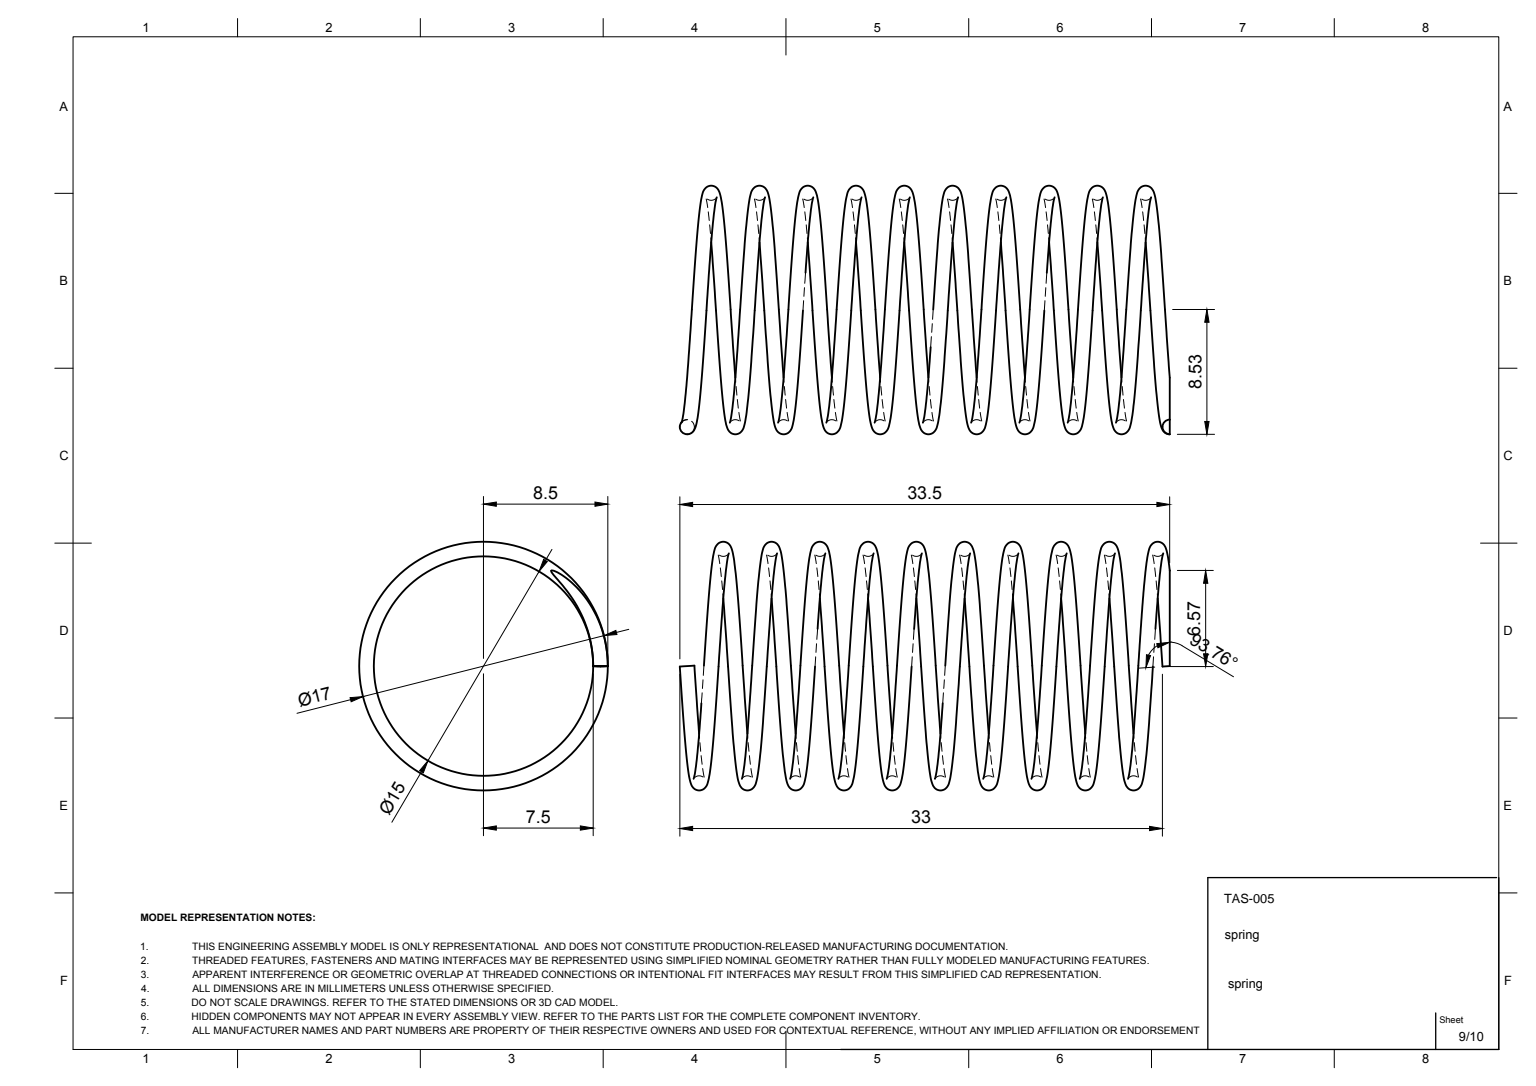
ISO-10303-21;
HEADER;
/* Generated by software containing ST-Developer
 * from STEP Tools, Inc. (www.steptools.com) 
 */

FILE_DESCRIPTION(
/* description */ ('STEP AP214'),
/* implementation_level */ '2;1');

FILE_NAME(
/* name */ 'spring.step',
/* time_stamp */ '2026-11-04T19:54:22-08:00',
/* author */ (''),
/* organization */ (''),
/* preprocessor_version */ 'ST-DEVELOPER v20.2',
/* originating_system */ 'Autodesk Translation Framework v15.17.0.0',
/* authorisation */ '');

FILE_SCHEMA (('AUTOMOTIVE_DESIGN { 1 0 10303 214 3 1 1 }'));
ENDSEC;

DATA;
#10=MECHANICAL_DESIGN_GEOMETRIC_PRESENTATION_REPRESENTATION('',(#245),#14084);
#63=(
BOUNDED_SURFACE()
B_SPLINE_SURFACE(3,2,((#9369,#9370,#9371,#9372,#9373,#9374,#9375,#9376,
#9377,#9378,#9379,#9380,#9381,#9382,#9383,#9384,#9385,#9386,#9387,#9388,
#9389,#9390,#9391,#9392,#9393,#9394,#9395,#9396,#9397,#9398,#9399,#9400,
#9401,#9402,#9403,#9404,#9405,#9406,#9407,#9408,#9409,#9410,#9411,#9412,
#9413,#9414,#9415,#9416,#9417,#9418,#9419,#9420,#9421,#9422,#9423,#9424,
#9425,#9426,#9427,#9428,#9429,#9430,#9431,#9432,#9433,#9434,#9435,#9436,
#9437,#9438,#9439,#9440,#9441,#9442,#9443,#9444,#9445,#9446,#9447,#9448,
#9449,#9450,#9451,#9452,#9453,#9454,#9455,#9456,#9457,#9458,#9459,#9460,
#9461,#9462,#9463,#9464,#9465,#9466,#9467,#9468,#9469,#9470,#9471,#9472,
#9473,#9474,#9475,#9476,#9477,#9478,#9479,#9480,#9481,#9482,#9483,#9484,
#9485,#9486,#9487,#9488,#9489,#9490,#9491,#9492,#9493,#9494,#9495,#9496,
#9497,#9498,#9499,#9500,#9501,#9502,#9503,#9504,#9505,#9506,#9507,#9508,
#9509,#9510,#9511,#9512,#9513,#9514,#9515,#9516,#9517,#9518,#9519,#9520,
#9521,#9522,#9523,#9524,#9525,#9526,#9527,#9528,#9529,#9530,#9531,#9532,
#9533,#9534,#9535,#9536,#9537,#9538,#9539,#9540,#9541,#9542,#9543,#9544,
#9545,#9546,#9547,#9548,#9549,#9550,#9551,#9552,#9553,#9554,#9555,#9556,
#9557,#9558,#9559,#9560,#9561,#9562,#9563,#9564,#9565,#9566,#9567,#9568,
#9569,#9570,#9571,#9572,#9573,#9574,#9575,#9576,#9577,#9578,#9579,#9580,
#9581,#9582,#9583,#9584,#9585,#9586,#9587,#9588,#9589,#9590,#9591,#9592,
#9593,#9594,#9595,#9596,#9597,#9598,#9599,#9600,#9601,#9602,#9603,#9604,
#9605,#9606,#9607,#9608,#9609),(#9610,#9611,#9612,#9613,#9614,#9615,#9616,
#9617,#9618,#9619,#9620,#9621,#9622,#9623,#9624,#9625,#9626,#9627,#9628,
#9629,#9630,#9631,#9632,#9633,#9634,#9635,#9636,#9637,#9638,#9639,#9640,
#9641,#9642,#9643,#9644,#9645,#9646,#9647,#9648,#9649,#9650,#9651,#9652,
#9653,#9654,#9655,#9656,#9657,#9658,#9659,#9660,#9661,#9662,#9663,#9664,
#9665,#9666,#9667,#9668,#9669,#9670,#9671,#9672,#9673,#9674,#9675,#9676,
#9677,#9678,#9679,#9680,#9681,#9682,#9683,#9684,#9685,#9686,#9687,#9688,
#9689,#9690,#9691,#9692,#9693,#9694,#9695,#9696,#9697,#9698,#9699,#9700,
#9701,#9702,#9703,#9704,#9705,#9706,#9707,#9708,#9709,#9710,#9711,#9712,
#9713,#9714,#9715,#9716,#9717,#9718,#9719,#9720,#9721,#9722,#9723,#9724,
#9725,#9726,#9727,#9728,#9729,#9730,#9731,#9732,#9733,#9734,#9735,#9736,
#9737,#9738,#9739,#9740,#9741,#9742,#9743,#9744,#9745,#9746,#9747,#9748,
#9749,#9750,#9751,#9752,#9753,#9754,#9755,#9756,#9757,#9758,#9759,#9760,
#9761,#9762,#9763,#9764,#9765,#9766,#9767,#9768,#9769,#9770,#9771,#9772,
#9773,#9774,#9775,#9776,#9777,#9778,#9779,#9780,#9781,#9782,#9783,#9784,
#9785,#9786,#9787,#9788,#9789,#9790,#9791,#9792,#9793,#9794,#9795,#9796,
#9797,#9798,#9799,#9800,#9801,#9802,#9803,#9804,#9805,#9806,#9807,#9808,
#9809,#9810,#9811,#9812,#9813,#9814,#9815,#9816,#9817,#9818,#9819,#9820,
#9821,#9822,#9823,#9824,#9825,#9826,#9827,#9828,#9829,#9830,#9831,#9832,
#9833,#9834,#9835,#9836,#9837,#9838,#9839,#9840,#9841,#9842,#9843,#9844,
#9845,#9846,#9847,#9848,#9849,#9850),(#9851,#9852,#9853,#9854,#9855,#9856,
#9857,#9858,#9859,#9860,#9861,#9862,#9863,#9864,#9865,#9866,#9867,#9868,
#9869,#9870,#9871,#9872,#9873,#9874,#9875,#9876,#9877,#9878,#9879,#9880,
#9881,#9882,#9883,#9884,#9885,#9886,#9887,#9888,#9889,#9890,#9891,#9892,
#9893,#9894,#9895,#9896,#9897,#9898,#9899,#9900,#9901,#9902,#9903,#9904,
#9905,#9906,#9907,#9908,#9909,#9910,#9911,#9912,#9913,#9914,#9915,#9916,
#9917,#9918,#9919,#9920,#9921,#9922,#9923,#9924,#9925,#9926,#9927,#9928,
#9929,#9930,#9931,#9932,#9933,#9934,#9935,#9936,#9937,#9938,#9939,#9940,
#9941,#9942,#9943,#9944,#9945,#9946,#9947,#9948,#9949,#9950,#9951,#9952,
#9953,#9954,#9955,#9956,#9957,#9958,#9959,#9960,#9961,#9962,#9963,#9964,
#9965,#9966,#9967,#9968,#9969,#9970,#9971,#9972,#9973,#9974,#9975,#9976,
#9977,#9978,#9979,#9980,#9981,#9982,#9983,#9984,#9985,#9986,#9987,#9988,
#9989,#9990,#9991,#9992,#9993,#9994,#9995,#9996,#9997,#9998,#9999,#10000,
#10001,#10002,#10003,#10004,#10005,#10006,#10007,#10008,#10009,#10010,#10011,
#10012,#10013,#10014,#10015,#10016,#10017,#10018,#10019,#10020,#10021,#10022,
#10023,#10024,#10025,#10026,#10027,#10028,#10029,#10030,#10031,#10032,#10033,
#10034,#10035,#10036,#10037,#10038,#10039,#10040,#10041,#10042,#10043,#10044,
#10045,#10046,#10047,#10048,#10049,#10050,#10051,#10052,#10053,#10054,#10055,
#10056,#10057,#10058,#10059,#10060,#10061,#10062,#10063,#10064,#10065,#10066,
#10067,#10068,#10069,#10070,#10071,#10072,#10073,#10074,#10075,#10076,#10077,
#10078,#10079,#10080,#10081,#10082,#10083,#10084,#10085,#10086,#10087,#10088,
#10089,#10090,#10091),(#10092,#10093,#10094,#10095,#10096,#10097,#10098,
#10099,#10100,#10101,#10102,#10103,#10104,#10105,#10106,#10107,#10108,#10109,
#10110,#10111,#10112,#10113,#10114,#10115,#10116,#10117,#10118,#10119,#10120,
#10121,#10122,#10123,#10124,#10125,#10126,#10127,#10128,#10129,#10130,#10131,
#10132,#10133,#10134,#10135,#10136,#10137,#10138,#10139,#10140,#10141,#10142,
#10143,#10144,#10145,#10146,#10147,#10148,#10149,#10150,#10151,#10152,#10153,
#10154,#10155,#10156,#10157,#10158,#10159,#10160,#10161,#10162,#10163,#10164,
#10165,#10166,#10167,#10168,#10169,#10170,#10171,#10172,#10173,#10174,#10175,
#10176,#10177,#10178,#10179,#10180,#10181,#10182,#10183,#10184,#10185,#10186,
#10187,#10188,#10189,#10190,#10191,#10192,#10193,#10194,#10195,#10196,#10197,
#10198,#10199,#10200,#10201,#10202,#10203,#10204,#10205,#10206,#10207,#10208,
#10209,#10210,#10211,#10212,#10213,#10214,#10215,#10216,#10217,#10218,#10219,
#10220,#10221,#10222,#10223,#10224,#10225,#10226,#10227,#10228,#10229,#10230,
#10231,#10232,#10233,#10234,#10235,#10236,#10237,#10238,#10239,#10240,#10241,
#10242,#10243,#10244,#10245,#10246,#10247,#10248,#10249,#10250,#10251,#10252,
#10253,#10254,#10255,#10256,#10257,#10258,#10259,#10260,#10261,#10262,#10263,
#10264,#10265,#10266,#10267,#10268,#10269,#10270,#10271,#10272,#10273,#10274,
#10275,#10276,#10277,#10278,#10279,#10280,#10281,#10282,#10283,#10284,#10285,
#10286,#10287,#10288,#10289,#10290,#10291,#10292,#10293,#10294,#10295,#10296,
#10297,#10298,#10299,#10300,#10301,#10302,#10303,#10304,#10305,#10306,#10307,
#10308,#10309,#10310,#10311,#10312,#10313,#10314,#10315,#10316,#10317,#10318,
#10319,#10320,#10321,#10322,#10323,#10324,#10325,#10326,#10327,#10328,#10329,
#10330,#10331,#10332),(#10333,#10334,#10335,#10336,#10337,#10338,#10339,
#10340,#10341,#10342,#10343,#10344,#10345,#10346,#10347,#10348,#10349,#10350,
#10351,#10352,#10353,#10354,#10355,#10356,#10357,#10358,#10359,#10360,#10361,
#10362,#10363,#10364,#10365,#10366,#10367,#10368,#10369,#10370,#10371,#10372,
#10373,#10374,#10375,#10376,#10377,#10378,#10379,#10380,#10381,#10382,#10383,
#10384,#10385,#10386,#10387,#10388,#10389,#10390,#10391,#10392,#10393,#10394,
#10395,#10396,#10397,#10398,#10399,#10400,#10401,#10402,#10403,#10404,#10405,
#10406,#10407,#10408,#10409,#10410,#10411,#10412,#10413,#10414,#10415,#10416,
#10417,#10418,#10419,#10420,#10421,#10422,#10423,#10424,#10425,#10426,#10427,
#10428,#10429,#10430,#10431,#10432,#10433,#10434,#10435,#10436,#10437,#10438,
#10439,#10440,#10441,#10442,#10443,#10444,#10445,#10446,#10447,#10448,#10449,
#10450,#10451,#10452,#10453,#10454,#10455,#10456,#10457,#10458,#10459,#10460,
#10461,#10462,#10463,#10464,#10465,#10466,#10467,#10468,#10469,#10470,#10471,
#10472,#10473,#10474,#10475,#10476,#10477,#10478,#10479,#10480,#10481,#10482,
#10483,#10484,#10485,#10486,#10487,#10488,#10489,#10490,#10491,#10492,#10493,
#10494,#10495,#10496,#10497,#10498,#10499,#10500,#10501,#10502,#10503,#10504,
#10505,#10506,#10507,#10508,#10509,#10510,#10511,#10512,#10513,#10514,#10515,
#10516,#10517,#10518,#10519,#10520,#10521,#10522,#10523,#10524,#10525,#10526,
#10527,#10528,#10529,#10530,#10531,#10532,#10533,#10534,#10535,#10536,#10537,
#10538,#10539,#10540,#10541,#10542,#10543,#10544,#10545,#10546,#10547,#10548,
#10549,#10550,#10551,#10552,#10553,#10554,#10555,#10556,#10557,#10558,#10559,
#10560,#10561,#10562,#10563,#10564,#10565,#10566,#10567,#10568,#10569,#10570,
#10571,#10572,#10573),(#10574,#10575,#10576,#10577,#10578,#10579,#10580,
#10581,#10582,#10583,#10584,#10585,#10586,#10587,#10588,#10589,#10590,#10591,
#10592,#10593,#10594,#10595,#10596,#10597,#10598,#10599,#10600,#10601,#10602,
#10603,#10604,#10605,#10606,#10607,#10608,#10609,#10610,#10611,#10612,#10613,
#10614,#10615,#10616,#10617,#10618,#10619,#10620,#10621,#10622,#10623,#10624,
#10625,#10626,#10627,#10628,#10629,#10630,#10631,#10632,#10633,#10634,#10635,
#10636,#10637,#10638,#10639,#10640,#10641,#10642,#10643,#10644,#10645,#10646,
#10647,#10648,#10649,#10650,#10651,#10652,#10653,#10654,#10655,#10656,#10657,
#10658,#10659,#10660,#10661,#10662,#10663,#10664,#10665,#10666,#10667,#10668,
#10669,#10670,#10671,#10672,#10673,#10674,#10675,#10676,#10677,#10678,#10679,
#10680,#10681,#10682,#10683,#10684,#10685,#10686,#10687,#10688,#10689,#10690,
#10691,#10692,#10693,#10694,#10695,#10696,#10697,#10698,#10699,#10700,#10701,
#10702,#10703,#10704,#10705,#10706,#10707,#10708,#10709,#10710,#10711,#10712,
#10713,#10714,#10715,#10716,#10717,#10718,#10719,#10720,#10721,#10722,#10723,
#10724,#10725,#10726,#10727,#10728,#10729,#10730,#10731,#10732,#10733,#10734,
#10735,#10736,#10737,#10738,#10739,#10740,#10741,#10742,#10743,#10744,#10745,
#10746,#10747,#10748,#10749,#10750,#10751,#10752,#10753,#10754,#10755,#10756,
#10757,#10758,#10759,#10760,#10761,#10762,#10763,#10764,#10765,#10766,#10767,
#10768,#10769,#10770,#10771,#10772,#10773,#10774,#10775,#10776,#10777,#10778,
#10779,#10780,#10781,#10782,#10783,#10784,#10785,#10786,#10787,#10788,#10789,
#10790,#10791,#10792,#10793,#10794,#10795,#10796,#10797,#10798,#10799,#10800,
#10801,#10802,#10803,#10804,#10805,#10806,#10807,#10808,#10809,#10810,#10811,
#10812,#10813,#10814),(#10815,#10816,#10817,#10818,#10819,#10820,#10821,
#10822,#10823,#10824,#10825,#10826,#10827,#10828,#10829,#10830,#10831,#10832,
#10833,#10834,#10835,#10836,#10837,#10838,#10839,#10840,#10841,#10842,#10843,
#10844,#10845,#10846,#10847,#10848,#10849,#10850,#10851,#10852,#10853,#10854,
#10855,#10856,#10857,#10858,#10859,#10860,#10861,#10862,#10863,#10864,#10865,
#10866,#10867,#10868,#10869,#10870,#10871,#10872,#10873,#10874,#10875,#10876,
#10877,#10878,#10879,#10880,#10881,#10882,#10883,#10884,#10885,#10886,#10887,
#10888,#10889,#10890,#10891,#10892,#10893,#10894,#10895,#10896,#10897,#10898,
#10899,#10900,#10901,#10902,#10903,#10904,#10905,#10906,#10907,#10908,#10909,
#10910,#10911,#10912,#10913,#10914,#10915,#10916,#10917,#10918,#10919,#10920,
#10921,#10922,#10923,#10924,#10925,#10926,#10927,#10928,#10929,#10930,#10931,
#10932,#10933,#10934,#10935,#10936,#10937,#10938,#10939,#10940,#10941,#10942,
#10943,#10944,#10945,#10946,#10947,#10948,#10949,#10950,#10951,#10952,#10953,
#10954,#10955,#10956,#10957,#10958,#10959,#10960,#10961,#10962,#10963,#10964,
#10965,#10966,#10967,#10968,#10969,#10970,#10971,#10972,#10973,#10974,#10975,
#10976,#10977,#10978,#10979,#10980,#10981,#10982,#10983,#10984,#10985,#10986,
#10987,#10988,#10989,#10990,#10991,#10992,#10993,#10994,#10995,#10996,#10997,
#10998,#10999,#11000,#11001,#11002,#11003,#11004,#11005,#11006,#11007,#11008,
#11009,#11010,#11011,#11012,#11013,#11014,#11015,#11016,#11017,#11018,#11019,
#11020,#11021,#11022,#11023,#11024,#11025,#11026,#11027,#11028,#11029,#11030,
#11031,#11032,#11033,#11034,#11035,#11036,#11037,#11038,#11039,#11040,#11041,
#11042,#11043,#11044,#11045,#11046,#11047,#11048,#11049,#11050,#11051,#11052,
#11053,#11054,#11055)),.UNSPECIFIED.,.T.,.F.,.F.)
B_SPLINE_SURFACE_WITH_KNOTS((4,3,4),(3,2,2,2,2,2,2,2,2,2,2,2,2,2,2,2,2,
2,2,2,2,2,2,2,2,2,2,2,2,2,2,2,2,2,2,2,2,2,2,2,2,2,2,2,2,2,2,2,2,2,2,2,2,
2,2,2,2,2,2,2,2,2,2,2,2,2,2,2,2,2,2,2,2,2,2,2,2,2,2,2,2,2,2,2,2,2,2,2,2,
2,2,2,2,2,2,2,2,2,2,2,2,2,2,2,2,2,2,2,2,2,2,2,2,2,2,2,2,2,2,2,3),(0.,0.5,
1.),(0.,0.00833333333333333,0.0166666666666667,0.025,0.0333333333333333,
0.0416666666666667,0.05,0.0583333333333333,0.0666666666666667,0.075,0.0833333333333333,
0.0916666666666667,0.1,0.108333333333333,0.116666666666667,0.125,0.133333333333333,
0.141666666666667,0.15,0.158333333333333,0.166666666666667,0.175,0.183333333333333,
0.191666666666667,0.2,0.208333333333333,0.216666666666667,0.225,0.233333333333333,
0.241666666666667,0.25,0.258333333333333,0.266666666666667,0.275,0.283333333333333,
0.291666666666667,0.3,0.308333333333333,0.316666666666667,0.325,0.333333333333333,
0.341666666666667,0.35,0.358333333333333,0.366666666666667,0.375,0.383333333333333,
0.391666666666667,0.4,0.408333333333333,0.416666666666667,0.425,0.433333333333333,
0.441666666666667,0.45,0.458333333333333,0.466666666666667,0.475,0.483333333333333,
0.491666666666667,0.5,0.508333333333333,0.516666666666667,0.525,0.533333333333333,
0.541666666666667,0.55,0.558333333333333,0.566666666666667,0.575,0.583333333333333,
0.591666666666667,0.6,0.608333333333333,0.616666666666667,0.625,0.633333333333333,
0.641666666666667,0.65,0.658333333333333,0.666666666666667,0.675,0.683333333333333,
0.691666666666667,0.7,0.708333333333333,0.716666666666667,0.725,0.733333333333333,
0.741666666666667,0.75,0.758333333333333,0.766666666666667,0.775,0.783333333333333,
0.791666666666667,0.8,0.808333333333333,0.816666666666667,0.825,0.833333333333333,
0.841666666666667,0.85,0.858333333333333,0.866666666666667,0.875,0.883333333333333,
0.891666666666667,0.9,0.908333333333333,0.916666666666667,0.925,0.933333333333333,
0.941666666666667,0.95,0.958333333333333,0.966666666666667,0.975,0.983333333333333,
0.991666666666667,1.),.UNSPECIFIED.)
GEOMETRIC_REPRESENTATION_ITEM()
RATIONAL_B_SPLINE_SURFACE(((1.,0.965925826289068,1.,0.965925826289068,1.,
0.965925826289068,1.,0.965925826289068,1.,0.965925826289068,1.,0.965925826289068,
1.,0.965925826289068,1.,0.965925826289068,1.,0.965925826289068,1.,0.965925826289068,
1.,0.965925826289068,1.,0.965925826289068,1.,0.965925826289068,1.,0.965925826289068,
1.,0.965925826289068,1.,0.965925826289068,1.,0.965925826289068,1.,0.965925826289068,
1.,0.965925826289068,1.,0.965925826289068,1.,0.965925826289068,1.,0.965925826289068,
1.,0.965925826289068,1.,0.965925826289068,1.,0.965925826289068,1.,0.965925826289068,
1.,0.965925826289068,1.,0.965925826289068,1.,0.965925826289068,1.,0.965925826289068,
1.,0.965925826289068,1.,0.965925826289068,1.,0.965925826289068,1.,0.965925826289068,
1.,0.965925826289068,1.,0.965925826289068,1.,0.965925826289068,1.,0.965925826289068,
1.,0.965925826289068,1.,0.965925826289068,1.,0.965925826289068,1.,0.965925826289068,
1.,0.965925826289068,1.,0.965925826289068,1.,0.965925826289068,1.,0.965925826289068,
1.,0.965925826289068,1.,0.965925826289068,1.,0.965925826289068,1.,0.965925826289068,
1.,0.965925826289068,1.,0.965925826289068,1.,0.965925826289068,1.,0.965925826289068,
1.,0.965925826289068,1.,0.965925826289068,1.,0.965925826289068,1.,0.965925826289068,
1.,0.965925826289068,1.,0.965925826289068,1.,0.965925826289068,1.,0.965925826289068,
1.,0.965925826289068,1.,0.965925826289068,1.,0.965925826289068,1.,0.965925826289068,
1.,0.965925826289068,1.,0.965925826289068,1.,0.965925826289068,1.,0.965925826289068,
1.,0.965925826289068,1.,0.965925826289068,1.,0.965925826289068,1.,0.965925826289068,
1.,0.965925826289068,1.,0.965925826289068,1.,0.965925826289068,1.,0.965925826289068,
1.,0.965925826289068,1.,0.965925826289068,1.,0.965925826289068,1.,0.965925826289068,
1.,0.965925826289068,1.,0.965925826289068,1.,0.965925826289068,1.,0.965925826289068,
1.,0.965925826289068,1.,0.965925826289068,1.,0.965925826289068,1.,0.965925826289068,
1.,0.965925826289068,1.,0.965925826289068,1.,0.965925826289068,1.,0.965925826289068,
1.,0.965925826289068,1.,0.965925826289068,1.,0.965925826289068,1.,0.965925826289068,
1.,0.965925826289068,1.,0.965925826289068,1.,0.965925826289068,1.,0.965925826289068,
1.,0.965925826289068,1.,0.965925826289068,1.,0.965925826289068,1.,0.965925826289068,
1.,0.965925826289068,1.,0.965925826289068,1.,0.965925826289068,1.,0.965925826289068,
1.,0.965925826289068,1.,0.965925826289068,1.,0.965925826289068,1.,0.965925826289068,
1.,0.965925826289068,1.,0.965925826289068,1.,0.965925826289068,1.,0.965925826289068,
1.,0.965925826289068,1.,0.965925826289068,1.),(0.333333333333333,0.321975275429689,
0.333333333333333,0.321975275429689,0.333333333333333,0.321975275429689,
0.333333333333333,0.321975275429689,0.333333333333333,0.321975275429689,
0.333333333333333,0.321975275429689,0.333333333333333,0.321975275429689,
0.333333333333333,0.321975275429689,0.333333333333333,0.321975275429689,
0.333333333333333,0.321975275429689,0.333333333333333,0.321975275429689,
0.333333333333333,0.321975275429689,0.333333333333333,0.321975275429689,
0.333333333333333,0.321975275429689,0.333333333333333,0.321975275429689,
0.333333333333333,0.321975275429689,0.333333333333333,0.321975275429689,
0.333333333333333,0.321975275429689,0.333333333333333,0.321975275429689,
0.333333333333333,0.321975275429689,0.333333333333333,0.321975275429689,
0.333333333333333,0.321975275429689,0.333333333333333,0.321975275429689,
0.333333333333333,0.321975275429689,0.333333333333333,0.321975275429689,
0.333333333333333,0.321975275429689,0.333333333333333,0.321975275429689,
0.333333333333333,0.321975275429689,0.333333333333333,0.321975275429689,
0.333333333333333,0.321975275429689,0.333333333333333,0.321975275429689,
0.333333333333333,0.321975275429689,0.333333333333333,0.321975275429689,
0.333333333333333,0.321975275429689,0.333333333333333,0.321975275429689,
0.333333333333333,0.321975275429689,0.333333333333333,0.321975275429689,
0.333333333333333,0.321975275429689,0.333333333333333,0.321975275429689,
0.333333333333333,0.321975275429689,0.333333333333333,0.321975275429689,
0.333333333333333,0.321975275429689,0.333333333333333,0.321975275429689,
0.333333333333333,0.321975275429689,0.333333333333333,0.321975275429689,
0.333333333333333,0.321975275429689,0.333333333333333,0.321975275429689,
0.333333333333333,0.321975275429689,0.333333333333333,0.321975275429689,
0.333333333333333,0.321975275429689,0.333333333333333,0.321975275429689,
0.333333333333333,0.321975275429689,0.333333333333333,0.321975275429689,
0.333333333333333,0.321975275429689,0.333333333333333,0.321975275429689,
0.333333333333333,0.321975275429689,0.333333333333333,0.321975275429689,
0.333333333333333,0.321975275429689,0.333333333333333,0.321975275429689,
0.333333333333333,0.321975275429689,0.333333333333333,0.321975275429689,
0.333333333333333,0.321975275429689,0.333333333333333,0.321975275429689,
0.333333333333333,0.321975275429689,0.333333333333333,0.321975275429689,
0.333333333333333,0.321975275429689,0.333333333333333,0.321975275429689,
0.333333333333333,0.321975275429689,0.333333333333333,0.321975275429689,
0.333333333333333,0.321975275429689,0.333333333333333,0.321975275429689,
0.333333333333333,0.321975275429689,0.333333333333333,0.321975275429689,
0.333333333333333,0.321975275429689,0.333333333333333,0.321975275429689,
0.333333333333333,0.321975275429689,0.333333333333333,0.321975275429689,
0.333333333333333,0.321975275429689,0.333333333333333,0.321975275429689,
0.333333333333333,0.321975275429689,0.333333333333333,0.321975275429689,
0.333333333333333,0.321975275429689,0.333333333333333,0.321975275429689,
0.333333333333333,0.321975275429689,0.333333333333333,0.321975275429689,
0.333333333333333,0.321975275429689,0.333333333333333,0.321975275429689,
0.333333333333333,0.321975275429689,0.333333333333333,0.321975275429689,
0.333333333333333,0.321975275429689,0.333333333333333,0.321975275429689,
0.333333333333333,0.321975275429689,0.333333333333333,0.321975275429689,
0.333333333333333,0.321975275429689,0.333333333333333,0.321975275429689,
0.333333333333333,0.321975275429689,0.333333333333333,0.321975275429689,
0.333333333333333,0.321975275429689,0.333333333333333,0.321975275429689,
0.333333333333333,0.321975275429689,0.333333333333333,0.321975275429689,
0.333333333333333,0.321975275429689,0.333333333333333,0.321975275429689,
0.333333333333333,0.321975275429689,0.333333333333333,0.321975275429689,
0.333333333333333,0.321975275429689,0.333333333333333,0.321975275429689,
0.333333333333333,0.321975275429689,0.333333333333333,0.321975275429689,
0.333333333333333,0.321975275429689,0.333333333333333,0.321975275429689,
0.333333333333333,0.321975275429689,0.333333333333333,0.321975275429689,
0.333333333333333,0.321975275429689,0.333333333333333,0.321975275429689,
0.333333333333333,0.321975275429689,0.333333333333333,0.321975275429689,
0.333333333333333,0.321975275429689,0.333333333333333,0.321975275429689,
0.333333333333333,0.321975275429689,0.333333333333333),(0.333333333333333,
0.321975275429689,0.333333333333333,0.321975275429689,0.333333333333333,
0.321975275429689,0.333333333333333,0.321975275429689,0.333333333333333,
0.321975275429689,0.333333333333333,0.321975275429689,0.333333333333333,
0.321975275429689,0.333333333333333,0.321975275429689,0.333333333333333,
0.321975275429689,0.333333333333333,0.321975275429689,0.333333333333333,
0.321975275429689,0.333333333333333,0.321975275429689,0.333333333333333,
0.321975275429689,0.333333333333333,0.321975275429689,0.333333333333333,
0.321975275429689,0.333333333333333,0.321975275429689,0.333333333333333,
0.321975275429689,0.333333333333333,0.321975275429689,0.333333333333333,
0.321975275429689,0.333333333333333,0.321975275429689,0.333333333333333,
0.321975275429689,0.333333333333333,0.321975275429689,0.333333333333333,
0.321975275429689,0.333333333333333,0.321975275429689,0.333333333333333,
0.321975275429689,0.333333333333333,0.321975275429689,0.333333333333333,
0.321975275429689,0.333333333333333,0.321975275429689,0.333333333333333,
0.321975275429689,0.333333333333333,0.321975275429689,0.333333333333333,
0.321975275429689,0.333333333333333,0.321975275429689,0.333333333333333,
0.321975275429689,0.333333333333333,0.321975275429689,0.333333333333333,
0.321975275429689,0.333333333333333,0.321975275429689,0.333333333333333,
0.321975275429689,0.333333333333333,0.321975275429689,0.333333333333333,
0.321975275429689,0.333333333333333,0.321975275429689,0.333333333333333,
0.321975275429689,0.333333333333333,0.321975275429689,0.333333333333333,
0.321975275429689,0.333333333333333,0.321975275429689,0.333333333333333,
0.321975275429689,0.333333333333333,0.321975275429689,0.333333333333333,
0.321975275429689,0.333333333333333,0.321975275429689,0.333333333333333,
0.321975275429689,0.333333333333333,0.321975275429689,0.333333333333333,
0.321975275429689,0.333333333333333,0.321975275429689,0.333333333333333,
0.321975275429689,0.333333333333333,0.321975275429689,0.333333333333333,
0.321975275429689,0.333333333333333,0.321975275429689,0.333333333333333,
0.321975275429689,0.333333333333333,0.321975275429689,0.333333333333333,
0.321975275429689,0.333333333333333,0.321975275429689,0.333333333333333,
0.321975275429689,0.333333333333333,0.321975275429689,0.333333333333333,
0.321975275429689,0.333333333333333,0.321975275429689,0.333333333333333,
0.321975275429689,0.333333333333333,0.321975275429689,0.333333333333333,
0.321975275429689,0.333333333333333,0.321975275429689,0.333333333333333,
0.321975275429689,0.333333333333333,0.321975275429689,0.333333333333333,
0.321975275429689,0.333333333333333,0.321975275429689,0.333333333333333,
0.321975275429689,0.333333333333333,0.321975275429689,0.333333333333333,
0.321975275429689,0.333333333333333,0.321975275429689,0.333333333333333,
0.321975275429689,0.333333333333333,0.321975275429689,0.333333333333333,
0.321975275429689,0.333333333333333,0.321975275429689,0.333333333333333,
0.321975275429689,0.333333333333333,0.321975275429689,0.333333333333333,
0.321975275429689,0.333333333333333,0.321975275429689,0.333333333333333,
0.321975275429689,0.333333333333333,0.321975275429689,0.333333333333333,
0.321975275429689,0.333333333333333,0.321975275429689,0.333333333333333,
0.321975275429689,0.333333333333333,0.321975275429689,0.333333333333333,
0.321975275429689,0.333333333333333,0.321975275429689,0.333333333333333,
0.321975275429689,0.333333333333333,0.321975275429689,0.333333333333333,
0.321975275429689,0.333333333333333,0.321975275429689,0.333333333333333,
0.321975275429689,0.333333333333333,0.321975275429689,0.333333333333333,
0.321975275429689,0.333333333333333,0.321975275429689,0.333333333333333,
0.321975275429689,0.333333333333333,0.321975275429689,0.333333333333333,
0.321975275429689,0.333333333333333,0.321975275429689,0.333333333333333,
0.321975275429689,0.333333333333333,0.321975275429689,0.333333333333333,
0.321975275429689,0.333333333333333,0.321975275429689,0.333333333333333,
0.321975275429689,0.333333333333333,0.321975275429689,0.333333333333333,
0.321975275429689,0.333333333333333,0.321975275429689,0.333333333333333,
0.321975275429689,0.333333333333333,0.321975275429689,0.333333333333333,
0.321975275429689,0.333333333333333,0.321975275429689,0.333333333333333,
0.321975275429689,0.333333333333333,0.321975275429689,0.333333333333333,
0.321975275429689,0.333333333333333,0.321975275429689,0.333333333333333),
(1.,0.965925826289068,1.,0.965925826289068,1.,0.965925826289068,1.,0.965925826289068,
1.,0.965925826289068,1.,0.965925826289068,1.,0.965925826289068,1.,0.965925826289068,
1.,0.965925826289068,1.,0.965925826289068,1.,0.965925826289068,1.,0.965925826289068,
1.,0.965925826289068,1.,0.965925826289068,1.,0.965925826289068,1.,0.965925826289068,
1.,0.965925826289068,1.,0.965925826289068,1.,0.965925826289068,1.,0.965925826289068,
1.,0.965925826289068,1.,0.965925826289068,1.,0.965925826289068,1.,0.965925826289068,
1.,0.965925826289068,1.,0.965925826289068,1.,0.965925826289068,1.,0.965925826289068,
1.,0.965925826289068,1.,0.965925826289068,1.,0.965925826289068,1.,0.965925826289068,
1.,0.965925826289068,1.,0.965925826289068,1.,0.965925826289068,1.,0.965925826289068,
1.,0.965925826289068,1.,0.965925826289068,1.,0.965925826289068,1.,0.965925826289068,
1.,0.965925826289068,1.,0.965925826289068,1.,0.965925826289068,1.,0.965925826289068,
1.,0.965925826289068,1.,0.965925826289068,1.,0.965925826289068,1.,0.965925826289068,
1.,0.965925826289068,1.,0.965925826289068,1.,0.965925826289068,1.,0.965925826289068,
1.,0.965925826289068,1.,0.965925826289068,1.,0.965925826289068,1.,0.965925826289068,
1.,0.965925826289068,1.,0.965925826289068,1.,0.965925826289068,1.,0.965925826289068,
1.,0.965925826289068,1.,0.965925826289068,1.,0.965925826289068,1.,0.965925826289068,
1.,0.965925826289068,1.,0.965925826289068,1.,0.965925826289068,1.,0.965925826289068,
1.,0.965925826289068,1.,0.965925826289068,1.,0.965925826289068,1.,0.965925826289068,
1.,0.965925826289068,1.,0.965925826289068,1.,0.965925826289068,1.,0.965925826289068,
1.,0.965925826289068,1.,0.965925826289068,1.,0.965925826289068,1.,0.965925826289068,
1.,0.965925826289068,1.,0.965925826289068,1.,0.965925826289068,1.,0.965925826289068,
1.,0.965925826289068,1.,0.965925826289068,1.,0.965925826289068,1.,0.965925826289068,
1.,0.965925826289068,1.,0.965925826289068,1.,0.965925826289068,1.,0.965925826289068,
1.,0.965925826289068,1.,0.965925826289068,1.,0.965925826289068,1.,0.965925826289068,
1.,0.965925826289068,1.,0.965925826289068,1.,0.965925826289068,1.,0.965925826289068,
1.,0.965925826289068,1.,0.965925826289068,1.,0.965925826289068,1.,0.965925826289068,
1.,0.965925826289068,1.,0.965925826289068,1.,0.965925826289068,1.,0.965925826289068,
1.,0.965925826289068,1.,0.965925826289068,1.,0.965925826289068,1.,0.965925826289068,
1.,0.965925826289068,1.,0.965925826289068,1.,0.965925826289068,1.,0.965925826289068,
1.,0.965925826289068,1.,0.965925826289068,1.,0.965925826289068,1.,0.965925826289068,
1.),(0.333333333333333,0.321975275429689,0.333333333333333,0.321975275429689,
0.333333333333333,0.321975275429689,0.333333333333333,0.321975275429689,
0.333333333333333,0.321975275429689,0.333333333333333,0.321975275429689,
0.333333333333333,0.321975275429689,0.333333333333333,0.321975275429689,
0.333333333333333,0.321975275429689,0.333333333333333,0.321975275429689,
0.333333333333333,0.321975275429689,0.333333333333333,0.321975275429689,
0.333333333333333,0.321975275429689,0.333333333333333,0.321975275429689,
0.333333333333333,0.321975275429689,0.333333333333333,0.321975275429689,
0.333333333333333,0.321975275429689,0.333333333333333,0.321975275429689,
0.333333333333333,0.321975275429689,0.333333333333333,0.321975275429689,
0.333333333333333,0.321975275429689,0.333333333333333,0.321975275429689,
0.333333333333333,0.321975275429689,0.333333333333333,0.321975275429689,
0.333333333333333,0.321975275429689,0.333333333333333,0.321975275429689,
0.333333333333333,0.321975275429689,0.333333333333333,0.321975275429689,
0.333333333333333,0.321975275429689,0.333333333333333,0.321975275429689,
0.333333333333333,0.321975275429689,0.333333333333333,0.321975275429689,
0.333333333333333,0.321975275429689,0.333333333333333,0.321975275429689,
0.333333333333333,0.321975275429689,0.333333333333333,0.321975275429689,
0.333333333333333,0.321975275429689,0.333333333333333,0.321975275429689,
0.333333333333333,0.321975275429689,0.333333333333333,0.321975275429689,
0.333333333333333,0.321975275429689,0.333333333333333,0.321975275429689,
0.333333333333333,0.321975275429689,0.333333333333333,0.321975275429689,
0.333333333333333,0.321975275429689,0.333333333333333,0.321975275429689,
0.333333333333333,0.321975275429689,0.333333333333333,0.321975275429689,
0.333333333333333,0.321975275429689,0.333333333333333,0.321975275429689,
0.333333333333333,0.321975275429689,0.333333333333333,0.321975275429689,
0.333333333333333,0.321975275429689,0.333333333333333,0.321975275429689,
0.333333333333333,0.321975275429689,0.333333333333333,0.321975275429689,
0.333333333333333,0.321975275429689,0.333333333333333,0.321975275429689,
0.333333333333333,0.321975275429689,0.333333333333333,0.321975275429689,
0.333333333333333,0.321975275429689,0.333333333333333,0.321975275429689,
0.333333333333333,0.321975275429689,0.333333333333333,0.321975275429689,
0.333333333333333,0.321975275429689,0.333333333333333,0.321975275429689,
0.333333333333333,0.321975275429689,0.333333333333333,0.321975275429689,
0.333333333333333,0.321975275429689,0.333333333333333,0.321975275429689,
0.333333333333333,0.321975275429689,0.333333333333333,0.321975275429689,
0.333333333333333,0.321975275429689,0.333333333333333,0.321975275429689,
0.333333333333333,0.321975275429689,0.333333333333333,0.321975275429689,
0.333333333333333,0.321975275429689,0.333333333333333,0.321975275429689,
0.333333333333333,0.321975275429689,0.333333333333333,0.321975275429689,
0.333333333333333,0.321975275429689,0.333333333333333,0.321975275429689,
0.333333333333333,0.321975275429689,0.333333333333333,0.321975275429689,
0.333333333333333,0.321975275429689,0.333333333333333,0.321975275429689,
0.333333333333333,0.321975275429689,0.333333333333333,0.321975275429689,
0.333333333333333,0.321975275429689,0.333333333333333,0.321975275429689,
0.333333333333333,0.321975275429689,0.333333333333333,0.321975275429689,
0.333333333333333,0.321975275429689,0.333333333333333,0.321975275429689,
0.333333333333333,0.321975275429689,0.333333333333333,0.321975275429689,
0.333333333333333,0.321975275429689,0.333333333333333,0.321975275429689,
0.333333333333333,0.321975275429689,0.333333333333333,0.321975275429689,
0.333333333333333,0.321975275429689,0.333333333333333,0.321975275429689,
0.333333333333333,0.321975275429689,0.333333333333333,0.321975275429689,
0.333333333333333,0.321975275429689,0.333333333333333,0.321975275429689,
0.333333333333333,0.321975275429689,0.333333333333333,0.321975275429689,
0.333333333333333,0.321975275429689,0.333333333333333,0.321975275429689,
0.333333333333333,0.321975275429689,0.333333333333333,0.321975275429689,
0.333333333333333,0.321975275429689,0.333333333333333,0.321975275429689,
0.333333333333333,0.321975275429689,0.333333333333333,0.321975275429689,
0.333333333333333,0.321975275429689,0.333333333333333,0.321975275429689,
0.333333333333333,0.321975275429689,0.333333333333333,0.321975275429689,
0.333333333333333),(0.333333333333333,0.321975275429689,0.333333333333333,
0.321975275429689,0.333333333333333,0.321975275429689,0.333333333333333,
0.321975275429689,0.333333333333333,0.321975275429689,0.333333333333333,
0.321975275429689,0.333333333333333,0.321975275429689,0.333333333333333,
0.321975275429689,0.333333333333333,0.321975275429689,0.333333333333333,
0.321975275429689,0.333333333333333,0.321975275429689,0.333333333333333,
0.321975275429689,0.333333333333333,0.321975275429689,0.333333333333333,
0.321975275429689,0.333333333333333,0.321975275429689,0.333333333333333,
0.321975275429689,0.333333333333333,0.321975275429689,0.333333333333333,
0.321975275429689,0.333333333333333,0.321975275429689,0.333333333333333,
0.321975275429689,0.333333333333333,0.321975275429689,0.333333333333333,
0.321975275429689,0.333333333333333,0.321975275429689,0.333333333333333,
0.321975275429689,0.333333333333333,0.321975275429689,0.333333333333333,
0.321975275429689,0.333333333333333,0.321975275429689,0.333333333333333,
0.321975275429689,0.333333333333333,0.321975275429689,0.333333333333333,
0.321975275429689,0.333333333333333,0.321975275429689,0.333333333333333,
0.321975275429689,0.333333333333333,0.321975275429689,0.333333333333333,
0.321975275429689,0.333333333333333,0.321975275429689,0.333333333333333,
0.321975275429689,0.333333333333333,0.321975275429689,0.333333333333333,
0.321975275429689,0.333333333333333,0.321975275429689,0.333333333333333,
0.321975275429689,0.333333333333333,0.321975275429689,0.333333333333333,
0.321975275429689,0.333333333333333,0.321975275429689,0.333333333333333,
0.321975275429689,0.333333333333333,0.321975275429689,0.333333333333333,
0.321975275429689,0.333333333333333,0.321975275429689,0.333333333333333,
0.321975275429689,0.333333333333333,0.321975275429689,0.333333333333333,
0.321975275429689,0.333333333333333,0.321975275429689,0.333333333333333,
0.321975275429689,0.333333333333333,0.321975275429689,0.333333333333333,
0.321975275429689,0.333333333333333,0.321975275429689,0.333333333333333,
0.321975275429689,0.333333333333333,0.321975275429689,0.333333333333333,
0.321975275429689,0.333333333333333,0.321975275429689,0.333333333333333,
0.321975275429689,0.333333333333333,0.321975275429689,0.333333333333333,
0.321975275429689,0.333333333333333,0.321975275429689,0.333333333333333,
0.321975275429689,0.333333333333333,0.321975275429689,0.333333333333333,
0.321975275429689,0.333333333333333,0.321975275429689,0.333333333333333,
0.321975275429689,0.333333333333333,0.321975275429689,0.333333333333333,
0.321975275429689,0.333333333333333,0.321975275429689,0.333333333333333,
0.321975275429689,0.333333333333333,0.321975275429689,0.333333333333333,
0.321975275429689,0.333333333333333,0.321975275429689,0.333333333333333,
0.321975275429689,0.333333333333333,0.321975275429689,0.333333333333333,
0.321975275429689,0.333333333333333,0.321975275429689,0.333333333333333,
0.321975275429689,0.333333333333333,0.321975275429689,0.333333333333333,
0.321975275429689,0.333333333333333,0.321975275429689,0.333333333333333,
0.321975275429689,0.333333333333333,0.321975275429689,0.333333333333333,
0.321975275429689,0.333333333333333,0.321975275429689,0.333333333333333,
0.321975275429689,0.333333333333333,0.321975275429689,0.333333333333333,
0.321975275429689,0.333333333333333,0.321975275429689,0.333333333333333,
0.321975275429689,0.333333333333333,0.321975275429689,0.333333333333333,
0.321975275429689,0.333333333333333,0.321975275429689,0.333333333333333,
0.321975275429689,0.333333333333333,0.321975275429689,0.333333333333333,
0.321975275429689,0.333333333333333,0.321975275429689,0.333333333333333,
0.321975275429689,0.333333333333333,0.321975275429689,0.333333333333333,
0.321975275429689,0.333333333333333,0.321975275429689,0.333333333333333,
0.321975275429689,0.333333333333333,0.321975275429689,0.333333333333333,
0.321975275429689,0.333333333333333,0.321975275429689,0.333333333333333,
0.321975275429689,0.333333333333333,0.321975275429689,0.333333333333333,
0.321975275429689,0.333333333333333,0.321975275429689,0.333333333333333,
0.321975275429689,0.333333333333333,0.321975275429689,0.333333333333333,
0.321975275429689,0.333333333333333,0.321975275429689,0.333333333333333,
0.321975275429689,0.333333333333333,0.321975275429689,0.333333333333333,
0.321975275429689,0.333333333333333,0.321975275429689,0.333333333333333,
0.321975275429689,0.333333333333333),(1.,0.965925826289068,1.,0.965925826289068,
1.,0.965925826289068,1.,0.965925826289068,1.,0.965925826289068,1.,0.965925826289068,
1.,0.965925826289068,1.,0.965925826289068,1.,0.965925826289068,1.,0.965925826289068,
1.,0.965925826289068,1.,0.965925826289068,1.,0.965925826289068,1.,0.965925826289068,
1.,0.965925826289068,1.,0.965925826289068,1.,0.965925826289068,1.,0.965925826289068,
1.,0.965925826289068,1.,0.965925826289068,1.,0.965925826289068,1.,0.965925826289068,
1.,0.965925826289068,1.,0.965925826289068,1.,0.965925826289068,1.,0.965925826289068,
1.,0.965925826289068,1.,0.965925826289068,1.,0.965925826289068,1.,0.965925826289068,
1.,0.965925826289068,1.,0.965925826289068,1.,0.965925826289068,1.,0.965925826289068,
1.,0.965925826289068,1.,0.965925826289068,1.,0.965925826289068,1.,0.965925826289068,
1.,0.965925826289068,1.,0.965925826289068,1.,0.965925826289068,1.,0.965925826289068,
1.,0.965925826289068,1.,0.965925826289068,1.,0.965925826289068,1.,0.965925826289068,
1.,0.965925826289068,1.,0.965925826289068,1.,0.965925826289068,1.,0.965925826289068,
1.,0.965925826289068,1.,0.965925826289068,1.,0.965925826289068,1.,0.965925826289068,
1.,0.965925826289068,1.,0.965925826289068,1.,0.965925826289068,1.,0.965925826289068,
1.,0.965925826289068,1.,0.965925826289068,1.,0.965925826289068,1.,0.965925826289068,
1.,0.965925826289068,1.,0.965925826289068,1.,0.965925826289068,1.,0.965925826289068,
1.,0.965925826289068,1.,0.965925826289068,1.,0.965925826289068,1.,0.965925826289068,
1.,0.965925826289068,1.,0.965925826289068,1.,0.965925826289068,1.,0.965925826289068,
1.,0.965925826289068,1.,0.965925826289068,1.,0.965925826289068,1.,0.965925826289068,
1.,0.965925826289068,1.,0.965925826289068,1.,0.965925826289068,1.,0.965925826289068,
1.,0.965925826289068,1.,0.965925826289068,1.,0.965925826289068,1.,0.965925826289068,
1.,0.965925826289068,1.,0.965925826289068,1.,0.965925826289068,1.,0.965925826289068,
1.,0.965925826289068,1.,0.965925826289068,1.,0.965925826289068,1.,0.965925826289068,
1.,0.965925826289068,1.,0.965925826289068,1.,0.965925826289068,1.,0.965925826289068,
1.,0.965925826289068,1.,0.965925826289068,1.,0.965925826289068,1.,0.965925826289068,
1.,0.965925826289068,1.,0.965925826289068,1.,0.965925826289068,1.,0.965925826289068,
1.,0.965925826289068,1.,0.965925826289068,1.,0.965925826289068,1.,0.965925826289068,
1.,0.965925826289068,1.,0.965925826289068,1.,0.965925826289068,1.,0.965925826289068,
1.,0.965925826289068,1.,0.965925826289068,1.,0.965925826289068,1.,0.965925826289068,
1.,0.965925826289068,1.,0.965925826289068,1.)))
REPRESENTATION_ITEM('')
SURFACE()
);
#64=(
BOUNDED_SURFACE()
B_SPLINE_SURFACE(3,2,((#11567,#11568,#11569,#11570,#11571,#11572,#11573,
#11574,#11575,#11576,#11577,#11578,#11579,#11580,#11581,#11582,#11583,#11584,
#11585,#11586,#11587,#11588,#11589,#11590,#11591,#11592,#11593,#11594,#11595,
#11596,#11597,#11598,#11599,#11600,#11601,#11602,#11603,#11604,#11605,#11606,
#11607,#11608,#11609,#11610,#11611,#11612,#11613,#11614,#11615,#11616,#11617,
#11618,#11619,#11620,#11621,#11622,#11623,#11624,#11625,#11626,#11627,#11628,
#11629,#11630,#11631,#11632,#11633,#11634,#11635,#11636,#11637,#11638,#11639,
#11640,#11641,#11642,#11643,#11644,#11645,#11646,#11647,#11648,#11649,#11650,
#11651,#11652,#11653,#11654,#11655,#11656,#11657,#11658,#11659,#11660,#11661,
#11662,#11663,#11664,#11665,#11666,#11667,#11668,#11669,#11670,#11671,#11672,
#11673,#11674,#11675,#11676,#11677,#11678,#11679,#11680,#11681,#11682,#11683,
#11684,#11685,#11686,#11687,#11688,#11689,#11690,#11691,#11692,#11693,#11694,
#11695,#11696,#11697,#11698,#11699,#11700,#11701,#11702,#11703,#11704,#11705,
#11706,#11707,#11708,#11709,#11710,#11711,#11712,#11713,#11714,#11715,#11716,
#11717,#11718,#11719,#11720,#11721,#11722,#11723,#11724,#11725,#11726,#11727,
#11728,#11729,#11730,#11731,#11732,#11733,#11734,#11735,#11736,#11737,#11738,
#11739,#11740,#11741,#11742,#11743,#11744,#11745,#11746,#11747,#11748,#11749,
#11750,#11751,#11752,#11753,#11754,#11755,#11756,#11757,#11758,#11759,#11760,
#11761,#11762,#11763,#11764,#11765,#11766,#11767,#11768,#11769,#11770,#11771,
#11772,#11773,#11774,#11775,#11776,#11777,#11778,#11779,#11780,#11781,#11782,
#11783,#11784,#11785,#11786,#11787,#11788,#11789,#11790,#11791,#11792,#11793,
#11794,#11795,#11796,#11797,#11798,#11799,#11800,#11801,#11802,#11803,#11804,
#11805,#11806,#11807),(#11808,#11809,#11810,#11811,#11812,#11813,#11814,
#11815,#11816,#11817,#11818,#11819,#11820,#11821,#11822,#11823,#11824,#11825,
#11826,#11827,#11828,#11829,#11830,#11831,#11832,#11833,#11834,#11835,#11836,
#11837,#11838,#11839,#11840,#11841,#11842,#11843,#11844,#11845,#11846,#11847,
#11848,#11849,#11850,#11851,#11852,#11853,#11854,#11855,#11856,#11857,#11858,
#11859,#11860,#11861,#11862,#11863,#11864,#11865,#11866,#11867,#11868,#11869,
#11870,#11871,#11872,#11873,#11874,#11875,#11876,#11877,#11878,#11879,#11880,
#11881,#11882,#11883,#11884,#11885,#11886,#11887,#11888,#11889,#11890,#11891,
#11892,#11893,#11894,#11895,#11896,#11897,#11898,#11899,#11900,#11901,#11902,
#11903,#11904,#11905,#11906,#11907,#11908,#11909,#11910,#11911,#11912,#11913,
#11914,#11915,#11916,#11917,#11918,#11919,#11920,#11921,#11922,#11923,#11924,
#11925,#11926,#11927,#11928,#11929,#11930,#11931,#11932,#11933,#11934,#11935,
#11936,#11937,#11938,#11939,#11940,#11941,#11942,#11943,#11944,#11945,#11946,
#11947,#11948,#11949,#11950,#11951,#11952,#11953,#11954,#11955,#11956,#11957,
#11958,#11959,#11960,#11961,#11962,#11963,#11964,#11965,#11966,#11967,#11968,
#11969,#11970,#11971,#11972,#11973,#11974,#11975,#11976,#11977,#11978,#11979,
#11980,#11981,#11982,#11983,#11984,#11985,#11986,#11987,#11988,#11989,#11990,
#11991,#11992,#11993,#11994,#11995,#11996,#11997,#11998,#11999,#12000,#12001,
#12002,#12003,#12004,#12005,#12006,#12007,#12008,#12009,#12010,#12011,#12012,
#12013,#12014,#12015,#12016,#12017,#12018,#12019,#12020,#12021,#12022,#12023,
#12024,#12025,#12026,#12027,#12028,#12029,#12030,#12031,#12032,#12033,#12034,
#12035,#12036,#12037,#12038,#12039,#12040,#12041,#12042,#12043,#12044,#12045,
#12046,#12047,#12048),(#12049,#12050,#12051,#12052,#12053,#12054,#12055,
#12056,#12057,#12058,#12059,#12060,#12061,#12062,#12063,#12064,#12065,#12066,
#12067,#12068,#12069,#12070,#12071,#12072,#12073,#12074,#12075,#12076,#12077,
#12078,#12079,#12080,#12081,#12082,#12083,#12084,#12085,#12086,#12087,#12088,
#12089,#12090,#12091,#12092,#12093,#12094,#12095,#12096,#12097,#12098,#12099,
#12100,#12101,#12102,#12103,#12104,#12105,#12106,#12107,#12108,#12109,#12110,
#12111,#12112,#12113,#12114,#12115,#12116,#12117,#12118,#12119,#12120,#12121,
#12122,#12123,#12124,#12125,#12126,#12127,#12128,#12129,#12130,#12131,#12132,
#12133,#12134,#12135,#12136,#12137,#12138,#12139,#12140,#12141,#12142,#12143,
#12144,#12145,#12146,#12147,#12148,#12149,#12150,#12151,#12152,#12153,#12154,
#12155,#12156,#12157,#12158,#12159,#12160,#12161,#12162,#12163,#12164,#12165,
#12166,#12167,#12168,#12169,#12170,#12171,#12172,#12173,#12174,#12175,#12176,
#12177,#12178,#12179,#12180,#12181,#12182,#12183,#12184,#12185,#12186,#12187,
#12188,#12189,#12190,#12191,#12192,#12193,#12194,#12195,#12196,#12197,#12198,
#12199,#12200,#12201,#12202,#12203,#12204,#12205,#12206,#12207,#12208,#12209,
#12210,#12211,#12212,#12213,#12214,#12215,#12216,#12217,#12218,#12219,#12220,
#12221,#12222,#12223,#12224,#12225,#12226,#12227,#12228,#12229,#12230,#12231,
#12232,#12233,#12234,#12235,#12236,#12237,#12238,#12239,#12240,#12241,#12242,
#12243,#12244,#12245,#12246,#12247,#12248,#12249,#12250,#12251,#12252,#12253,
#12254,#12255,#12256,#12257,#12258,#12259,#12260,#12261,#12262,#12263,#12264,
#12265,#12266,#12267,#12268,#12269,#12270,#12271,#12272,#12273,#12274,#12275,
#12276,#12277,#12278,#12279,#12280,#12281,#12282,#12283,#12284,#12285,#12286,
#12287,#12288,#12289),(#12290,#12291,#12292,#12293,#12294,#12295,#12296,
#12297,#12298,#12299,#12300,#12301,#12302,#12303,#12304,#12305,#12306,#12307,
#12308,#12309,#12310,#12311,#12312,#12313,#12314,#12315,#12316,#12317,#12318,
#12319,#12320,#12321,#12322,#12323,#12324,#12325,#12326,#12327,#12328,#12329,
#12330,#12331,#12332,#12333,#12334,#12335,#12336,#12337,#12338,#12339,#12340,
#12341,#12342,#12343,#12344,#12345,#12346,#12347,#12348,#12349,#12350,#12351,
#12352,#12353,#12354,#12355,#12356,#12357,#12358,#12359,#12360,#12361,#12362,
#12363,#12364,#12365,#12366,#12367,#12368,#12369,#12370,#12371,#12372,#12373,
#12374,#12375,#12376,#12377,#12378,#12379,#12380,#12381,#12382,#12383,#12384,
#12385,#12386,#12387,#12388,#12389,#12390,#12391,#12392,#12393,#12394,#12395,
#12396,#12397,#12398,#12399,#12400,#12401,#12402,#12403,#12404,#12405,#12406,
#12407,#12408,#12409,#12410,#12411,#12412,#12413,#12414,#12415,#12416,#12417,
#12418,#12419,#12420,#12421,#12422,#12423,#12424,#12425,#12426,#12427,#12428,
#12429,#12430,#12431,#12432,#12433,#12434,#12435,#12436,#12437,#12438,#12439,
#12440,#12441,#12442,#12443,#12444,#12445,#12446,#12447,#12448,#12449,#12450,
#12451,#12452,#12453,#12454,#12455,#12456,#12457,#12458,#12459,#12460,#12461,
#12462,#12463,#12464,#12465,#12466,#12467,#12468,#12469,#12470,#12471,#12472,
#12473,#12474,#12475,#12476,#12477,#12478,#12479,#12480,#12481,#12482,#12483,
#12484,#12485,#12486,#12487,#12488,#12489,#12490,#12491,#12492,#12493,#12494,
#12495,#12496,#12497,#12498,#12499,#12500,#12501,#12502,#12503,#12504,#12505,
#12506,#12507,#12508,#12509,#12510,#12511,#12512,#12513,#12514,#12515,#12516,
#12517,#12518,#12519,#12520,#12521,#12522,#12523,#12524,#12525,#12526,#12527,
#12528,#12529,#12530),(#12531,#12532,#12533,#12534,#12535,#12536,#12537,
#12538,#12539,#12540,#12541,#12542,#12543,#12544,#12545,#12546,#12547,#12548,
#12549,#12550,#12551,#12552,#12553,#12554,#12555,#12556,#12557,#12558,#12559,
#12560,#12561,#12562,#12563,#12564,#12565,#12566,#12567,#12568,#12569,#12570,
#12571,#12572,#12573,#12574,#12575,#12576,#12577,#12578,#12579,#12580,#12581,
#12582,#12583,#12584,#12585,#12586,#12587,#12588,#12589,#12590,#12591,#12592,
#12593,#12594,#12595,#12596,#12597,#12598,#12599,#12600,#12601,#12602,#12603,
#12604,#12605,#12606,#12607,#12608,#12609,#12610,#12611,#12612,#12613,#12614,
#12615,#12616,#12617,#12618,#12619,#12620,#12621,#12622,#12623,#12624,#12625,
#12626,#12627,#12628,#12629,#12630,#12631,#12632,#12633,#12634,#12635,#12636,
#12637,#12638,#12639,#12640,#12641,#12642,#12643,#12644,#12645,#12646,#12647,
#12648,#12649,#12650,#12651,#12652,#12653,#12654,#12655,#12656,#12657,#12658,
#12659,#12660,#12661,#12662,#12663,#12664,#12665,#12666,#12667,#12668,#12669,
#12670,#12671,#12672,#12673,#12674,#12675,#12676,#12677,#12678,#12679,#12680,
#12681,#12682,#12683,#12684,#12685,#12686,#12687,#12688,#12689,#12690,#12691,
#12692,#12693,#12694,#12695,#12696,#12697,#12698,#12699,#12700,#12701,#12702,
#12703,#12704,#12705,#12706,#12707,#12708,#12709,#12710,#12711,#12712,#12713,
#12714,#12715,#12716,#12717,#12718,#12719,#12720,#12721,#12722,#12723,#12724,
#12725,#12726,#12727,#12728,#12729,#12730,#12731,#12732,#12733,#12734,#12735,
#12736,#12737,#12738,#12739,#12740,#12741,#12742,#12743,#12744,#12745,#12746,
#12747,#12748,#12749,#12750,#12751,#12752,#12753,#12754,#12755,#12756,#12757,
#12758,#12759,#12760,#12761,#12762,#12763,#12764,#12765,#12766,#12767,#12768,
#12769,#12770,#12771),(#12772,#12773,#12774,#12775,#12776,#12777,#12778,
#12779,#12780,#12781,#12782,#12783,#12784,#12785,#12786,#12787,#12788,#12789,
#12790,#12791,#12792,#12793,#12794,#12795,#12796,#12797,#12798,#12799,#12800,
#12801,#12802,#12803,#12804,#12805,#12806,#12807,#12808,#12809,#12810,#12811,
#12812,#12813,#12814,#12815,#12816,#12817,#12818,#12819,#12820,#12821,#12822,
#12823,#12824,#12825,#12826,#12827,#12828,#12829,#12830,#12831,#12832,#12833,
#12834,#12835,#12836,#12837,#12838,#12839,#12840,#12841,#12842,#12843,#12844,
#12845,#12846,#12847,#12848,#12849,#12850,#12851,#12852,#12853,#12854,#12855,
#12856,#12857,#12858,#12859,#12860,#12861,#12862,#12863,#12864,#12865,#12866,
#12867,#12868,#12869,#12870,#12871,#12872,#12873,#12874,#12875,#12876,#12877,
#12878,#12879,#12880,#12881,#12882,#12883,#12884,#12885,#12886,#12887,#12888,
#12889,#12890,#12891,#12892,#12893,#12894,#12895,#12896,#12897,#12898,#12899,
#12900,#12901,#12902,#12903,#12904,#12905,#12906,#12907,#12908,#12909,#12910,
#12911,#12912,#12913,#12914,#12915,#12916,#12917,#12918,#12919,#12920,#12921,
#12922,#12923,#12924,#12925,#12926,#12927,#12928,#12929,#12930,#12931,#12932,
#12933,#12934,#12935,#12936,#12937,#12938,#12939,#12940,#12941,#12942,#12943,
#12944,#12945,#12946,#12947,#12948,#12949,#12950,#12951,#12952,#12953,#12954,
#12955,#12956,#12957,#12958,#12959,#12960,#12961,#12962,#12963,#12964,#12965,
#12966,#12967,#12968,#12969,#12970,#12971,#12972,#12973,#12974,#12975,#12976,
#12977,#12978,#12979,#12980,#12981,#12982,#12983,#12984,#12985,#12986,#12987,
#12988,#12989,#12990,#12991,#12992,#12993,#12994,#12995,#12996,#12997,#12998,
#12999,#13000,#13001,#13002,#13003,#13004,#13005,#13006,#13007,#13008,#13009,
#13010,#13011,#13012),(#13013,#13014,#13015,#13016,#13017,#13018,#13019,
#13020,#13021,#13022,#13023,#13024,#13025,#13026,#13027,#13028,#13029,#13030,
#13031,#13032,#13033,#13034,#13035,#13036,#13037,#13038,#13039,#13040,#13041,
#13042,#13043,#13044,#13045,#13046,#13047,#13048,#13049,#13050,#13051,#13052,
#13053,#13054,#13055,#13056,#13057,#13058,#13059,#13060,#13061,#13062,#13063,
#13064,#13065,#13066,#13067,#13068,#13069,#13070,#13071,#13072,#13073,#13074,
#13075,#13076,#13077,#13078,#13079,#13080,#13081,#13082,#13083,#13084,#13085,
#13086,#13087,#13088,#13089,#13090,#13091,#13092,#13093,#13094,#13095,#13096,
#13097,#13098,#13099,#13100,#13101,#13102,#13103,#13104,#13105,#13106,#13107,
#13108,#13109,#13110,#13111,#13112,#13113,#13114,#13115,#13116,#13117,#13118,
#13119,#13120,#13121,#13122,#13123,#13124,#13125,#13126,#13127,#13128,#13129,
#13130,#13131,#13132,#13133,#13134,#13135,#13136,#13137,#13138,#13139,#13140,
#13141,#13142,#13143,#13144,#13145,#13146,#13147,#13148,#13149,#13150,#13151,
#13152,#13153,#13154,#13155,#13156,#13157,#13158,#13159,#13160,#13161,#13162,
#13163,#13164,#13165,#13166,#13167,#13168,#13169,#13170,#13171,#13172,#13173,
#13174,#13175,#13176,#13177,#13178,#13179,#13180,#13181,#13182,#13183,#13184,
#13185,#13186,#13187,#13188,#13189,#13190,#13191,#13192,#13193,#13194,#13195,
#13196,#13197,#13198,#13199,#13200,#13201,#13202,#13203,#13204,#13205,#13206,
#13207,#13208,#13209,#13210,#13211,#13212,#13213,#13214,#13215,#13216,#13217,
#13218,#13219,#13220,#13221,#13222,#13223,#13224,#13225,#13226,#13227,#13228,
#13229,#13230,#13231,#13232,#13233,#13234,#13235,#13236,#13237,#13238,#13239,
#13240,#13241,#13242,#13243,#13244,#13245,#13246,#13247,#13248,#13249,#13250,
#13251,#13252,#13253)),.UNSPECIFIED.,.T.,.F.,.F.)
B_SPLINE_SURFACE_WITH_KNOTS((4,3,4),(3,2,2,2,2,2,2,2,2,2,2,2,2,2,2,2,2,
2,2,2,2,2,2,2,2,2,2,2,2,2,2,2,2,2,2,2,2,2,2,2,2,2,2,2,2,2,2,2,2,2,2,2,2,
2,2,2,2,2,2,2,2,2,2,2,2,2,2,2,2,2,2,2,2,2,2,2,2,2,2,2,2,2,2,2,2,2,2,2,2,
2,2,2,2,2,2,2,2,2,2,2,2,2,2,2,2,2,2,2,2,2,2,2,2,2,2,2,2,2,2,2,3),(0.,0.5,
1.),(0.,0.00833333333333333,0.0166666666666667,0.025,0.0333333333333333,
0.0416666666666667,0.05,0.0583333333333333,0.0666666666666667,0.075,0.0833333333333333,
0.0916666666666667,0.1,0.108333333333333,0.116666666666667,0.125,0.133333333333333,
0.141666666666667,0.15,0.158333333333333,0.166666666666667,0.175,0.183333333333333,
0.191666666666667,0.2,0.208333333333333,0.216666666666667,0.225,0.233333333333333,
0.241666666666667,0.25,0.258333333333333,0.266666666666667,0.275,0.283333333333333,
0.291666666666667,0.3,0.308333333333333,0.316666666666667,0.325,0.333333333333333,
0.341666666666667,0.35,0.358333333333333,0.366666666666667,0.375,0.383333333333333,
0.391666666666667,0.4,0.408333333333333,0.416666666666667,0.425,0.433333333333333,
0.441666666666667,0.45,0.458333333333333,0.466666666666667,0.475,0.483333333333333,
0.491666666666667,0.5,0.508333333333333,0.516666666666667,0.525,0.533333333333333,
0.541666666666667,0.55,0.558333333333333,0.566666666666667,0.575,0.583333333333333,
0.591666666666667,0.6,0.608333333333333,0.616666666666667,0.625,0.633333333333333,
0.641666666666667,0.65,0.658333333333333,0.666666666666667,0.675,0.683333333333333,
0.691666666666667,0.7,0.708333333333333,0.716666666666667,0.725,0.733333333333333,
0.741666666666667,0.75,0.758333333333333,0.766666666666667,0.775,0.783333333333333,
0.791666666666667,0.8,0.808333333333333,0.816666666666667,0.825,0.833333333333333,
0.841666666666667,0.85,0.858333333333333,0.866666666666667,0.875,0.883333333333333,
0.891666666666667,0.9,0.908333333333333,0.916666666666667,0.925,0.933333333333333,
0.941666666666667,0.95,0.958333333333333,0.966666666666667,0.975,0.983333333333333,
0.991666666666667,1.),.UNSPECIFIED.)
GEOMETRIC_REPRESENTATION_ITEM()
RATIONAL_B_SPLINE_SURFACE(((1.,0.965925826289068,1.,0.965925826289068,1.,
0.965925826289068,1.,0.965925826289068,1.,0.965925826289068,1.,0.965925826289068,
1.,0.965925826289068,1.,0.965925826289068,1.,0.965925826289068,1.,0.965925826289068,
1.,0.965925826289068,1.,0.965925826289068,1.,0.965925826289068,1.,0.965925826289068,
1.,0.965925826289068,1.,0.965925826289068,1.,0.965925826289068,1.,0.965925826289068,
1.,0.965925826289068,1.,0.965925826289068,1.,0.965925826289068,1.,0.965925826289068,
1.,0.965925826289068,1.,0.965925826289068,1.,0.965925826289068,1.,0.965925826289068,
1.,0.965925826289068,1.,0.965925826289068,1.,0.965925826289068,1.,0.965925826289068,
1.,0.965925826289068,1.,0.965925826289068,1.,0.965925826289068,1.,0.965925826289068,
1.,0.965925826289068,1.,0.965925826289068,1.,0.965925826289068,1.,0.965925826289068,
1.,0.965925826289068,1.,0.965925826289068,1.,0.965925826289068,1.,0.965925826289068,
1.,0.965925826289068,1.,0.965925826289068,1.,0.965925826289068,1.,0.965925826289068,
1.,0.965925826289068,1.,0.965925826289068,1.,0.965925826289068,1.,0.965925826289068,
1.,0.965925826289068,1.,0.965925826289068,1.,0.965925826289068,1.,0.965925826289068,
1.,0.965925826289068,1.,0.965925826289068,1.,0.965925826289068,1.,0.965925826289068,
1.,0.965925826289068,1.,0.965925826289068,1.,0.965925826289068,1.,0.965925826289068,
1.,0.965925826289068,1.,0.965925826289068,1.,0.965925826289068,1.,0.965925826289068,
1.,0.965925826289068,1.,0.965925826289068,1.,0.965925826289068,1.,0.965925826289068,
1.,0.965925826289068,1.,0.965925826289068,1.,0.965925826289068,1.,0.965925826289068,
1.,0.965925826289068,1.,0.965925826289068,1.,0.965925826289068,1.,0.965925826289068,
1.,0.965925826289068,1.,0.965925826289068,1.,0.965925826289068,1.,0.965925826289068,
1.,0.965925826289068,1.,0.965925826289068,1.,0.965925826289068,1.,0.965925826289068,
1.,0.965925826289068,1.,0.965925826289068,1.,0.965925826289068,1.,0.965925826289068,
1.,0.965925826289068,1.,0.965925826289068,1.,0.965925826289068,1.,0.965925826289068,
1.,0.965925826289068,1.,0.965925826289068,1.,0.965925826289068,1.,0.965925826289068,
1.,0.965925826289068,1.,0.965925826289068,1.,0.965925826289068,1.,0.965925826289068,
1.,0.965925826289068,1.,0.965925826289068,1.,0.965925826289068,1.,0.965925826289068,
1.,0.965925826289068,1.,0.965925826289068,1.,0.965925826289068,1.,0.965925826289068,
1.,0.965925826289068,1.,0.965925826289068,1.,0.965925826289068,1.,0.965925826289068,
1.,0.965925826289068,1.,0.965925826289068,1.,0.965925826289068,1.,0.965925826289068,
1.,0.965925826289068,1.,0.965925826289068,1.),(0.333333333333333,0.321975275429689,
0.333333333333333,0.321975275429689,0.333333333333333,0.321975275429689,
0.333333333333333,0.321975275429689,0.333333333333333,0.321975275429689,
0.333333333333333,0.321975275429689,0.333333333333333,0.321975275429689,
0.333333333333333,0.321975275429689,0.333333333333333,0.321975275429689,
0.333333333333333,0.321975275429689,0.333333333333333,0.321975275429689,
0.333333333333333,0.321975275429689,0.333333333333333,0.321975275429689,
0.333333333333333,0.321975275429689,0.333333333333333,0.321975275429689,
0.333333333333333,0.321975275429689,0.333333333333333,0.321975275429689,
0.333333333333333,0.321975275429689,0.333333333333333,0.321975275429689,
0.333333333333333,0.321975275429689,0.333333333333333,0.321975275429689,
0.333333333333333,0.321975275429689,0.333333333333333,0.321975275429689,
0.333333333333333,0.321975275429689,0.333333333333333,0.321975275429689,
0.333333333333333,0.321975275429689,0.333333333333333,0.321975275429689,
0.333333333333333,0.321975275429689,0.333333333333333,0.321975275429689,
0.333333333333333,0.321975275429689,0.333333333333333,0.321975275429689,
0.333333333333333,0.321975275429689,0.333333333333333,0.321975275429689,
0.333333333333333,0.321975275429689,0.333333333333333,0.321975275429689,
0.333333333333333,0.321975275429689,0.333333333333333,0.321975275429689,
0.333333333333333,0.321975275429689,0.333333333333333,0.321975275429689,
0.333333333333333,0.321975275429689,0.333333333333333,0.321975275429689,
0.333333333333333,0.321975275429689,0.333333333333333,0.321975275429689,
0.333333333333333,0.321975275429689,0.333333333333333,0.321975275429689,
0.333333333333333,0.321975275429689,0.333333333333333,0.321975275429689,
0.333333333333333,0.321975275429689,0.333333333333333,0.321975275429689,
0.333333333333333,0.321975275429689,0.333333333333333,0.321975275429689,
0.333333333333333,0.321975275429689,0.333333333333333,0.321975275429689,
0.333333333333333,0.321975275429689,0.333333333333333,0.321975275429689,
0.333333333333333,0.321975275429689,0.333333333333333,0.321975275429689,
0.333333333333333,0.321975275429689,0.333333333333333,0.321975275429689,
0.333333333333333,0.321975275429689,0.333333333333333,0.321975275429689,
0.333333333333333,0.321975275429689,0.333333333333333,0.321975275429689,
0.333333333333333,0.321975275429689,0.333333333333333,0.321975275429689,
0.333333333333333,0.321975275429689,0.333333333333333,0.321975275429689,
0.333333333333333,0.321975275429689,0.333333333333333,0.321975275429689,
0.333333333333333,0.321975275429689,0.333333333333333,0.321975275429689,
0.333333333333333,0.321975275429689,0.333333333333333,0.321975275429689,
0.333333333333333,0.321975275429689,0.333333333333333,0.321975275429689,
0.333333333333333,0.321975275429689,0.333333333333333,0.321975275429689,
0.333333333333333,0.321975275429689,0.333333333333333,0.321975275429689,
0.333333333333333,0.321975275429689,0.333333333333333,0.321975275429689,
0.333333333333333,0.321975275429689,0.333333333333333,0.321975275429689,
0.333333333333333,0.321975275429689,0.333333333333333,0.321975275429689,
0.333333333333333,0.321975275429689,0.333333333333333,0.321975275429689,
0.333333333333333,0.321975275429689,0.333333333333333,0.321975275429689,
0.333333333333333,0.321975275429689,0.333333333333333,0.321975275429689,
0.333333333333333,0.321975275429689,0.333333333333333,0.321975275429689,
0.333333333333333,0.321975275429689,0.333333333333333,0.321975275429689,
0.333333333333333,0.321975275429689,0.333333333333333,0.321975275429689,
0.333333333333333,0.321975275429689,0.333333333333333,0.321975275429689,
0.333333333333333,0.321975275429689,0.333333333333333,0.321975275429689,
0.333333333333333,0.321975275429689,0.333333333333333,0.321975275429689,
0.333333333333333,0.321975275429689,0.333333333333333,0.321975275429689,
0.333333333333333,0.321975275429689,0.333333333333333,0.321975275429689,
0.333333333333333,0.321975275429689,0.333333333333333,0.321975275429689,
0.333333333333333,0.321975275429689,0.333333333333333,0.321975275429689,
0.333333333333333,0.321975275429689,0.333333333333333,0.321975275429689,
0.333333333333333,0.321975275429689,0.333333333333333,0.321975275429689,
0.333333333333333,0.321975275429689,0.333333333333333,0.321975275429689,
0.333333333333333,0.321975275429689,0.333333333333333,0.321975275429689,
0.333333333333333,0.321975275429689,0.333333333333333),(0.333333333333333,
0.321975275429689,0.333333333333333,0.321975275429689,0.333333333333333,
0.321975275429689,0.333333333333333,0.321975275429689,0.333333333333333,
0.321975275429689,0.333333333333333,0.321975275429689,0.333333333333333,
0.321975275429689,0.333333333333333,0.321975275429689,0.333333333333333,
0.321975275429689,0.333333333333333,0.321975275429689,0.333333333333333,
0.321975275429689,0.333333333333333,0.321975275429689,0.333333333333333,
0.321975275429689,0.333333333333333,0.321975275429689,0.333333333333333,
0.321975275429689,0.333333333333333,0.321975275429689,0.333333333333333,
0.321975275429689,0.333333333333333,0.321975275429689,0.333333333333333,
0.321975275429689,0.333333333333333,0.321975275429689,0.333333333333333,
0.321975275429689,0.333333333333333,0.321975275429689,0.333333333333333,
0.321975275429689,0.333333333333333,0.321975275429689,0.333333333333333,
0.321975275429689,0.333333333333333,0.321975275429689,0.333333333333333,
0.321975275429689,0.333333333333333,0.321975275429689,0.333333333333333,
0.321975275429689,0.333333333333333,0.321975275429689,0.333333333333333,
0.321975275429689,0.333333333333333,0.321975275429689,0.333333333333333,
0.321975275429689,0.333333333333333,0.321975275429689,0.333333333333333,
0.321975275429689,0.333333333333333,0.321975275429689,0.333333333333333,
0.321975275429689,0.333333333333333,0.321975275429689,0.333333333333333,
0.321975275429689,0.333333333333333,0.321975275429689,0.333333333333333,
0.321975275429689,0.333333333333333,0.321975275429689,0.333333333333333,
0.321975275429689,0.333333333333333,0.321975275429689,0.333333333333333,
0.321975275429689,0.333333333333333,0.321975275429689,0.333333333333333,
0.321975275429689,0.333333333333333,0.321975275429689,0.333333333333333,
0.321975275429689,0.333333333333333,0.321975275429689,0.333333333333333,
0.321975275429689,0.333333333333333,0.321975275429689,0.333333333333333,
0.321975275429689,0.333333333333333,0.321975275429689,0.333333333333333,
0.321975275429689,0.333333333333333,0.321975275429689,0.333333333333333,
0.321975275429689,0.333333333333333,0.321975275429689,0.333333333333333,
0.321975275429689,0.333333333333333,0.321975275429689,0.333333333333333,
0.321975275429689,0.333333333333333,0.321975275429689,0.333333333333333,
0.321975275429689,0.333333333333333,0.321975275429689,0.333333333333333,
0.321975275429689,0.333333333333333,0.321975275429689,0.333333333333333,
0.321975275429689,0.333333333333333,0.321975275429689,0.333333333333333,
0.321975275429689,0.333333333333333,0.321975275429689,0.333333333333333,
0.321975275429689,0.333333333333333,0.321975275429689,0.333333333333333,
0.321975275429689,0.333333333333333,0.321975275429689,0.333333333333333,
0.321975275429689,0.333333333333333,0.321975275429689,0.333333333333333,
0.321975275429689,0.333333333333333,0.321975275429689,0.333333333333333,
0.321975275429689,0.333333333333333,0.321975275429689,0.333333333333333,
0.321975275429689,0.333333333333333,0.321975275429689,0.333333333333333,
0.321975275429689,0.333333333333333,0.321975275429689,0.333333333333333,
0.321975275429689,0.333333333333333,0.321975275429689,0.333333333333333,
0.321975275429689,0.333333333333333,0.321975275429689,0.333333333333333,
0.321975275429689,0.333333333333333,0.321975275429689,0.333333333333333,
0.321975275429689,0.333333333333333,0.321975275429689,0.333333333333333,
0.321975275429689,0.333333333333333,0.321975275429689,0.333333333333333,
0.321975275429689,0.333333333333333,0.321975275429689,0.333333333333333,
0.321975275429689,0.333333333333333,0.321975275429689,0.333333333333333,
0.321975275429689,0.333333333333333,0.321975275429689,0.333333333333333,
0.321975275429689,0.333333333333333,0.321975275429689,0.333333333333333,
0.321975275429689,0.333333333333333,0.321975275429689,0.333333333333333,
0.321975275429689,0.333333333333333,0.321975275429689,0.333333333333333,
0.321975275429689,0.333333333333333,0.321975275429689,0.333333333333333,
0.321975275429689,0.333333333333333,0.321975275429689,0.333333333333333,
0.321975275429689,0.333333333333333,0.321975275429689,0.333333333333333,
0.321975275429689,0.333333333333333,0.321975275429689,0.333333333333333,
0.321975275429689,0.333333333333333,0.321975275429689,0.333333333333333,
0.321975275429689,0.333333333333333,0.321975275429689,0.333333333333333,
0.321975275429689,0.333333333333333,0.321975275429689,0.333333333333333),
(1.,0.965925826289068,1.,0.965925826289068,1.,0.965925826289068,1.,0.965925826289068,
1.,0.965925826289068,1.,0.965925826289068,1.,0.965925826289068,1.,0.965925826289068,
1.,0.965925826289068,1.,0.965925826289068,1.,0.965925826289068,1.,0.965925826289068,
1.,0.965925826289068,1.,0.965925826289068,1.,0.965925826289068,1.,0.965925826289068,
1.,0.965925826289068,1.,0.965925826289068,1.,0.965925826289068,1.,0.965925826289068,
1.,0.965925826289068,1.,0.965925826289068,1.,0.965925826289068,1.,0.965925826289068,
1.,0.965925826289068,1.,0.965925826289068,1.,0.965925826289068,1.,0.965925826289068,
1.,0.965925826289068,1.,0.965925826289068,1.,0.965925826289068,1.,0.965925826289068,
1.,0.965925826289068,1.,0.965925826289068,1.,0.965925826289068,1.,0.965925826289068,
1.,0.965925826289068,1.,0.965925826289068,1.,0.965925826289068,1.,0.965925826289068,
1.,0.965925826289068,1.,0.965925826289068,1.,0.965925826289068,1.,0.965925826289068,
1.,0.965925826289068,1.,0.965925826289068,1.,0.965925826289068,1.,0.965925826289068,
1.,0.965925826289068,1.,0.965925826289068,1.,0.965925826289068,1.,0.965925826289068,
1.,0.965925826289068,1.,0.965925826289068,1.,0.965925826289068,1.,0.965925826289068,
1.,0.965925826289068,1.,0.965925826289068,1.,0.965925826289068,1.,0.965925826289068,
1.,0.965925826289068,1.,0.965925826289068,1.,0.965925826289068,1.,0.965925826289068,
1.,0.965925826289068,1.,0.965925826289068,1.,0.965925826289068,1.,0.965925826289068,
1.,0.965925826289068,1.,0.965925826289068,1.,0.965925826289068,1.,0.965925826289068,
1.,0.965925826289068,1.,0.965925826289068,1.,0.965925826289068,1.,0.965925826289068,
1.,0.965925826289068,1.,0.965925826289068,1.,0.965925826289068,1.,0.965925826289068,
1.,0.965925826289068,1.,0.965925826289068,1.,0.965925826289068,1.,0.965925826289068,
1.,0.965925826289068,1.,0.965925826289068,1.,0.965925826289068,1.,0.965925826289068,
1.,0.965925826289068,1.,0.965925826289068,1.,0.965925826289068,1.,0.965925826289068,
1.,0.965925826289068,1.,0.965925826289068,1.,0.965925826289068,1.,0.965925826289068,
1.,0.965925826289068,1.,0.965925826289068,1.,0.965925826289068,1.,0.965925826289068,
1.,0.965925826289068,1.,0.965925826289068,1.,0.965925826289068,1.,0.965925826289068,
1.,0.965925826289068,1.,0.965925826289068,1.,0.965925826289068,1.,0.965925826289068,
1.,0.965925826289068,1.,0.965925826289068,1.,0.965925826289068,1.,0.965925826289068,
1.,0.965925826289068,1.,0.965925826289068,1.,0.965925826289068,1.,0.965925826289068,
1.,0.965925826289068,1.,0.965925826289068,1.,0.965925826289068,1.,0.965925826289068,
1.),(0.333333333333333,0.321975275429689,0.333333333333333,0.321975275429689,
0.333333333333333,0.321975275429689,0.333333333333333,0.321975275429689,
0.333333333333333,0.321975275429689,0.333333333333333,0.321975275429689,
0.333333333333333,0.321975275429689,0.333333333333333,0.321975275429689,
0.333333333333333,0.321975275429689,0.333333333333333,0.321975275429689,
0.333333333333333,0.321975275429689,0.333333333333333,0.321975275429689,
0.333333333333333,0.321975275429689,0.333333333333333,0.321975275429689,
0.333333333333333,0.321975275429689,0.333333333333333,0.321975275429689,
0.333333333333333,0.321975275429689,0.333333333333333,0.321975275429689,
0.333333333333333,0.321975275429689,0.333333333333333,0.321975275429689,
0.333333333333333,0.321975275429689,0.333333333333333,0.321975275429689,
0.333333333333333,0.321975275429689,0.333333333333333,0.321975275429689,
0.333333333333333,0.321975275429689,0.333333333333333,0.321975275429689,
0.333333333333333,0.321975275429689,0.333333333333333,0.321975275429689,
0.333333333333333,0.321975275429689,0.333333333333333,0.321975275429689,
0.333333333333333,0.321975275429689,0.333333333333333,0.321975275429689,
0.333333333333333,0.321975275429689,0.333333333333333,0.321975275429689,
0.333333333333333,0.321975275429689,0.333333333333333,0.321975275429689,
0.333333333333333,0.321975275429689,0.333333333333333,0.321975275429689,
0.333333333333333,0.321975275429689,0.333333333333333,0.321975275429689,
0.333333333333333,0.321975275429689,0.333333333333333,0.321975275429689,
0.333333333333333,0.321975275429689,0.333333333333333,0.321975275429689,
0.333333333333333,0.321975275429689,0.333333333333333,0.321975275429689,
0.333333333333333,0.321975275429689,0.333333333333333,0.321975275429689,
0.333333333333333,0.321975275429689,0.333333333333333,0.321975275429689,
0.333333333333333,0.321975275429689,0.333333333333333,0.321975275429689,
0.333333333333333,0.321975275429689,0.333333333333333,0.321975275429689,
0.333333333333333,0.321975275429689,0.333333333333333,0.321975275429689,
0.333333333333333,0.321975275429689,0.333333333333333,0.321975275429689,
0.333333333333333,0.321975275429689,0.333333333333333,0.321975275429689,
0.333333333333333,0.321975275429689,0.333333333333333,0.321975275429689,
0.333333333333333,0.321975275429689,0.333333333333333,0.321975275429689,
0.333333333333333,0.321975275429689,0.333333333333333,0.321975275429689,
0.333333333333333,0.321975275429689,0.333333333333333,0.321975275429689,
0.333333333333333,0.321975275429689,0.333333333333333,0.321975275429689,
0.333333333333333,0.321975275429689,0.333333333333333,0.321975275429689,
0.333333333333333,0.321975275429689,0.333333333333333,0.321975275429689,
0.333333333333333,0.321975275429689,0.333333333333333,0.321975275429689,
0.333333333333333,0.321975275429689,0.333333333333333,0.321975275429689,
0.333333333333333,0.321975275429689,0.333333333333333,0.321975275429689,
0.333333333333333,0.321975275429689,0.333333333333333,0.321975275429689,
0.333333333333333,0.321975275429689,0.333333333333333,0.321975275429689,
0.333333333333333,0.321975275429689,0.333333333333333,0.321975275429689,
0.333333333333333,0.321975275429689,0.333333333333333,0.321975275429689,
0.333333333333333,0.321975275429689,0.333333333333333,0.321975275429689,
0.333333333333333,0.321975275429689,0.333333333333333,0.321975275429689,
0.333333333333333,0.321975275429689,0.333333333333333,0.321975275429689,
0.333333333333333,0.321975275429689,0.333333333333333,0.321975275429689,
0.333333333333333,0.321975275429689,0.333333333333333,0.321975275429689,
0.333333333333333,0.321975275429689,0.333333333333333,0.321975275429689,
0.333333333333333,0.321975275429689,0.333333333333333,0.321975275429689,
0.333333333333333,0.321975275429689,0.333333333333333,0.321975275429689,
0.333333333333333,0.321975275429689,0.333333333333333,0.321975275429689,
0.333333333333333,0.321975275429689,0.333333333333333,0.321975275429689,
0.333333333333333,0.321975275429689,0.333333333333333,0.321975275429689,
0.333333333333333,0.321975275429689,0.333333333333333,0.321975275429689,
0.333333333333333,0.321975275429689,0.333333333333333,0.321975275429689,
0.333333333333333,0.321975275429689,0.333333333333333,0.321975275429689,
0.333333333333333,0.321975275429689,0.333333333333333,0.321975275429689,
0.333333333333333,0.321975275429689,0.333333333333333,0.321975275429689,
0.333333333333333),(0.333333333333333,0.321975275429689,0.333333333333333,
0.321975275429689,0.333333333333333,0.321975275429689,0.333333333333333,
0.321975275429689,0.333333333333333,0.321975275429689,0.333333333333333,
0.321975275429689,0.333333333333333,0.321975275429689,0.333333333333333,
0.321975275429689,0.333333333333333,0.321975275429689,0.333333333333333,
0.321975275429689,0.333333333333333,0.321975275429689,0.333333333333333,
0.321975275429689,0.333333333333333,0.321975275429689,0.333333333333333,
0.321975275429689,0.333333333333333,0.321975275429689,0.333333333333333,
0.321975275429689,0.333333333333333,0.321975275429689,0.333333333333333,
0.321975275429689,0.333333333333333,0.321975275429689,0.333333333333333,
0.321975275429689,0.333333333333333,0.321975275429689,0.333333333333333,
0.321975275429689,0.333333333333333,0.321975275429689,0.333333333333333,
0.321975275429689,0.333333333333333,0.321975275429689,0.333333333333333,
0.321975275429689,0.333333333333333,0.321975275429689,0.333333333333333,
0.321975275429689,0.333333333333333,0.321975275429689,0.333333333333333,
0.321975275429689,0.333333333333333,0.321975275429689,0.333333333333333,
0.321975275429689,0.333333333333333,0.321975275429689,0.333333333333333,
0.321975275429689,0.333333333333333,0.321975275429689,0.333333333333333,
0.321975275429689,0.333333333333333,0.321975275429689,0.333333333333333,
0.321975275429689,0.333333333333333,0.321975275429689,0.333333333333333,
0.321975275429689,0.333333333333333,0.321975275429689,0.333333333333333,
0.321975275429689,0.333333333333333,0.321975275429689,0.333333333333333,
0.321975275429689,0.333333333333333,0.321975275429689,0.333333333333333,
0.321975275429689,0.333333333333333,0.321975275429689,0.333333333333333,
0.321975275429689,0.333333333333333,0.321975275429689,0.333333333333333,
0.321975275429689,0.333333333333333,0.321975275429689,0.333333333333333,
0.321975275429689,0.333333333333333,0.321975275429689,0.333333333333333,
0.321975275429689,0.333333333333333,0.321975275429689,0.333333333333333,
0.321975275429689,0.333333333333333,0.321975275429689,0.333333333333333,
0.321975275429689,0.333333333333333,0.321975275429689,0.333333333333333,
0.321975275429689,0.333333333333333,0.321975275429689,0.333333333333333,
0.321975275429689,0.333333333333333,0.321975275429689,0.333333333333333,
0.321975275429689,0.333333333333333,0.321975275429689,0.333333333333333,
0.321975275429689,0.333333333333333,0.321975275429689,0.333333333333333,
0.321975275429689,0.333333333333333,0.321975275429689,0.333333333333333,
0.321975275429689,0.333333333333333,0.321975275429689,0.333333333333333,
0.321975275429689,0.333333333333333,0.321975275429689,0.333333333333333,
0.321975275429689,0.333333333333333,0.321975275429689,0.333333333333333,
0.321975275429689,0.333333333333333,0.321975275429689,0.333333333333333,
0.321975275429689,0.333333333333333,0.321975275429689,0.333333333333333,
0.321975275429689,0.333333333333333,0.321975275429689,0.333333333333333,
0.321975275429689,0.333333333333333,0.321975275429689,0.333333333333333,
0.321975275429689,0.333333333333333,0.321975275429689,0.333333333333333,
0.321975275429689,0.333333333333333,0.321975275429689,0.333333333333333,
0.321975275429689,0.333333333333333,0.321975275429689,0.333333333333333,
0.321975275429689,0.333333333333333,0.321975275429689,0.333333333333333,
0.321975275429689,0.333333333333333,0.321975275429689,0.333333333333333,
0.321975275429689,0.333333333333333,0.321975275429689,0.333333333333333,
0.321975275429689,0.333333333333333,0.321975275429689,0.333333333333333,
0.321975275429689,0.333333333333333,0.321975275429689,0.333333333333333,
0.321975275429689,0.333333333333333,0.321975275429689,0.333333333333333,
0.321975275429689,0.333333333333333,0.321975275429689,0.333333333333333,
0.321975275429689,0.333333333333333,0.321975275429689,0.333333333333333,
0.321975275429689,0.333333333333333,0.321975275429689,0.333333333333333,
0.321975275429689,0.333333333333333,0.321975275429689,0.333333333333333,
0.321975275429689,0.333333333333333,0.321975275429689,0.333333333333333,
0.321975275429689,0.333333333333333,0.321975275429689,0.333333333333333,
0.321975275429689,0.333333333333333,0.321975275429689,0.333333333333333,
0.321975275429689,0.333333333333333,0.321975275429689,0.333333333333333,
0.321975275429689,0.333333333333333,0.321975275429689,0.333333333333333,
0.321975275429689,0.333333333333333),(1.,0.965925826289068,1.,0.965925826289068,
1.,0.965925826289068,1.,0.965925826289068,1.,0.965925826289068,1.,0.965925826289068,
1.,0.965925826289068,1.,0.965925826289068,1.,0.965925826289068,1.,0.965925826289068,
1.,0.965925826289068,1.,0.965925826289068,1.,0.965925826289068,1.,0.965925826289068,
1.,0.965925826289068,1.,0.965925826289068,1.,0.965925826289068,1.,0.965925826289068,
1.,0.965925826289068,1.,0.965925826289068,1.,0.965925826289068,1.,0.965925826289068,
1.,0.965925826289068,1.,0.965925826289068,1.,0.965925826289068,1.,0.965925826289068,
1.,0.965925826289068,1.,0.965925826289068,1.,0.965925826289068,1.,0.965925826289068,
1.,0.965925826289068,1.,0.965925826289068,1.,0.965925826289068,1.,0.965925826289068,
1.,0.965925826289068,1.,0.965925826289068,1.,0.965925826289068,1.,0.965925826289068,
1.,0.965925826289068,1.,0.965925826289068,1.,0.965925826289068,1.,0.965925826289068,
1.,0.965925826289068,1.,0.965925826289068,1.,0.965925826289068,1.,0.965925826289068,
1.,0.965925826289068,1.,0.965925826289068,1.,0.965925826289068,1.,0.965925826289068,
1.,0.965925826289068,1.,0.965925826289068,1.,0.965925826289068,1.,0.965925826289068,
1.,0.965925826289068,1.,0.965925826289068,1.,0.965925826289068,1.,0.965925826289068,
1.,0.965925826289068,1.,0.965925826289068,1.,0.965925826289068,1.,0.965925826289068,
1.,0.965925826289068,1.,0.965925826289068,1.,0.965925826289068,1.,0.965925826289068,
1.,0.965925826289068,1.,0.965925826289068,1.,0.965925826289068,1.,0.965925826289068,
1.,0.965925826289068,1.,0.965925826289068,1.,0.965925826289068,1.,0.965925826289068,
1.,0.965925826289068,1.,0.965925826289068,1.,0.965925826289068,1.,0.965925826289068,
1.,0.965925826289068,1.,0.965925826289068,1.,0.965925826289068,1.,0.965925826289068,
1.,0.965925826289068,1.,0.965925826289068,1.,0.965925826289068,1.,0.965925826289068,
1.,0.965925826289068,1.,0.965925826289068,1.,0.965925826289068,1.,0.965925826289068,
1.,0.965925826289068,1.,0.965925826289068,1.,0.965925826289068,1.,0.965925826289068,
1.,0.965925826289068,1.,0.965925826289068,1.,0.965925826289068,1.,0.965925826289068,
1.,0.965925826289068,1.,0.965925826289068,1.,0.965925826289068,1.,0.965925826289068,
1.,0.965925826289068,1.,0.965925826289068,1.,0.965925826289068,1.,0.965925826289068,
1.,0.965925826289068,1.,0.965925826289068,1.,0.965925826289068,1.,0.965925826289068,
1.,0.965925826289068,1.,0.965925826289068,1.,0.965925826289068,1.,0.965925826289068,
1.,0.965925826289068,1.,0.965925826289068,1.,0.965925826289068,1.,0.965925826289068,
1.,0.965925826289068,1.,0.965925826289068,1.)))
REPRESENTATION_ITEM('')
SURFACE()
);
#129=B_SPLINE_CURVE_WITH_KNOTS('',3,(#11058,#11059,#11060,#11061,#11062,
#11063,#11064,#11065,#11066,#11067,#11068,#11069,#11070,#11071,#11072,#11073,
#11074,#11075,#11076,#11077),.UNSPECIFIED.,.F.,.F.,(4,2,2,2,2,2,2,2,2,4),
(0.,0.192262276611165,0.36487527397464,0.666841526039601,0.859077160205319,
0.933919508034091,0.964372101203401,0.976575083217201,0.981856483830181,
0.986854022611611),.UNSPECIFIED.);
#130=B_SPLINE_CURVE_WITH_KNOTS('',3,(#13254,#13255,#13256,#13257,#13258,
#13259,#13260,#13261,#13262,#13263,#13264,#13265,#13266,#13267,#13268,#13269,
#13270,#13271,#13272,#13273),.UNSPECIFIED.,.F.,.F.,(4,2,2,2,2,2,2,2,2,4),
(1.00001729274522E-6,0.000806658582909784,0.00167003986182473,0.00372333846850495,
0.00950633881409832,0.0259676755535791,0.0679386431653802,0.119530949671773,
0.1558134434742,0.196417574801726),.UNSPECIFIED.);
#207=(
BOUNDED_CURVE()
B_SPLINE_CURVE(2,(#11079,#11080,#11081,#11082,#11083,#11084,#11085,#11086,
#11087,#11088,#11089,#11090,#11091,#11092,#11093,#11094,#11095,#11096,#11097,
#11098,#11099,#11100,#11101,#11102,#11103,#11104,#11105,#11106,#11107,#11108,
#11109,#11110,#11111,#11112,#11113,#11114,#11115,#11116,#11117,#11118,#11119,
#11120,#11121,#11122,#11123,#11124,#11125,#11126,#11127,#11128,#11129,#11130,
#11131,#11132,#11133,#11134,#11135,#11136,#11137,#11138,#11139,#11140,#11141,
#11142,#11143,#11144,#11145,#11146,#11147,#11148,#11149,#11150,#11151,#11152,
#11153,#11154,#11155,#11156,#11157,#11158,#11159,#11160,#11161,#11162,#11163,
#11164,#11165,#11166,#11167,#11168,#11169,#11170,#11171,#11172,#11173,#11174,
#11175,#11176,#11177,#11178,#11179,#11180,#11181,#11182,#11183,#11184,#11185,
#11186,#11187,#11188,#11189,#11190,#11191,#11192,#11193,#11194,#11195,#11196,
#11197,#11198,#11199,#11200,#11201,#11202,#11203,#11204,#11205,#11206,#11207,
#11208,#11209,#11210,#11211,#11212,#11213,#11214,#11215,#11216,#11217,#11218,
#11219,#11220,#11221,#11222,#11223,#11224,#11225,#11226,#11227,#11228,#11229,
#11230,#11231,#11232,#11233,#11234,#11235,#11236,#11237,#11238,#11239,#11240,
#11241,#11242,#11243,#11244,#11245,#11246,#11247,#11248,#11249,#11250,#11251,
#11252,#11253,#11254,#11255,#11256,#11257,#11258,#11259,#11260,#11261,#11262,
#11263,#11264,#11265,#11266,#11267,#11268,#11269,#11270,#11271,#11272,#11273,
#11274,#11275,#11276,#11277,#11278,#11279,#11280,#11281,#11282,#11283,#11284,
#11285,#11286,#11287,#11288,#11289,#11290,#11291,#11292,#11293,#11294,#11295,
#11296,#11297,#11298,#11299,#11300,#11301,#11302,#11303,#11304,#11305,#11306,
#11307,#11308,#11309,#11310,#11311,#11312,#11313,#11314,#11315,#11316,#11317),
 .UNSPECIFIED.,.F.,.F.)
B_SPLINE_CURVE_WITH_KNOTS((3,2,2,2,2,2,2,2,2,2,2,2,2,2,2,2,2,2,2,2,2,2,
2,2,2,2,2,2,2,2,2,2,2,2,2,2,2,2,2,2,2,2,2,2,2,2,2,2,2,2,2,2,2,2,2,2,2,2,
2,2,2,2,2,2,2,2,2,2,2,2,2,2,2,2,2,2,2,2,2,2,2,2,2,2,2,2,2,2,2,2,2,2,2,2,
2,2,2,2,2,2,2,2,2,2,2,2,2,2,2,2,2,2,2,2,2,2,2,2,2,3),(0.0150916102575603,
0.0166666666666667,0.025,0.0333333333333333,0.0416666666666667,0.05,0.0583333333333333,
0.0666666666666667,0.075,0.0833333333333333,0.0916666666666667,0.1,0.108333333333333,
0.116666666666667,0.125,0.133333333333333,0.141666666666667,0.15,0.158333333333333,
0.166666666666667,0.175,0.183333333333333,0.191666666666667,0.2,0.208333333333333,
0.216666666666667,0.225,0.233333333333333,0.241666666666667,0.25,0.258333333333333,
0.266666666666667,0.275,0.283333333333333,0.291666666666667,0.3,0.308333333333333,
0.316666666666667,0.325,0.333333333333333,0.341666666666667,0.35,0.358333333333333,
0.366666666666667,0.375,0.383333333333333,0.391666666666667,0.4,0.408333333333333,
0.416666666666667,0.425,0.433333333333333,0.441666666666667,0.45,0.458333333333333,
0.466666666666667,0.475,0.483333333333333,0.491666666666667,0.5,0.508333333333333,
0.516666666666667,0.525,0.533333333333333,0.541666666666667,0.55,0.558333333333333,
0.566666666666667,0.575,0.583333333333333,0.591666666666667,0.6,0.608333333333333,
0.616666666666667,0.625,0.633333333333333,0.641666666666667,0.65,0.658333333333333,
0.666666666666667,0.675,0.683333333333333,0.691666666666667,0.7,0.708333333333333,
0.716666666666667,0.725,0.733333333333333,0.741666666666667,0.75,0.758333333333333,
0.766666666666667,0.775,0.783333333333333,0.791666666666667,0.8,0.808333333333333,
0.816666666666667,0.825,0.833333333333333,0.841666666666667,0.85,0.858333333333333,
0.866666666666667,0.875,0.883333333333333,0.891666666666667,0.9,0.908333333333333,
0.916666666666667,0.925,0.933333333333333,0.941666666666667,0.95,0.958333333333333,
0.966666666666667,0.975,0.983333333333333,0.991666666666667,1.),
 .UNSPECIFIED.)
CURVE()
GEOMETRIC_REPRESENTATION_ITEM()
RATIONAL_B_SPLINE_CURVE((0.989554002528501,0.993559750517391,1.,0.965925826289068,
1.,0.965925826289068,1.,0.965925826289068,1.,0.965925826289068,1.,0.965925826289068,
1.,0.965925826289068,1.,0.965925826289068,1.,0.965925826289068,1.,0.965925826289068,
1.,0.965925826289068,1.,0.965925826289068,1.,0.965925826289068,1.,0.965925826289068,
1.,0.965925826289068,1.,0.965925826289068,1.,0.965925826289068,1.,0.965925826289068,
1.,0.965925826289068,1.,0.965925826289068,1.,0.965925826289068,1.,0.965925826289068,
1.,0.965925826289068,1.,0.965925826289068,1.,0.965925826289068,1.,0.965925826289068,
1.,0.965925826289068,1.,0.965925826289068,1.,0.965925826289068,1.,0.965925826289068,
1.,0.965925826289068,1.,0.965925826289068,1.,0.965925826289068,1.,0.965925826289068,
1.,0.965925826289068,1.,0.965925826289068,1.,0.965925826289068,1.,0.965925826289068,
1.,0.965925826289068,1.,0.965925826289068,1.,0.965925826289068,1.,0.965925826289068,
1.,0.965925826289068,1.,0.965925826289068,1.,0.965925826289068,1.,0.965925826289068,
1.,0.965925826289068,1.,0.965925826289068,1.,0.965925826289068,1.,0.965925826289068,
1.,0.965925826289068,1.,0.965925826289068,1.,0.965925826289068,1.,0.965925826289068,
1.,0.965925826289068,1.,0.965925826289068,1.,0.965925826289068,1.,0.965925826289068,
1.,0.965925826289068,1.,0.965925826289068,1.,0.965925826289068,1.,0.965925826289068,
1.,0.965925826289068,1.,0.965925826289068,1.,0.965925826289068,1.,0.965925826289068,
1.,0.965925826289068,1.,0.965925826289068,1.,0.965925826289068,1.,0.965925826289068,
1.,0.965925826289068,1.,0.965925826289068,1.,0.965925826289068,1.,0.965925826289068,
1.,0.965925826289068,1.,0.965925826289068,1.,0.965925826289068,1.,0.965925826289068,
1.,0.965925826289068,1.,0.965925826289068,1.,0.965925826289068,1.,0.965925826289068,
1.,0.965925826289068,1.,0.965925826289068,1.,0.965925826289068,1.,0.965925826289068,
1.,0.965925826289068,1.,0.965925826289068,1.,0.965925826289068,1.,0.965925826289068,
1.,0.965925826289068,1.,0.965925826289068,1.,0.965925826289068,1.,0.965925826289068,
1.,0.965925826289068,1.,0.965925826289068,1.,0.965925826289068,1.,0.965925826289068,
1.,0.965925826289068,1.,0.965925826289068,1.,0.965925826289068,1.,0.965925826289068,
1.,0.965925826289068,1.,0.965925826289068,1.,0.965925826289068,1.,0.965925826289068,
1.,0.965925826289068,1.,0.965925826289068,1.,0.965925826289068,1.,0.965925826289068,
1.,0.965925826289068,1.,0.965925826289068,1.,0.965925826289068,1.,0.965925826289068,
1.,0.965925826289068,1.,0.965925826289068,1.,0.965925826289068,1.,0.965925826289068,
1.,0.965925826289068,1.))
REPRESENTATION_ITEM('')
);
#208=(
BOUNDED_CURVE()
B_SPLINE_CURVE(2,(#11321,#11322,#11323,#11324,#11325,#11326,#11327,#11328,
#11329,#11330,#11331,#11332,#11333,#11334,#11335,#11336,#11337,#11338,#11339,
#11340,#11341,#11342,#11343,#11344,#11345,#11346,#11347,#11348,#11349,#11350,
#11351,#11352,#11353,#11354,#11355,#11356,#11357,#11358,#11359,#11360,#11361,
#11362,#11363,#11364,#11365,#11366,#11367,#11368,#11369,#11370,#11371,#11372,
#11373,#11374,#11375,#11376,#11377,#11378,#11379,#11380,#11381,#11382,#11383,
#11384,#11385,#11386,#11387,#11388,#11389,#11390,#11391,#11392,#11393,#11394,
#11395,#11396,#11397,#11398,#11399,#11400,#11401,#11402,#11403,#11404,#11405,
#11406,#11407,#11408,#11409,#11410,#11411,#11412,#11413,#11414,#11415,#11416,
#11417,#11418,#11419,#11420,#11421,#11422,#11423,#11424,#11425,#11426,#11427,
#11428,#11429,#11430,#11431,#11432,#11433,#11434,#11435,#11436,#11437,#11438,
#11439,#11440,#11441,#11442,#11443,#11444,#11445,#11446,#11447,#11448,#11449,
#11450,#11451,#11452,#11453,#11454,#11455,#11456,#11457,#11458,#11459,#11460,
#11461,#11462,#11463,#11464,#11465,#11466,#11467,#11468,#11469,#11470,#11471,
#11472,#11473,#11474,#11475,#11476,#11477,#11478,#11479,#11480,#11481,#11482,
#11483,#11484,#11485,#11486,#11487,#11488,#11489,#11490,#11491,#11492,#11493,
#11494,#11495,#11496,#11497,#11498,#11499,#11500,#11501,#11502,#11503,#11504,
#11505,#11506,#11507,#11508,#11509,#11510,#11511,#11512,#11513,#11514,#11515,
#11516,#11517,#11518,#11519,#11520,#11521,#11522,#11523,#11524,#11525,#11526,
#11527,#11528,#11529,#11530,#11531,#11532,#11533,#11534,#11535,#11536,#11537,
#11538,#11539,#11540,#11541,#11542,#11543,#11544,#11545,#11546,#11547,#11548,
#11549,#11550,#11551,#11552,#11553,#11554,#11555,#11556,#11557,#11558,#11559,
#11560,#11561),.UNSPECIFIED.,.F.,.F.)
B_SPLINE_CURVE_WITH_KNOTS((3,2,2,2,2,2,2,2,2,2,2,2,2,2,2,2,2,2,2,2,2,2,
2,2,2,2,2,2,2,2,2,2,2,2,2,2,2,2,2,2,2,2,2,2,2,2,2,2,2,2,2,2,2,2,2,2,2,2,
2,2,2,2,2,2,2,2,2,2,2,2,2,2,2,2,2,2,2,2,2,2,2,2,2,2,2,2,2,2,2,2,2,2,2,2,
2,2,2,2,2,2,2,2,2,2,2,2,2,2,2,2,2,2,2,2,2,2,2,2,2,2,3),(0.,0.00833333333333333,
0.0166666666666667,0.025,0.0333333333333333,0.0416666666666667,0.05,0.0583333333333333,
0.0666666666666667,0.075,0.0833333333333333,0.0916666666666667,0.1,0.108333333333333,
0.116666666666667,0.125,0.133333333333333,0.141666666666667,0.15,0.158333333333333,
0.166666666666667,0.175,0.183333333333333,0.191666666666667,0.2,0.208333333333333,
0.216666666666667,0.225,0.233333333333333,0.241666666666667,0.25,0.258333333333333,
0.266666666666667,0.275,0.283333333333333,0.291666666666667,0.3,0.308333333333333,
0.316666666666667,0.325,0.333333333333333,0.341666666666667,0.35,0.358333333333333,
0.366666666666667,0.375,0.383333333333333,0.391666666666667,0.4,0.408333333333333,
0.416666666666667,0.425,0.433333333333333,0.441666666666667,0.45,0.458333333333333,
0.466666666666667,0.475,0.483333333333333,0.491666666666667,0.5,0.508333333333333,
0.516666666666667,0.525,0.533333333333333,0.541666666666667,0.55,0.558333333333333,
0.566666666666667,0.575,0.583333333333333,0.591666666666667,0.6,0.608333333333333,
0.616666666666667,0.625,0.633333333333333,0.641666666666667,0.65,0.658333333333333,
0.666666666666667,0.675,0.683333333333333,0.691666666666667,0.7,0.708333333333333,
0.716666666666667,0.725,0.733333333333333,0.741666666666667,0.75,0.758333333333333,
0.766666666666667,0.775,0.783333333333333,0.791666666666667,0.8,0.808333333333333,
0.816666666666667,0.825,0.833333333333333,0.841666666666667,0.85,0.858333333333333,
0.866666666666667,0.875,0.883333333333333,0.891666666666667,0.9,0.908333333333333,
0.916666666666667,0.925,0.933333333333333,0.941666666666667,0.95,0.958333333333333,
0.966666666666667,0.975,0.983333333333333,0.991666666666667,1.),
 .UNSPECIFIED.)
CURVE()
GEOMETRIC_REPRESENTATION_ITEM()
RATIONAL_B_SPLINE_CURVE((1.,0.965925826289068,1.,0.965925826289068,1.,0.965925826289068,
1.,0.965925826289068,1.,0.965925826289068,1.,0.965925826289068,1.,0.965925826289068,
1.,0.965925826289068,1.,0.965925826289068,1.,0.965925826289068,1.,0.965925826289068,
1.,0.965925826289068,1.,0.965925826289068,1.,0.965925826289068,1.,0.965925826289068,
1.,0.965925826289068,1.,0.965925826289068,1.,0.965925826289068,1.,0.965925826289068,
1.,0.965925826289068,1.,0.965925826289068,1.,0.965925826289068,1.,0.965925826289068,
1.,0.965925826289068,1.,0.965925826289068,1.,0.965925826289068,1.,0.965925826289068,
1.,0.965925826289068,1.,0.965925826289068,1.,0.965925826289068,1.,0.965925826289068,
1.,0.965925826289068,1.,0.965925826289068,1.,0.965925826289068,1.,0.965925826289068,
1.,0.965925826289068,1.,0.965925826289068,1.,0.965925826289068,1.,0.965925826289068,
1.,0.965925826289068,1.,0.965925826289068,1.,0.965925826289068,1.,0.965925826289068,
1.,0.965925826289068,1.,0.965925826289068,1.,0.965925826289068,1.,0.965925826289068,
1.,0.965925826289068,1.,0.965925826289068,1.,0.965925826289068,1.,0.965925826289068,
1.,0.965925826289068,1.,0.965925826289068,1.,0.965925826289068,1.,0.965925826289068,
1.,0.965925826289068,1.,0.965925826289068,1.,0.965925826289068,1.,0.965925826289068,
1.,0.965925826289068,1.,0.965925826289068,1.,0.965925826289068,1.,0.965925826289068,
1.,0.965925826289068,1.,0.965925826289068,1.,0.965925826289068,1.,0.965925826289068,
1.,0.965925826289068,1.,0.965925826289068,1.,0.965925826289068,1.,0.965925826289068,
1.,0.965925826289068,1.,0.965925826289068,1.,0.965925826289068,1.,0.965925826289068,
1.,0.965925826289068,1.,0.965925826289068,1.,0.965925826289068,1.,0.965925826289068,
1.,0.965925826289068,1.,0.965925826289068,1.,0.965925826289068,1.,0.965925826289068,
1.,0.965925826289068,1.,0.965925826289068,1.,0.965925826289068,1.,0.965925826289068,
1.,0.965925826289068,1.,0.965925826289068,1.,0.965925826289068,1.,0.965925826289068,
1.,0.965925826289068,1.,0.965925826289068,1.,0.965925826289068,1.,0.965925826289068,
1.,0.965925826289068,1.,0.965925826289068,1.,0.965925826289068,1.,0.965925826289068,
1.,0.965925826289068,1.,0.965925826289068,1.,0.965925826289068,1.,0.965925826289068,
1.,0.965925826289068,1.,0.965925826289068,1.,0.965925826289068,1.,0.965925826289068,
1.,0.965925826289068,1.,0.965925826289068,1.,0.965925826289068,1.,0.965925826289068,
1.,0.965925826289068,1.,0.965925826289068,1.,0.965925826289068,1.,0.965925826289068,
1.,0.965925826289068,1.,0.965925826289068,1.,0.965925826289068,1.,0.965925826289068,
1.,0.965925826289068,1.))
REPRESENTATION_ITEM('')
);
#227=SHAPE_REPRESENTATION_RELATIONSHIP('SRR','None',#14126,#236);
#236=ADVANCED_BREP_SHAPE_REPRESENTATION('',(#254),#14081);
#245=STYLED_ITEM('',(#14176),#254);
#254=MANIFOLD_SOLID_BREP('Body1',#3471);
#350=PLANE('',#3797);
#351=PLANE('',#3800);
#352=PLANE('',#3801);
#517=FACE_OUTER_BOUND('',#731,.T.);
#518=FACE_OUTER_BOUND('',#732,.T.);
#519=FACE_OUTER_BOUND('',#733,.T.);
#520=FACE_OUTER_BOUND('',#734,.T.);
#521=FACE_OUTER_BOUND('',#735,.T.);
#731=EDGE_LOOP('',(#3031,#3032,#3033,#3034,#3035));
#732=EDGE_LOOP('',(#3036,#3037,#3038));
#733=EDGE_LOOP('',(#3039,#3040,#3041,#3042,#3043));
#734=EDGE_LOOP('',(#3044,#3045));
#735=EDGE_LOOP('',(#3046,#3047,#3048));
#1015=LINE('',#11566,#1272);
#1272=VECTOR('',#4556,1000.);
#1350=CIRCLE('',#3795,0.499999999999983);
#1351=CIRCLE('',#3796,0.499999999999983);
#1352=CIRCLE('',#3798,0.499999999999983);
#1353=CIRCLE('',#3799,0.499999999999983);
#1654=VERTEX_POINT('',#11056);
#1655=VERTEX_POINT('',#11057);
#1656=VERTEX_POINT('',#11078);
#1657=VERTEX_POINT('',#11318);
#1658=VERTEX_POINT('',#11320);
#1659=VERTEX_POINT('',#11564);
#2119=EDGE_CURVE('',#1654,#1655,#129,.T.);
#2120=EDGE_CURVE('',#1655,#1656,#207,.T.);
#2121=EDGE_CURVE('',#1656,#1657,#1350,.T.);
#2122=EDGE_CURVE('',#1658,#1657,#208,.T.);
#2123=EDGE_CURVE('',#1658,#1654,#1351,.T.);
#2124=EDGE_CURVE('',#1659,#1658,#1352,.T.);
#2125=EDGE_CURVE('',#1659,#1654,#1015,.T.);
#2126=EDGE_CURVE('',#1655,#1659,#130,.T.);
#2127=EDGE_CURVE('',#1657,#1656,#1353,.T.);
#3031=ORIENTED_EDGE('',*,*,#2119,.T.);
#3032=ORIENTED_EDGE('',*,*,#2120,.T.);
#3033=ORIENTED_EDGE('',*,*,#2121,.T.);
#3034=ORIENTED_EDGE('',*,*,#2122,.F.);
#3035=ORIENTED_EDGE('',*,*,#2123,.T.);
#3036=ORIENTED_EDGE('',*,*,#2124,.F.);
#3037=ORIENTED_EDGE('',*,*,#2125,.T.);
#3038=ORIENTED_EDGE('',*,*,#2123,.F.);
#3039=ORIENTED_EDGE('',*,*,#2120,.F.);
#3040=ORIENTED_EDGE('',*,*,#2126,.T.);
#3041=ORIENTED_EDGE('',*,*,#2124,.T.);
#3042=ORIENTED_EDGE('',*,*,#2122,.T.);
#3043=ORIENTED_EDGE('',*,*,#2127,.T.);
#3044=ORIENTED_EDGE('',*,*,#2127,.F.);
#3045=ORIENTED_EDGE('',*,*,#2121,.F.);
#3046=ORIENTED_EDGE('',*,*,#2119,.F.);
#3047=ORIENTED_EDGE('',*,*,#2125,.F.);
#3048=ORIENTED_EDGE('',*,*,#2126,.F.);
#3427=ADVANCED_FACE('',(#517),#63,.T.);
#3428=ADVANCED_FACE('',(#518),#350,.T.);
#3429=ADVANCED_FACE('',(#519),#64,.T.);
#3430=ADVANCED_FACE('',(#520),#351,.F.);
#3431=ADVANCED_FACE('',(#521),#352,.T.);
#3471=CLOSED_SHELL('',(#3427,#3428,#3429,#3430,#3431));
#3794=AXIS2_PLACEMENT_3D('',#9368,#4546,#4547);
#3795=AXIS2_PLACEMENT_3D('',#11319,#4548,#4549);
#3796=AXIS2_PLACEMENT_3D('',#11562,#4550,#4551);
#3797=AXIS2_PLACEMENT_3D('',#11563,#4552,#4553);
#3798=AXIS2_PLACEMENT_3D('',#11565,#4554,#4555);
#3799=AXIS2_PLACEMENT_3D('',#13274,#4557,#4558);
#3800=AXIS2_PLACEMENT_3D('',#13275,#4559,#4560);
#3801=AXIS2_PLACEMENT_3D('',#13276,#4561,#4562);
#4546=DIRECTION('axis',(0.,0.,1.));
#4547=DIRECTION('refdir',(1.,0.,0.));
#4548=DIRECTION('center_axis',(9.93970987904536E-15,-0.0655103873942315,
0.99785188737781));
#4549=DIRECTION('ref_axis',(-2.5496135091776E-31,0.99785188737781,0.0655103873942315));
#4550=DIRECTION('center_axis',(-9.93970987904536E-15,0.0655103873942315,
-0.99785188737781));
#4551=DIRECTION('ref_axis',(-2.5496135091776E-31,0.99785188737781,0.0655103873942315));
#4552=DIRECTION('center_axis',(9.93970987904537E-15,-0.0655103873942315,
0.99785188737781));
#4553=DIRECTION('ref_axis',(-1.56056201915558E-32,-0.99785188737781,-0.0655103873942315));
#4554=DIRECTION('center_axis',(-9.93970987904536E-15,0.0655103873942315,
-0.99785188737781));
#4555=DIRECTION('ref_axis',(-2.5496135091776E-31,0.99785188737781,0.0655103873942315));
#4556=DIRECTION('',(1.,0.,-9.96110745971056E-15));
#4557=DIRECTION('center_axis',(9.93970987904536E-15,-0.0655103873942315,
0.99785188737781));
#4558=DIRECTION('ref_axis',(-2.5496135091776E-31,0.99785188737781,0.0655103873942315));
#4559=DIRECTION('center_axis',(9.93970987904537E-15,-0.0655103873942315,
0.99785188737781));
#4560=DIRECTION('ref_axis',(-1.56056201915558E-32,-0.99785188737781,-0.0655103873942315));
#4561=DIRECTION('center_axis',(0.,-1.,0.));
#4562=DIRECTION('ref_axis',(-1.,0.,0.));
#9368=CARTESIAN_POINT('',(0.,0.,0.));
#9369=CARTESIAN_POINT('Ctrl Pts',(-8.,285.498925943689,0.0327551936971979));
#9370=CARTESIAN_POINT('Ctrl Pts',(-8.00877672769909,285.636425943689,-2.11083834575178));
#9371=CARTESIAN_POINT('Ctrl Pts',(-6.94458082712411,285.773925943689,-3.97163317015235));
#9372=CARTESIAN_POINT('Ctrl Pts',(-5.88038492654913,285.911425943689,-5.83242799455291));
#9373=CARTESIAN_POINT('Ctrl Pts',(-4.02836682984766,286.048925943689,-6.91182563342691));
#9374=CARTESIAN_POINT('Ctrl Pts',(-2.17634873314618,286.186425943689,-7.99122327230091));
#9375=CARTESIAN_POINT('Ctrl Pts',(-0.0327551936971984,286.323925943689,
-8.));
#9376=CARTESIAN_POINT('Ctrl Pts',(2.11083834575178,286.461425943689,-8.00877672769909));
#9377=CARTESIAN_POINT('Ctrl Pts',(3.97163317015235,286.598925943689,-6.94458082712411));
#9378=CARTESIAN_POINT('Ctrl Pts',(5.83242799455291,286.736425943689,-5.88038492654913));
#9379=CARTESIAN_POINT('Ctrl Pts',(6.91182563342691,286.873925943689,-4.02836682984766));
#9380=CARTESIAN_POINT('Ctrl Pts',(7.99122327230091,287.011425943689,-2.17634873314618));
#9381=CARTESIAN_POINT('Ctrl Pts',(8.,287.148925943689,-0.0327551936971989));
#9382=CARTESIAN_POINT('Ctrl Pts',(8.00877672769909,287.286425943689,2.11083834575178));
#9383=CARTESIAN_POINT('Ctrl Pts',(6.94458082712411,287.423925943689,3.97163317015235));
#9384=CARTESIAN_POINT('Ctrl Pts',(5.88038492654913,287.561425943689,5.83242799455291));
#9385=CARTESIAN_POINT('Ctrl Pts',(4.02836682984766,287.698925943689,6.91182563342691));
#9386=CARTESIAN_POINT('Ctrl Pts',(2.17634873314619,287.836425943689,7.99122327230091));
#9387=CARTESIAN_POINT('Ctrl Pts',(0.0327551936971994,287.973925943689,8.));
#9388=CARTESIAN_POINT('Ctrl Pts',(-2.11083834575178,288.111425943689,8.00877672769909));
#9389=CARTESIAN_POINT('Ctrl Pts',(-3.97163317015234,288.248925943689,6.94458082712412));
#9390=CARTESIAN_POINT('Ctrl Pts',(-5.83242799455291,288.386425943689,5.88038492654913));
#9391=CARTESIAN_POINT('Ctrl Pts',(-6.91182563342691,288.523925943689,4.02836682984766));
#9392=CARTESIAN_POINT('Ctrl Pts',(-7.99122327230091,288.661425943689,2.17634873314619));
#9393=CARTESIAN_POINT('Ctrl Pts',(-8.,288.798925943689,0.0327551936971979));
#9394=CARTESIAN_POINT('Ctrl Pts',(-8.00877672769909,288.936425943689,-2.11083834575178));
#9395=CARTESIAN_POINT('Ctrl Pts',(-6.94458082712411,289.073925943689,-3.97163317015235));
#9396=CARTESIAN_POINT('Ctrl Pts',(-5.88038492654913,289.211425943689,-5.83242799455291));
#9397=CARTESIAN_POINT('Ctrl Pts',(-4.02836682984766,289.348925943689,-6.91182563342691));
#9398=CARTESIAN_POINT('Ctrl Pts',(-2.17634873314618,289.486425943689,-7.99122327230091));
#9399=CARTESIAN_POINT('Ctrl Pts',(-0.0327551936971984,289.623925943689,
-8.));
#9400=CARTESIAN_POINT('Ctrl Pts',(2.11083834575178,289.761425943689,-8.00877672769909));
#9401=CARTESIAN_POINT('Ctrl Pts',(3.97163317015235,289.898925943689,-6.94458082712411));
#9402=CARTESIAN_POINT('Ctrl Pts',(5.83242799455291,290.036425943689,-5.88038492654913));
#9403=CARTESIAN_POINT('Ctrl Pts',(6.91182563342691,290.173925943689,-4.02836682984766));
#9404=CARTESIAN_POINT('Ctrl Pts',(7.99122327230091,290.311425943689,-2.17634873314618));
#9405=CARTESIAN_POINT('Ctrl Pts',(8.,290.448925943689,-0.0327551936971989));
#9406=CARTESIAN_POINT('Ctrl Pts',(8.00877672769909,290.586425943689,2.11083834575178));
#9407=CARTESIAN_POINT('Ctrl Pts',(6.94458082712411,290.723925943689,3.97163317015235));
#9408=CARTESIAN_POINT('Ctrl Pts',(5.88038492654913,290.861425943689,5.83242799455291));
#9409=CARTESIAN_POINT('Ctrl Pts',(4.02836682984766,290.998925943689,6.91182563342691));
#9410=CARTESIAN_POINT('Ctrl Pts',(2.17634873314619,291.136425943689,7.99122327230091));
#9411=CARTESIAN_POINT('Ctrl Pts',(0.0327551936971994,291.273925943689,8.));
#9412=CARTESIAN_POINT('Ctrl Pts',(-2.11083834575178,291.411425943689,8.00877672769909));
#9413=CARTESIAN_POINT('Ctrl Pts',(-3.97163317015234,291.548925943689,6.94458082712412));
#9414=CARTESIAN_POINT('Ctrl Pts',(-5.83242799455291,291.686425943689,5.88038492654913));
#9415=CARTESIAN_POINT('Ctrl Pts',(-6.91182563342691,291.823925943689,4.02836682984766));
#9416=CARTESIAN_POINT('Ctrl Pts',(-7.99122327230091,291.961425943689,2.17634873314619));
#9417=CARTESIAN_POINT('Ctrl Pts',(-8.,292.098925943689,0.0327551936971979));
#9418=CARTESIAN_POINT('Ctrl Pts',(-8.00877672769909,292.236425943689,-2.11083834575178));
#9419=CARTESIAN_POINT('Ctrl Pts',(-6.94458082712411,292.373925943689,-3.97163317015235));
#9420=CARTESIAN_POINT('Ctrl Pts',(-5.88038492654913,292.511425943689,-5.83242799455291));
#9421=CARTESIAN_POINT('Ctrl Pts',(-4.02836682984766,292.648925943689,-6.91182563342691));
#9422=CARTESIAN_POINT('Ctrl Pts',(-2.17634873314618,292.786425943689,-7.99122327230091));
#9423=CARTESIAN_POINT('Ctrl Pts',(-0.0327551936971984,292.923925943689,
-8.));
#9424=CARTESIAN_POINT('Ctrl Pts',(2.11083834575178,293.061425943689,-8.00877672769909));
#9425=CARTESIAN_POINT('Ctrl Pts',(3.97163317015235,293.198925943689,-6.94458082712411));
#9426=CARTESIAN_POINT('Ctrl Pts',(5.83242799455291,293.336425943689,-5.88038492654913));
#9427=CARTESIAN_POINT('Ctrl Pts',(6.91182563342691,293.473925943689,-4.02836682984766));
#9428=CARTESIAN_POINT('Ctrl Pts',(7.99122327230091,293.611425943689,-2.17634873314618));
#9429=CARTESIAN_POINT('Ctrl Pts',(8.,293.748925943689,-0.0327551936971989));
#9430=CARTESIAN_POINT('Ctrl Pts',(8.00877672769909,293.886425943689,2.11083834575178));
#9431=CARTESIAN_POINT('Ctrl Pts',(6.94458082712411,294.023925943689,3.97163317015235));
#9432=CARTESIAN_POINT('Ctrl Pts',(5.88038492654913,294.161425943689,5.83242799455291));
#9433=CARTESIAN_POINT('Ctrl Pts',(4.02836682984766,294.298925943689,6.91182563342691));
#9434=CARTESIAN_POINT('Ctrl Pts',(2.17634873314619,294.436425943689,7.99122327230091));
#9435=CARTESIAN_POINT('Ctrl Pts',(0.0327551936971994,294.573925943689,8.));
#9436=CARTESIAN_POINT('Ctrl Pts',(-2.11083834575178,294.711425943689,8.00877672769909));
#9437=CARTESIAN_POINT('Ctrl Pts',(-3.97163317015234,294.848925943689,6.94458082712412));
#9438=CARTESIAN_POINT('Ctrl Pts',(-5.83242799455291,294.986425943689,5.88038492654913));
#9439=CARTESIAN_POINT('Ctrl Pts',(-6.91182563342691,295.123925943689,4.02836682984766));
#9440=CARTESIAN_POINT('Ctrl Pts',(-7.99122327230091,295.261425943689,2.17634873314619));
#9441=CARTESIAN_POINT('Ctrl Pts',(-8.,295.398925943689,0.0327551936971979));
#9442=CARTESIAN_POINT('Ctrl Pts',(-8.00877672769909,295.536425943689,-2.11083834575178));
#9443=CARTESIAN_POINT('Ctrl Pts',(-6.94458082712411,295.673925943689,-3.97163317015235));
#9444=CARTESIAN_POINT('Ctrl Pts',(-5.88038492654913,295.811425943689,-5.83242799455291));
#9445=CARTESIAN_POINT('Ctrl Pts',(-4.02836682984766,295.948925943689,-6.91182563342691));
#9446=CARTESIAN_POINT('Ctrl Pts',(-2.17634873314618,296.086425943689,-7.99122327230091));
#9447=CARTESIAN_POINT('Ctrl Pts',(-0.0327551936971984,296.223925943689,
-8.));
#9448=CARTESIAN_POINT('Ctrl Pts',(2.11083834575178,296.361425943689,-8.00877672769909));
#9449=CARTESIAN_POINT('Ctrl Pts',(3.97163317015235,296.498925943689,-6.94458082712411));
#9450=CARTESIAN_POINT('Ctrl Pts',(5.83242799455291,296.636425943689,-5.88038492654913));
#9451=CARTESIAN_POINT('Ctrl Pts',(6.91182563342691,296.773925943689,-4.02836682984766));
#9452=CARTESIAN_POINT('Ctrl Pts',(7.99122327230091,296.911425943689,-2.17634873314618));
#9453=CARTESIAN_POINT('Ctrl Pts',(8.,297.048925943689,-0.0327551936971989));
#9454=CARTESIAN_POINT('Ctrl Pts',(8.00877672769909,297.186425943689,2.11083834575178));
#9455=CARTESIAN_POINT('Ctrl Pts',(6.94458082712411,297.323925943689,3.97163317015235));
#9456=CARTESIAN_POINT('Ctrl Pts',(5.88038492654913,297.461425943689,5.83242799455291));
#9457=CARTESIAN_POINT('Ctrl Pts',(4.02836682984766,297.598925943689,6.91182563342691));
#9458=CARTESIAN_POINT('Ctrl Pts',(2.17634873314619,297.736425943689,7.99122327230091));
#9459=CARTESIAN_POINT('Ctrl Pts',(0.0327551936971994,297.873925943689,8.));
#9460=CARTESIAN_POINT('Ctrl Pts',(-2.11083834575178,298.011425943689,8.00877672769909));
#9461=CARTESIAN_POINT('Ctrl Pts',(-3.97163317015234,298.148925943689,6.94458082712412));
#9462=CARTESIAN_POINT('Ctrl Pts',(-5.83242799455291,298.286425943689,5.88038492654913));
#9463=CARTESIAN_POINT('Ctrl Pts',(-6.91182563342691,298.423925943689,4.02836682984766));
#9464=CARTESIAN_POINT('Ctrl Pts',(-7.99122327230091,298.561425943689,2.17634873314619));
#9465=CARTESIAN_POINT('Ctrl Pts',(-8.,298.698925943689,0.0327551936971979));
#9466=CARTESIAN_POINT('Ctrl Pts',(-8.00877672769909,298.836425943689,-2.11083834575178));
#9467=CARTESIAN_POINT('Ctrl Pts',(-6.94458082712411,298.973925943689,-3.97163317015235));
#9468=CARTESIAN_POINT('Ctrl Pts',(-5.88038492654913,299.111425943689,-5.83242799455291));
#9469=CARTESIAN_POINT('Ctrl Pts',(-4.02836682984766,299.248925943689,-6.91182563342691));
#9470=CARTESIAN_POINT('Ctrl Pts',(-2.17634873314618,299.386425943689,-7.99122327230091));
#9471=CARTESIAN_POINT('Ctrl Pts',(-0.0327551936971984,299.523925943689,
-8.));
#9472=CARTESIAN_POINT('Ctrl Pts',(2.11083834575178,299.661425943689,-8.00877672769909));
#9473=CARTESIAN_POINT('Ctrl Pts',(3.97163317015235,299.798925943689,-6.94458082712411));
#9474=CARTESIAN_POINT('Ctrl Pts',(5.83242799455291,299.936425943689,-5.88038492654913));
#9475=CARTESIAN_POINT('Ctrl Pts',(6.91182563342691,300.073925943689,-4.02836682984766));
#9476=CARTESIAN_POINT('Ctrl Pts',(7.99122327230091,300.211425943689,-2.17634873314618));
#9477=CARTESIAN_POINT('Ctrl Pts',(8.,300.348925943689,-0.0327551936971989));
#9478=CARTESIAN_POINT('Ctrl Pts',(8.00877672769909,300.486425943689,2.11083834575178));
#9479=CARTESIAN_POINT('Ctrl Pts',(6.94458082712411,300.623925943689,3.97163317015235));
#9480=CARTESIAN_POINT('Ctrl Pts',(5.88038492654913,300.761425943689,5.83242799455291));
#9481=CARTESIAN_POINT('Ctrl Pts',(4.02836682984766,300.898925943689,6.91182563342691));
#9482=CARTESIAN_POINT('Ctrl Pts',(2.17634873314619,301.036425943689,7.99122327230091));
#9483=CARTESIAN_POINT('Ctrl Pts',(0.0327551936971994,301.173925943689,8.));
#9484=CARTESIAN_POINT('Ctrl Pts',(-2.11083834575178,301.311425943689,8.00877672769909));
#9485=CARTESIAN_POINT('Ctrl Pts',(-3.97163317015234,301.448925943689,6.94458082712412));
#9486=CARTESIAN_POINT('Ctrl Pts',(-5.83242799455291,301.586425943689,5.88038492654913));
#9487=CARTESIAN_POINT('Ctrl Pts',(-6.91182563342691,301.723925943689,4.02836682984766));
#9488=CARTESIAN_POINT('Ctrl Pts',(-7.99122327230091,301.861425943689,2.17634873314619));
#9489=CARTESIAN_POINT('Ctrl Pts',(-8.,301.998925943689,0.0327551936971979));
#9490=CARTESIAN_POINT('Ctrl Pts',(-8.00877672769909,302.136425943689,-2.11083834575178));
#9491=CARTESIAN_POINT('Ctrl Pts',(-6.94458082712411,302.273925943689,-3.97163317015235));
#9492=CARTESIAN_POINT('Ctrl Pts',(-5.88038492654913,302.411425943689,-5.83242799455291));
#9493=CARTESIAN_POINT('Ctrl Pts',(-4.02836682984766,302.548925943689,-6.91182563342691));
#9494=CARTESIAN_POINT('Ctrl Pts',(-2.17634873314618,302.686425943689,-7.99122327230091));
#9495=CARTESIAN_POINT('Ctrl Pts',(-0.0327551936971984,302.823925943689,
-8.));
#9496=CARTESIAN_POINT('Ctrl Pts',(2.11083834575178,302.961425943689,-8.00877672769909));
#9497=CARTESIAN_POINT('Ctrl Pts',(3.97163317015235,303.098925943689,-6.94458082712411));
#9498=CARTESIAN_POINT('Ctrl Pts',(5.83242799455291,303.236425943689,-5.88038492654913));
#9499=CARTESIAN_POINT('Ctrl Pts',(6.91182563342691,303.373925943689,-4.02836682984766));
#9500=CARTESIAN_POINT('Ctrl Pts',(7.99122327230091,303.511425943689,-2.17634873314618));
#9501=CARTESIAN_POINT('Ctrl Pts',(8.,303.648925943689,-0.0327551936971989));
#9502=CARTESIAN_POINT('Ctrl Pts',(8.00877672769909,303.786425943689,2.11083834575178));
#9503=CARTESIAN_POINT('Ctrl Pts',(6.94458082712411,303.923925943689,3.97163317015235));
#9504=CARTESIAN_POINT('Ctrl Pts',(5.88038492654913,304.061425943689,5.83242799455291));
#9505=CARTESIAN_POINT('Ctrl Pts',(4.02836682984766,304.198925943689,6.91182563342691));
#9506=CARTESIAN_POINT('Ctrl Pts',(2.17634873314619,304.336425943689,7.99122327230091));
#9507=CARTESIAN_POINT('Ctrl Pts',(0.0327551936971994,304.473925943689,8.));
#9508=CARTESIAN_POINT('Ctrl Pts',(-2.11083834575178,304.611425943689,8.00877672769909));
#9509=CARTESIAN_POINT('Ctrl Pts',(-3.97163317015234,304.748925943689,6.94458082712412));
#9510=CARTESIAN_POINT('Ctrl Pts',(-5.83242799455291,304.886425943689,5.88038492654913));
#9511=CARTESIAN_POINT('Ctrl Pts',(-6.91182563342691,305.023925943689,4.02836682984766));
#9512=CARTESIAN_POINT('Ctrl Pts',(-7.99122327230091,305.161425943689,2.17634873314619));
#9513=CARTESIAN_POINT('Ctrl Pts',(-8.,305.298925943689,0.0327551936971979));
#9514=CARTESIAN_POINT('Ctrl Pts',(-8.00877672769909,305.436425943689,-2.11083834575178));
#9515=CARTESIAN_POINT('Ctrl Pts',(-6.94458082712411,305.573925943689,-3.97163317015235));
#9516=CARTESIAN_POINT('Ctrl Pts',(-5.88038492654913,305.711425943689,-5.83242799455291));
#9517=CARTESIAN_POINT('Ctrl Pts',(-4.02836682984766,305.848925943689,-6.91182563342691));
#9518=CARTESIAN_POINT('Ctrl Pts',(-2.17634873314618,305.986425943689,-7.99122327230091));
#9519=CARTESIAN_POINT('Ctrl Pts',(-0.0327551936971984,306.123925943689,
-8.));
#9520=CARTESIAN_POINT('Ctrl Pts',(2.11083834575178,306.261425943689,-8.00877672769909));
#9521=CARTESIAN_POINT('Ctrl Pts',(3.97163317015235,306.398925943689,-6.94458082712411));
#9522=CARTESIAN_POINT('Ctrl Pts',(5.83242799455291,306.536425943689,-5.88038492654913));
#9523=CARTESIAN_POINT('Ctrl Pts',(6.91182563342691,306.673925943689,-4.02836682984766));
#9524=CARTESIAN_POINT('Ctrl Pts',(7.99122327230091,306.811425943689,-2.17634873314618));
#9525=CARTESIAN_POINT('Ctrl Pts',(8.,306.948925943689,-0.0327551936971989));
#9526=CARTESIAN_POINT('Ctrl Pts',(8.00877672769909,307.086425943689,2.11083834575178));
#9527=CARTESIAN_POINT('Ctrl Pts',(6.94458082712411,307.223925943689,3.97163317015235));
#9528=CARTESIAN_POINT('Ctrl Pts',(5.88038492654913,307.361425943689,5.83242799455291));
#9529=CARTESIAN_POINT('Ctrl Pts',(4.02836682984766,307.498925943689,6.91182563342691));
#9530=CARTESIAN_POINT('Ctrl Pts',(2.17634873314619,307.636425943689,7.99122327230091));
#9531=CARTESIAN_POINT('Ctrl Pts',(0.0327551936971994,307.773925943689,8.));
#9532=CARTESIAN_POINT('Ctrl Pts',(-2.11083834575178,307.911425943689,8.00877672769909));
#9533=CARTESIAN_POINT('Ctrl Pts',(-3.97163317015234,308.048925943689,6.94458082712412));
#9534=CARTESIAN_POINT('Ctrl Pts',(-5.83242799455291,308.186425943689,5.88038492654913));
#9535=CARTESIAN_POINT('Ctrl Pts',(-6.91182563342691,308.323925943689,4.02836682984766));
#9536=CARTESIAN_POINT('Ctrl Pts',(-7.99122327230091,308.461425943689,2.17634873314619));
#9537=CARTESIAN_POINT('Ctrl Pts',(-8.,308.598925943689,0.0327551936971979));
#9538=CARTESIAN_POINT('Ctrl Pts',(-8.00877672769909,308.736425943689,-2.11083834575178));
#9539=CARTESIAN_POINT('Ctrl Pts',(-6.94458082712411,308.873925943689,-3.97163317015235));
#9540=CARTESIAN_POINT('Ctrl Pts',(-5.88038492654913,309.011425943689,-5.83242799455291));
#9541=CARTESIAN_POINT('Ctrl Pts',(-4.02836682984766,309.148925943689,-6.91182563342691));
#9542=CARTESIAN_POINT('Ctrl Pts',(-2.17634873314618,309.286425943689,-7.99122327230091));
#9543=CARTESIAN_POINT('Ctrl Pts',(-0.0327551936971984,309.423925943689,
-8.));
#9544=CARTESIAN_POINT('Ctrl Pts',(2.11083834575178,309.561425943689,-8.00877672769909));
#9545=CARTESIAN_POINT('Ctrl Pts',(3.97163317015235,309.698925943689,-6.94458082712411));
#9546=CARTESIAN_POINT('Ctrl Pts',(5.83242799455291,309.836425943689,-5.88038492654913));
#9547=CARTESIAN_POINT('Ctrl Pts',(6.91182563342691,309.973925943689,-4.02836682984766));
#9548=CARTESIAN_POINT('Ctrl Pts',(7.99122327230091,310.111425943689,-2.17634873314618));
#9549=CARTESIAN_POINT('Ctrl Pts',(8.,310.248925943689,-0.0327551936971989));
#9550=CARTESIAN_POINT('Ctrl Pts',(8.00877672769909,310.386425943689,2.11083834575178));
#9551=CARTESIAN_POINT('Ctrl Pts',(6.94458082712411,310.523925943689,3.97163317015235));
#9552=CARTESIAN_POINT('Ctrl Pts',(5.88038492654913,310.661425943689,5.83242799455291));
#9553=CARTESIAN_POINT('Ctrl Pts',(4.02836682984766,310.798925943689,6.91182563342691));
#9554=CARTESIAN_POINT('Ctrl Pts',(2.17634873314619,310.936425943689,7.99122327230091));
#9555=CARTESIAN_POINT('Ctrl Pts',(0.0327551936971994,311.073925943689,8.));
#9556=CARTESIAN_POINT('Ctrl Pts',(-2.11083834575178,311.211425943689,8.00877672769909));
#9557=CARTESIAN_POINT('Ctrl Pts',(-3.97163317015234,311.348925943689,6.94458082712412));
#9558=CARTESIAN_POINT('Ctrl Pts',(-5.83242799455291,311.486425943689,5.88038492654913));
#9559=CARTESIAN_POINT('Ctrl Pts',(-6.91182563342691,311.623925943689,4.02836682984766));
#9560=CARTESIAN_POINT('Ctrl Pts',(-7.99122327230091,311.761425943689,2.17634873314619));
#9561=CARTESIAN_POINT('Ctrl Pts',(-8.,311.898925943689,0.0327551936971979));
#9562=CARTESIAN_POINT('Ctrl Pts',(-8.00877672769909,312.036425943689,-2.11083834575178));
#9563=CARTESIAN_POINT('Ctrl Pts',(-6.94458082712411,312.173925943689,-3.97163317015235));
#9564=CARTESIAN_POINT('Ctrl Pts',(-5.88038492654913,312.311425943689,-5.83242799455291));
#9565=CARTESIAN_POINT('Ctrl Pts',(-4.02836682984766,312.448925943689,-6.91182563342691));
#9566=CARTESIAN_POINT('Ctrl Pts',(-2.17634873314618,312.586425943689,-7.99122327230091));
#9567=CARTESIAN_POINT('Ctrl Pts',(-0.0327551936971984,312.723925943689,
-8.));
#9568=CARTESIAN_POINT('Ctrl Pts',(2.11083834575178,312.861425943689,-8.00877672769909));
#9569=CARTESIAN_POINT('Ctrl Pts',(3.97163317015235,312.998925943689,-6.94458082712411));
#9570=CARTESIAN_POINT('Ctrl Pts',(5.83242799455291,313.136425943689,-5.88038492654913));
#9571=CARTESIAN_POINT('Ctrl Pts',(6.91182563342691,313.273925943689,-4.02836682984766));
#9572=CARTESIAN_POINT('Ctrl Pts',(7.99122327230091,313.411425943689,-2.17634873314618));
#9573=CARTESIAN_POINT('Ctrl Pts',(8.,313.548925943689,-0.0327551936971989));
#9574=CARTESIAN_POINT('Ctrl Pts',(8.00877672769909,313.686425943689,2.11083834575178));
#9575=CARTESIAN_POINT('Ctrl Pts',(6.94458082712411,313.823925943689,3.97163317015235));
#9576=CARTESIAN_POINT('Ctrl Pts',(5.88038492654913,313.961425943689,5.83242799455291));
#9577=CARTESIAN_POINT('Ctrl Pts',(4.02836682984766,314.098925943689,6.91182563342691));
#9578=CARTESIAN_POINT('Ctrl Pts',(2.17634873314619,314.236425943689,7.99122327230091));
#9579=CARTESIAN_POINT('Ctrl Pts',(0.0327551936971994,314.373925943689,8.));
#9580=CARTESIAN_POINT('Ctrl Pts',(-2.11083834575178,314.511425943689,8.00877672769909));
#9581=CARTESIAN_POINT('Ctrl Pts',(-3.97163317015234,314.648925943689,6.94458082712412));
#9582=CARTESIAN_POINT('Ctrl Pts',(-5.83242799455291,314.786425943689,5.88038492654913));
#9583=CARTESIAN_POINT('Ctrl Pts',(-6.91182563342691,314.923925943689,4.02836682984766));
#9584=CARTESIAN_POINT('Ctrl Pts',(-7.99122327230091,315.061425943689,2.17634873314619));
#9585=CARTESIAN_POINT('Ctrl Pts',(-8.,315.198925943689,0.0327551936971979));
#9586=CARTESIAN_POINT('Ctrl Pts',(-8.00877672769909,315.336425943689,-2.11083834575178));
#9587=CARTESIAN_POINT('Ctrl Pts',(-6.94458082712411,315.473925943689,-3.97163317015235));
#9588=CARTESIAN_POINT('Ctrl Pts',(-5.88038492654913,315.611425943689,-5.83242799455291));
#9589=CARTESIAN_POINT('Ctrl Pts',(-4.02836682984766,315.748925943689,-6.91182563342691));
#9590=CARTESIAN_POINT('Ctrl Pts',(-2.17634873314618,315.886425943689,-7.99122327230091));
#9591=CARTESIAN_POINT('Ctrl Pts',(-0.0327551936971984,316.023925943689,
-8.));
#9592=CARTESIAN_POINT('Ctrl Pts',(2.11083834575178,316.161425943689,-8.00877672769909));
#9593=CARTESIAN_POINT('Ctrl Pts',(3.97163317015235,316.298925943689,-6.94458082712411));
#9594=CARTESIAN_POINT('Ctrl Pts',(5.83242799455291,316.436425943689,-5.88038492654913));
#9595=CARTESIAN_POINT('Ctrl Pts',(6.91182563342691,316.573925943689,-4.02836682984766));
#9596=CARTESIAN_POINT('Ctrl Pts',(7.99122327230091,316.711425943689,-2.17634873314618));
#9597=CARTESIAN_POINT('Ctrl Pts',(8.,316.848925943689,-0.0327551936971989));
#9598=CARTESIAN_POINT('Ctrl Pts',(8.00877672769909,316.986425943689,2.11083834575178));
#9599=CARTESIAN_POINT('Ctrl Pts',(6.94458082712411,317.123925943689,3.97163317015235));
#9600=CARTESIAN_POINT('Ctrl Pts',(5.88038492654913,317.261425943689,5.83242799455291));
#9601=CARTESIAN_POINT('Ctrl Pts',(4.02836682984766,317.398925943689,6.91182563342691));
#9602=CARTESIAN_POINT('Ctrl Pts',(2.17634873314619,317.536425943689,7.99122327230091));
#9603=CARTESIAN_POINT('Ctrl Pts',(0.0327551936971994,317.673925943689,8.));
#9604=CARTESIAN_POINT('Ctrl Pts',(-2.11083834575178,317.811425943689,8.00877672769909));
#9605=CARTESIAN_POINT('Ctrl Pts',(-3.97163317015234,317.948925943689,6.94458082712412));
#9606=CARTESIAN_POINT('Ctrl Pts',(-5.83242799455291,318.086425943689,5.88038492654913));
#9607=CARTESIAN_POINT('Ctrl Pts',(-6.91182563342691,318.223925943689,4.02836682984766));
#9608=CARTESIAN_POINT('Ctrl Pts',(-7.99122327230091,318.361425943689,2.17634873314619));
#9609=CARTESIAN_POINT('Ctrl Pts',(-8.,318.498925943689,0.0327551936971979));
#9610=CARTESIAN_POINT('Ctrl Pts',(-7.,285.498925943689,0.0327551936971879));
#9611=CARTESIAN_POINT('Ctrl Pts',(-7.00877672769909,285.636425943689,-1.84288915332067));
#9612=CARTESIAN_POINT('Ctrl Pts',(-6.07855542333967,285.773925943689,-3.47163317015236));
#9613=CARTESIAN_POINT('Ctrl Pts',(-5.14833411898024,285.911425943689,-5.10037718698404));
#9614=CARTESIAN_POINT('Ctrl Pts',(-3.52836682984765,286.048925943689,-6.04580022964248));
#9615=CARTESIAN_POINT('Ctrl Pts',(-1.90839954071505,286.186425943689,-6.99122327230092));
#9616=CARTESIAN_POINT('Ctrl Pts',(-0.0327551936971884,286.323925943689,
-7.));
#9617=CARTESIAN_POINT('Ctrl Pts',(1.84288915332067,286.461425943689,-7.00877672769909));
#9618=CARTESIAN_POINT('Ctrl Pts',(3.47163317015236,286.598925943689,-6.07855542333967));
#9619=CARTESIAN_POINT('Ctrl Pts',(5.10037718698404,286.736425943689,-5.14833411898024));
#9620=CARTESIAN_POINT('Ctrl Pts',(6.04580022964248,286.873925943689,-3.52836682984765));
#9621=CARTESIAN_POINT('Ctrl Pts',(6.99122327230092,287.011425943689,-1.90839954071505));
#9622=CARTESIAN_POINT('Ctrl Pts',(7.,287.148925943689,-0.0327551936971888));
#9623=CARTESIAN_POINT('Ctrl Pts',(7.00877672769909,287.286425943689,1.84288915332067));
#9624=CARTESIAN_POINT('Ctrl Pts',(6.07855542333967,287.423925943689,3.47163317015236));
#9625=CARTESIAN_POINT('Ctrl Pts',(5.14833411898025,287.561425943689,5.10037718698404));
#9626=CARTESIAN_POINT('Ctrl Pts',(3.52836682984765,287.698925943689,6.04580022964248));
#9627=CARTESIAN_POINT('Ctrl Pts',(1.90839954071505,287.836425943689,6.99122327230091));
#9628=CARTESIAN_POINT('Ctrl Pts',(0.0327551936971892,287.973925943689,7.));
#9629=CARTESIAN_POINT('Ctrl Pts',(-1.84288915332067,288.111425943689,7.00877672769909));
#9630=CARTESIAN_POINT('Ctrl Pts',(-3.47163317015235,288.248925943689,6.07855542333967));
#9631=CARTESIAN_POINT('Ctrl Pts',(-5.10037718698404,288.386425943689,5.14833411898025));
#9632=CARTESIAN_POINT('Ctrl Pts',(-6.04580022964248,288.523925943689,3.52836682984765));
#9633=CARTESIAN_POINT('Ctrl Pts',(-6.99122327230091,288.661425943689,1.90839954071505));
#9634=CARTESIAN_POINT('Ctrl Pts',(-7.,288.798925943689,0.0327551936971879));
#9635=CARTESIAN_POINT('Ctrl Pts',(-7.00877672769909,288.936425943689,-1.84288915332067));
#9636=CARTESIAN_POINT('Ctrl Pts',(-6.07855542333967,289.073925943689,-3.47163317015236));
#9637=CARTESIAN_POINT('Ctrl Pts',(-5.14833411898024,289.211425943689,-5.10037718698404));
#9638=CARTESIAN_POINT('Ctrl Pts',(-3.52836682984765,289.348925943689,-6.04580022964248));
#9639=CARTESIAN_POINT('Ctrl Pts',(-1.90839954071505,289.486425943689,-6.99122327230092));
#9640=CARTESIAN_POINT('Ctrl Pts',(-0.0327551936971884,289.623925943689,
-7.));
#9641=CARTESIAN_POINT('Ctrl Pts',(1.84288915332067,289.761425943689,-7.00877672769909));
#9642=CARTESIAN_POINT('Ctrl Pts',(3.47163317015236,289.898925943689,-6.07855542333967));
#9643=CARTESIAN_POINT('Ctrl Pts',(5.10037718698404,290.036425943689,-5.14833411898024));
#9644=CARTESIAN_POINT('Ctrl Pts',(6.04580022964248,290.173925943689,-3.52836682984765));
#9645=CARTESIAN_POINT('Ctrl Pts',(6.99122327230092,290.311425943689,-1.90839954071505));
#9646=CARTESIAN_POINT('Ctrl Pts',(7.,290.448925943689,-0.0327551936971888));
#9647=CARTESIAN_POINT('Ctrl Pts',(7.00877672769909,290.586425943689,1.84288915332067));
#9648=CARTESIAN_POINT('Ctrl Pts',(6.07855542333967,290.723925943689,3.47163317015236));
#9649=CARTESIAN_POINT('Ctrl Pts',(5.14833411898025,290.861425943689,5.10037718698404));
#9650=CARTESIAN_POINT('Ctrl Pts',(3.52836682984765,290.998925943689,6.04580022964248));
#9651=CARTESIAN_POINT('Ctrl Pts',(1.90839954071505,291.136425943689,6.99122327230091));
#9652=CARTESIAN_POINT('Ctrl Pts',(0.0327551936971892,291.273925943689,7.));
#9653=CARTESIAN_POINT('Ctrl Pts',(-1.84288915332067,291.411425943689,7.00877672769909));
#9654=CARTESIAN_POINT('Ctrl Pts',(-3.47163317015235,291.548925943689,6.07855542333967));
#9655=CARTESIAN_POINT('Ctrl Pts',(-5.10037718698404,291.686425943689,5.14833411898025));
#9656=CARTESIAN_POINT('Ctrl Pts',(-6.04580022964248,291.823925943689,3.52836682984765));
#9657=CARTESIAN_POINT('Ctrl Pts',(-6.99122327230091,291.961425943689,1.90839954071505));
#9658=CARTESIAN_POINT('Ctrl Pts',(-7.,292.098925943689,0.0327551936971879));
#9659=CARTESIAN_POINT('Ctrl Pts',(-7.00877672769909,292.236425943689,-1.84288915332067));
#9660=CARTESIAN_POINT('Ctrl Pts',(-6.07855542333967,292.373925943689,-3.47163317015236));
#9661=CARTESIAN_POINT('Ctrl Pts',(-5.14833411898024,292.511425943689,-5.10037718698404));
#9662=CARTESIAN_POINT('Ctrl Pts',(-3.52836682984765,292.648925943689,-6.04580022964248));
#9663=CARTESIAN_POINT('Ctrl Pts',(-1.90839954071505,292.786425943689,-6.99122327230092));
#9664=CARTESIAN_POINT('Ctrl Pts',(-0.0327551936971884,292.923925943689,
-7.));
#9665=CARTESIAN_POINT('Ctrl Pts',(1.84288915332067,293.061425943689,-7.00877672769909));
#9666=CARTESIAN_POINT('Ctrl Pts',(3.47163317015236,293.198925943689,-6.07855542333967));
#9667=CARTESIAN_POINT('Ctrl Pts',(5.10037718698404,293.336425943689,-5.14833411898024));
#9668=CARTESIAN_POINT('Ctrl Pts',(6.04580022964248,293.473925943689,-3.52836682984765));
#9669=CARTESIAN_POINT('Ctrl Pts',(6.99122327230092,293.611425943689,-1.90839954071505));
#9670=CARTESIAN_POINT('Ctrl Pts',(7.,293.748925943689,-0.0327551936971888));
#9671=CARTESIAN_POINT('Ctrl Pts',(7.00877672769909,293.886425943689,1.84288915332067));
#9672=CARTESIAN_POINT('Ctrl Pts',(6.07855542333967,294.023925943689,3.47163317015236));
#9673=CARTESIAN_POINT('Ctrl Pts',(5.14833411898025,294.161425943689,5.10037718698404));
#9674=CARTESIAN_POINT('Ctrl Pts',(3.52836682984765,294.298925943689,6.04580022964248));
#9675=CARTESIAN_POINT('Ctrl Pts',(1.90839954071505,294.436425943689,6.99122327230091));
#9676=CARTESIAN_POINT('Ctrl Pts',(0.0327551936971892,294.573925943689,7.));
#9677=CARTESIAN_POINT('Ctrl Pts',(-1.84288915332067,294.711425943689,7.00877672769909));
#9678=CARTESIAN_POINT('Ctrl Pts',(-3.47163317015235,294.848925943689,6.07855542333967));
#9679=CARTESIAN_POINT('Ctrl Pts',(-5.10037718698404,294.986425943689,5.14833411898025));
#9680=CARTESIAN_POINT('Ctrl Pts',(-6.04580022964248,295.123925943689,3.52836682984765));
#9681=CARTESIAN_POINT('Ctrl Pts',(-6.99122327230091,295.261425943689,1.90839954071505));
#9682=CARTESIAN_POINT('Ctrl Pts',(-7.,295.398925943689,0.0327551936971879));
#9683=CARTESIAN_POINT('Ctrl Pts',(-7.00877672769909,295.536425943689,-1.84288915332067));
#9684=CARTESIAN_POINT('Ctrl Pts',(-6.07855542333967,295.673925943689,-3.47163317015236));
#9685=CARTESIAN_POINT('Ctrl Pts',(-5.14833411898024,295.811425943689,-5.10037718698404));
#9686=CARTESIAN_POINT('Ctrl Pts',(-3.52836682984765,295.948925943689,-6.04580022964248));
#9687=CARTESIAN_POINT('Ctrl Pts',(-1.90839954071505,296.086425943689,-6.99122327230092));
#9688=CARTESIAN_POINT('Ctrl Pts',(-0.0327551936971884,296.223925943689,
-7.));
#9689=CARTESIAN_POINT('Ctrl Pts',(1.84288915332067,296.361425943689,-7.00877672769909));
#9690=CARTESIAN_POINT('Ctrl Pts',(3.47163317015236,296.498925943689,-6.07855542333967));
#9691=CARTESIAN_POINT('Ctrl Pts',(5.10037718698404,296.636425943689,-5.14833411898024));
#9692=CARTESIAN_POINT('Ctrl Pts',(6.04580022964248,296.773925943689,-3.52836682984765));
#9693=CARTESIAN_POINT('Ctrl Pts',(6.99122327230092,296.911425943689,-1.90839954071505));
#9694=CARTESIAN_POINT('Ctrl Pts',(7.,297.048925943689,-0.0327551936971888));
#9695=CARTESIAN_POINT('Ctrl Pts',(7.00877672769909,297.186425943689,1.84288915332067));
#9696=CARTESIAN_POINT('Ctrl Pts',(6.07855542333967,297.323925943689,3.47163317015236));
#9697=CARTESIAN_POINT('Ctrl Pts',(5.14833411898025,297.461425943689,5.10037718698404));
#9698=CARTESIAN_POINT('Ctrl Pts',(3.52836682984765,297.598925943689,6.04580022964248));
#9699=CARTESIAN_POINT('Ctrl Pts',(1.90839954071505,297.736425943689,6.99122327230091));
#9700=CARTESIAN_POINT('Ctrl Pts',(0.0327551936971892,297.873925943689,7.));
#9701=CARTESIAN_POINT('Ctrl Pts',(-1.84288915332067,298.011425943689,7.00877672769909));
#9702=CARTESIAN_POINT('Ctrl Pts',(-3.47163317015235,298.148925943689,6.07855542333967));
#9703=CARTESIAN_POINT('Ctrl Pts',(-5.10037718698404,298.286425943689,5.14833411898025));
#9704=CARTESIAN_POINT('Ctrl Pts',(-6.04580022964248,298.423925943689,3.52836682984765));
#9705=CARTESIAN_POINT('Ctrl Pts',(-6.99122327230091,298.561425943689,1.90839954071505));
#9706=CARTESIAN_POINT('Ctrl Pts',(-7.,298.698925943689,0.0327551936971879));
#9707=CARTESIAN_POINT('Ctrl Pts',(-7.00877672769909,298.836425943689,-1.84288915332067));
#9708=CARTESIAN_POINT('Ctrl Pts',(-6.07855542333967,298.973925943689,-3.47163317015236));
#9709=CARTESIAN_POINT('Ctrl Pts',(-5.14833411898024,299.111425943689,-5.10037718698404));
#9710=CARTESIAN_POINT('Ctrl Pts',(-3.52836682984765,299.248925943689,-6.04580022964248));
#9711=CARTESIAN_POINT('Ctrl Pts',(-1.90839954071505,299.386425943689,-6.99122327230092));
#9712=CARTESIAN_POINT('Ctrl Pts',(-0.0327551936971884,299.523925943689,
-7.));
#9713=CARTESIAN_POINT('Ctrl Pts',(1.84288915332067,299.661425943689,-7.00877672769909));
#9714=CARTESIAN_POINT('Ctrl Pts',(3.47163317015236,299.798925943689,-6.07855542333967));
#9715=CARTESIAN_POINT('Ctrl Pts',(5.10037718698404,299.936425943689,-5.14833411898024));
#9716=CARTESIAN_POINT('Ctrl Pts',(6.04580022964248,300.073925943689,-3.52836682984765));
#9717=CARTESIAN_POINT('Ctrl Pts',(6.99122327230092,300.211425943689,-1.90839954071505));
#9718=CARTESIAN_POINT('Ctrl Pts',(7.,300.348925943689,-0.0327551936971888));
#9719=CARTESIAN_POINT('Ctrl Pts',(7.00877672769909,300.486425943689,1.84288915332067));
#9720=CARTESIAN_POINT('Ctrl Pts',(6.07855542333967,300.623925943689,3.47163317015236));
#9721=CARTESIAN_POINT('Ctrl Pts',(5.14833411898025,300.761425943689,5.10037718698404));
#9722=CARTESIAN_POINT('Ctrl Pts',(3.52836682984765,300.898925943689,6.04580022964248));
#9723=CARTESIAN_POINT('Ctrl Pts',(1.90839954071505,301.036425943689,6.99122327230091));
#9724=CARTESIAN_POINT('Ctrl Pts',(0.0327551936971892,301.173925943689,7.));
#9725=CARTESIAN_POINT('Ctrl Pts',(-1.84288915332067,301.311425943689,7.00877672769909));
#9726=CARTESIAN_POINT('Ctrl Pts',(-3.47163317015235,301.448925943689,6.07855542333967));
#9727=CARTESIAN_POINT('Ctrl Pts',(-5.10037718698404,301.586425943689,5.14833411898025));
#9728=CARTESIAN_POINT('Ctrl Pts',(-6.04580022964248,301.723925943689,3.52836682984765));
#9729=CARTESIAN_POINT('Ctrl Pts',(-6.99122327230091,301.861425943689,1.90839954071505));
#9730=CARTESIAN_POINT('Ctrl Pts',(-7.,301.998925943689,0.0327551936971879));
#9731=CARTESIAN_POINT('Ctrl Pts',(-7.00877672769909,302.136425943689,-1.84288915332067));
#9732=CARTESIAN_POINT('Ctrl Pts',(-6.07855542333967,302.273925943689,-3.47163317015236));
#9733=CARTESIAN_POINT('Ctrl Pts',(-5.14833411898024,302.411425943689,-5.10037718698404));
#9734=CARTESIAN_POINT('Ctrl Pts',(-3.52836682984765,302.548925943689,-6.04580022964248));
#9735=CARTESIAN_POINT('Ctrl Pts',(-1.90839954071505,302.686425943689,-6.99122327230092));
#9736=CARTESIAN_POINT('Ctrl Pts',(-0.0327551936971884,302.823925943689,
-7.));
#9737=CARTESIAN_POINT('Ctrl Pts',(1.84288915332067,302.961425943689,-7.00877672769909));
#9738=CARTESIAN_POINT('Ctrl Pts',(3.47163317015236,303.098925943689,-6.07855542333967));
#9739=CARTESIAN_POINT('Ctrl Pts',(5.10037718698404,303.236425943689,-5.14833411898024));
#9740=CARTESIAN_POINT('Ctrl Pts',(6.04580022964248,303.373925943689,-3.52836682984765));
#9741=CARTESIAN_POINT('Ctrl Pts',(6.99122327230092,303.511425943689,-1.90839954071505));
#9742=CARTESIAN_POINT('Ctrl Pts',(7.,303.648925943689,-0.0327551936971888));
#9743=CARTESIAN_POINT('Ctrl Pts',(7.00877672769909,303.786425943689,1.84288915332067));
#9744=CARTESIAN_POINT('Ctrl Pts',(6.07855542333967,303.923925943689,3.47163317015236));
#9745=CARTESIAN_POINT('Ctrl Pts',(5.14833411898025,304.061425943689,5.10037718698404));
#9746=CARTESIAN_POINT('Ctrl Pts',(3.52836682984765,304.198925943689,6.04580022964248));
#9747=CARTESIAN_POINT('Ctrl Pts',(1.90839954071505,304.336425943689,6.99122327230091));
#9748=CARTESIAN_POINT('Ctrl Pts',(0.0327551936971892,304.473925943689,7.));
#9749=CARTESIAN_POINT('Ctrl Pts',(-1.84288915332067,304.611425943689,7.00877672769909));
#9750=CARTESIAN_POINT('Ctrl Pts',(-3.47163317015235,304.748925943689,6.07855542333967));
#9751=CARTESIAN_POINT('Ctrl Pts',(-5.10037718698404,304.886425943689,5.14833411898025));
#9752=CARTESIAN_POINT('Ctrl Pts',(-6.04580022964248,305.023925943689,3.52836682984765));
#9753=CARTESIAN_POINT('Ctrl Pts',(-6.99122327230091,305.161425943689,1.90839954071505));
#9754=CARTESIAN_POINT('Ctrl Pts',(-7.,305.298925943689,0.0327551936971879));
#9755=CARTESIAN_POINT('Ctrl Pts',(-7.00877672769909,305.436425943689,-1.84288915332067));
#9756=CARTESIAN_POINT('Ctrl Pts',(-6.07855542333967,305.573925943689,-3.47163317015236));
#9757=CARTESIAN_POINT('Ctrl Pts',(-5.14833411898024,305.711425943689,-5.10037718698404));
#9758=CARTESIAN_POINT('Ctrl Pts',(-3.52836682984765,305.848925943689,-6.04580022964248));
#9759=CARTESIAN_POINT('Ctrl Pts',(-1.90839954071505,305.986425943689,-6.99122327230092));
#9760=CARTESIAN_POINT('Ctrl Pts',(-0.0327551936971884,306.123925943689,
-7.));
#9761=CARTESIAN_POINT('Ctrl Pts',(1.84288915332067,306.261425943689,-7.00877672769909));
#9762=CARTESIAN_POINT('Ctrl Pts',(3.47163317015236,306.398925943689,-6.07855542333967));
#9763=CARTESIAN_POINT('Ctrl Pts',(5.10037718698404,306.536425943689,-5.14833411898024));
#9764=CARTESIAN_POINT('Ctrl Pts',(6.04580022964248,306.673925943689,-3.52836682984765));
#9765=CARTESIAN_POINT('Ctrl Pts',(6.99122327230092,306.811425943689,-1.90839954071505));
#9766=CARTESIAN_POINT('Ctrl Pts',(7.,306.948925943689,-0.0327551936971888));
#9767=CARTESIAN_POINT('Ctrl Pts',(7.00877672769909,307.086425943689,1.84288915332067));
#9768=CARTESIAN_POINT('Ctrl Pts',(6.07855542333967,307.223925943689,3.47163317015236));
#9769=CARTESIAN_POINT('Ctrl Pts',(5.14833411898025,307.361425943689,5.10037718698404));
#9770=CARTESIAN_POINT('Ctrl Pts',(3.52836682984765,307.498925943689,6.04580022964248));
#9771=CARTESIAN_POINT('Ctrl Pts',(1.90839954071505,307.636425943689,6.99122327230091));
#9772=CARTESIAN_POINT('Ctrl Pts',(0.0327551936971892,307.773925943689,7.));
#9773=CARTESIAN_POINT('Ctrl Pts',(-1.84288915332067,307.911425943689,7.00877672769909));
#9774=CARTESIAN_POINT('Ctrl Pts',(-3.47163317015235,308.048925943689,6.07855542333967));
#9775=CARTESIAN_POINT('Ctrl Pts',(-5.10037718698404,308.186425943689,5.14833411898025));
#9776=CARTESIAN_POINT('Ctrl Pts',(-6.04580022964248,308.323925943689,3.52836682984765));
#9777=CARTESIAN_POINT('Ctrl Pts',(-6.99122327230091,308.461425943689,1.90839954071505));
#9778=CARTESIAN_POINT('Ctrl Pts',(-7.,308.598925943689,0.0327551936971879));
#9779=CARTESIAN_POINT('Ctrl Pts',(-7.00877672769909,308.736425943689,-1.84288915332067));
#9780=CARTESIAN_POINT('Ctrl Pts',(-6.07855542333967,308.873925943689,-3.47163317015236));
#9781=CARTESIAN_POINT('Ctrl Pts',(-5.14833411898024,309.011425943689,-5.10037718698404));
#9782=CARTESIAN_POINT('Ctrl Pts',(-3.52836682984765,309.148925943689,-6.04580022964248));
#9783=CARTESIAN_POINT('Ctrl Pts',(-1.90839954071505,309.286425943689,-6.99122327230092));
#9784=CARTESIAN_POINT('Ctrl Pts',(-0.0327551936971884,309.423925943689,
-7.));
#9785=CARTESIAN_POINT('Ctrl Pts',(1.84288915332067,309.561425943689,-7.00877672769909));
#9786=CARTESIAN_POINT('Ctrl Pts',(3.47163317015236,309.698925943689,-6.07855542333967));
#9787=CARTESIAN_POINT('Ctrl Pts',(5.10037718698404,309.836425943689,-5.14833411898024));
#9788=CARTESIAN_POINT('Ctrl Pts',(6.04580022964248,309.973925943689,-3.52836682984765));
#9789=CARTESIAN_POINT('Ctrl Pts',(6.99122327230092,310.111425943689,-1.90839954071505));
#9790=CARTESIAN_POINT('Ctrl Pts',(7.,310.248925943689,-0.0327551936971888));
#9791=CARTESIAN_POINT('Ctrl Pts',(7.00877672769909,310.386425943689,1.84288915332067));
#9792=CARTESIAN_POINT('Ctrl Pts',(6.07855542333967,310.523925943689,3.47163317015236));
#9793=CARTESIAN_POINT('Ctrl Pts',(5.14833411898025,310.661425943689,5.10037718698404));
#9794=CARTESIAN_POINT('Ctrl Pts',(3.52836682984765,310.798925943689,6.04580022964248));
#9795=CARTESIAN_POINT('Ctrl Pts',(1.90839954071505,310.936425943689,6.99122327230091));
#9796=CARTESIAN_POINT('Ctrl Pts',(0.0327551936971892,311.073925943689,7.));
#9797=CARTESIAN_POINT('Ctrl Pts',(-1.84288915332067,311.211425943689,7.00877672769909));
#9798=CARTESIAN_POINT('Ctrl Pts',(-3.47163317015235,311.348925943689,6.07855542333967));
#9799=CARTESIAN_POINT('Ctrl Pts',(-5.10037718698404,311.486425943689,5.14833411898025));
#9800=CARTESIAN_POINT('Ctrl Pts',(-6.04580022964248,311.623925943689,3.52836682984765));
#9801=CARTESIAN_POINT('Ctrl Pts',(-6.99122327230091,311.761425943689,1.90839954071505));
#9802=CARTESIAN_POINT('Ctrl Pts',(-7.,311.898925943689,0.0327551936971879));
#9803=CARTESIAN_POINT('Ctrl Pts',(-7.00877672769909,312.036425943689,-1.84288915332067));
#9804=CARTESIAN_POINT('Ctrl Pts',(-6.07855542333967,312.173925943689,-3.47163317015236));
#9805=CARTESIAN_POINT('Ctrl Pts',(-5.14833411898024,312.311425943689,-5.10037718698404));
#9806=CARTESIAN_POINT('Ctrl Pts',(-3.52836682984765,312.448925943689,-6.04580022964248));
#9807=CARTESIAN_POINT('Ctrl Pts',(-1.90839954071505,312.586425943689,-6.99122327230092));
#9808=CARTESIAN_POINT('Ctrl Pts',(-0.0327551936971884,312.723925943689,
-7.));
#9809=CARTESIAN_POINT('Ctrl Pts',(1.84288915332067,312.861425943689,-7.00877672769909));
#9810=CARTESIAN_POINT('Ctrl Pts',(3.47163317015236,312.998925943689,-6.07855542333967));
#9811=CARTESIAN_POINT('Ctrl Pts',(5.10037718698404,313.136425943689,-5.14833411898024));
#9812=CARTESIAN_POINT('Ctrl Pts',(6.04580022964248,313.273925943689,-3.52836682984765));
#9813=CARTESIAN_POINT('Ctrl Pts',(6.99122327230092,313.411425943689,-1.90839954071505));
#9814=CARTESIAN_POINT('Ctrl Pts',(7.,313.548925943689,-0.0327551936971888));
#9815=CARTESIAN_POINT('Ctrl Pts',(7.00877672769909,313.686425943689,1.84288915332067));
#9816=CARTESIAN_POINT('Ctrl Pts',(6.07855542333967,313.823925943689,3.47163317015236));
#9817=CARTESIAN_POINT('Ctrl Pts',(5.14833411898025,313.961425943689,5.10037718698404));
#9818=CARTESIAN_POINT('Ctrl Pts',(3.52836682984765,314.098925943689,6.04580022964248));
#9819=CARTESIAN_POINT('Ctrl Pts',(1.90839954071505,314.236425943689,6.99122327230091));
#9820=CARTESIAN_POINT('Ctrl Pts',(0.0327551936971892,314.373925943689,7.));
#9821=CARTESIAN_POINT('Ctrl Pts',(-1.84288915332067,314.511425943689,7.00877672769909));
#9822=CARTESIAN_POINT('Ctrl Pts',(-3.47163317015235,314.648925943689,6.07855542333967));
#9823=CARTESIAN_POINT('Ctrl Pts',(-5.10037718698404,314.786425943689,5.14833411898025));
#9824=CARTESIAN_POINT('Ctrl Pts',(-6.04580022964248,314.923925943689,3.52836682984765));
#9825=CARTESIAN_POINT('Ctrl Pts',(-6.99122327230091,315.061425943689,1.90839954071505));
#9826=CARTESIAN_POINT('Ctrl Pts',(-7.,315.198925943689,0.0327551936971879));
#9827=CARTESIAN_POINT('Ctrl Pts',(-7.00877672769909,315.336425943689,-1.84288915332067));
#9828=CARTESIAN_POINT('Ctrl Pts',(-6.07855542333967,315.473925943689,-3.47163317015236));
#9829=CARTESIAN_POINT('Ctrl Pts',(-5.14833411898024,315.611425943689,-5.10037718698404));
#9830=CARTESIAN_POINT('Ctrl Pts',(-3.52836682984765,315.748925943689,-6.04580022964248));
#9831=CARTESIAN_POINT('Ctrl Pts',(-1.90839954071505,315.886425943689,-6.99122327230092));
#9832=CARTESIAN_POINT('Ctrl Pts',(-0.0327551936971884,316.023925943689,
-7.));
#9833=CARTESIAN_POINT('Ctrl Pts',(1.84288915332067,316.161425943689,-7.00877672769909));
#9834=CARTESIAN_POINT('Ctrl Pts',(3.47163317015236,316.298925943689,-6.07855542333967));
#9835=CARTESIAN_POINT('Ctrl Pts',(5.10037718698404,316.436425943689,-5.14833411898024));
#9836=CARTESIAN_POINT('Ctrl Pts',(6.04580022964248,316.573925943689,-3.52836682984765));
#9837=CARTESIAN_POINT('Ctrl Pts',(6.99122327230092,316.711425943689,-1.90839954071505));
#9838=CARTESIAN_POINT('Ctrl Pts',(7.,316.848925943689,-0.0327551936971888));
#9839=CARTESIAN_POINT('Ctrl Pts',(7.00877672769909,316.986425943689,1.84288915332067));
#9840=CARTESIAN_POINT('Ctrl Pts',(6.07855542333967,317.123925943689,3.47163317015236));
#9841=CARTESIAN_POINT('Ctrl Pts',(5.14833411898025,317.261425943689,5.10037718698404));
#9842=CARTESIAN_POINT('Ctrl Pts',(3.52836682984765,317.398925943689,6.04580022964248));
#9843=CARTESIAN_POINT('Ctrl Pts',(1.90839954071505,317.536425943689,6.99122327230091));
#9844=CARTESIAN_POINT('Ctrl Pts',(0.0327551936971892,317.673925943689,7.));
#9845=CARTESIAN_POINT('Ctrl Pts',(-1.84288915332067,317.811425943689,7.00877672769909));
#9846=CARTESIAN_POINT('Ctrl Pts',(-3.47163317015235,317.948925943689,6.07855542333967));
#9847=CARTESIAN_POINT('Ctrl Pts',(-5.10037718698404,318.086425943689,5.14833411898025));
#9848=CARTESIAN_POINT('Ctrl Pts',(-6.04580022964248,318.223925943689,3.52836682984765));
#9849=CARTESIAN_POINT('Ctrl Pts',(-6.99122327230091,318.361425943689,1.90839954071505));
#9850=CARTESIAN_POINT('Ctrl Pts',(-7.,318.498925943689,0.0327551936971879));
#9851=CARTESIAN_POINT('Ctrl Pts',(-7.,284.501074056311,-0.0327551936970413));
#9852=CARTESIAN_POINT('Ctrl Pts',(-6.99122327230096,284.638574056311,-1.9083995407149));
#9853=CARTESIAN_POINT('Ctrl Pts',(-6.04580022964255,284.776074056311,-3.52836682984752));
#9854=CARTESIAN_POINT('Ctrl Pts',(-5.10037718698415,284.913574056311,-5.14833411898014));
#9855=CARTESIAN_POINT('Ctrl Pts',(-3.47163317015249,285.051074056311,-6.07855542333959));
#9856=CARTESIAN_POINT('Ctrl Pts',(-1.84288915332082,285.188574056311,-7.00877672769905));
#9857=CARTESIAN_POINT('Ctrl Pts',(0.0327551936970409,285.326074056311,-7.));
#9858=CARTESIAN_POINT('Ctrl Pts',(1.9083995407149,285.463574056311,-6.99122327230096));
#9859=CARTESIAN_POINT('Ctrl Pts',(3.52836682984752,285.601074056311,-6.04580022964255));
#9860=CARTESIAN_POINT('Ctrl Pts',(5.14833411898014,285.738574056311,-5.10037718698415));
#9861=CARTESIAN_POINT('Ctrl Pts',(6.07855542333959,285.876074056311,-3.47163317015249));
#9862=CARTESIAN_POINT('Ctrl Pts',(7.00877672769905,286.013574056311,-1.84288915332082));
#9863=CARTESIAN_POINT('Ctrl Pts',(7.,286.151074056311,0.0327551936970405));
#9864=CARTESIAN_POINT('Ctrl Pts',(6.99122327230096,286.288574056311,1.9083995407149));
#9865=CARTESIAN_POINT('Ctrl Pts',(6.04580022964255,286.426074056311,3.52836682984752));
#9866=CARTESIAN_POINT('Ctrl Pts',(5.10037718698415,286.563574056311,5.14833411898013));
#9867=CARTESIAN_POINT('Ctrl Pts',(3.47163317015249,286.701074056311,6.07855542333959));
#9868=CARTESIAN_POINT('Ctrl Pts',(1.84288915332082,286.838574056311,7.00877672769905));
#9869=CARTESIAN_POINT('Ctrl Pts',(-0.03275519369704,286.976074056311,7.));
#9870=CARTESIAN_POINT('Ctrl Pts',(-1.9083995407149,287.113574056311,6.99122327230096));
#9871=CARTESIAN_POINT('Ctrl Pts',(-3.52836682984752,287.251074056311,6.04580022964255));
#9872=CARTESIAN_POINT('Ctrl Pts',(-5.14833411898014,287.388574056311,5.10037718698415));
#9873=CARTESIAN_POINT('Ctrl Pts',(-6.07855542333959,287.526074056311,3.47163317015249));
#9874=CARTESIAN_POINT('Ctrl Pts',(-7.00877672769905,287.663574056311,1.84288915332082));
#9875=CARTESIAN_POINT('Ctrl Pts',(-7.,287.801074056311,-0.0327551936970413));
#9876=CARTESIAN_POINT('Ctrl Pts',(-6.99122327230096,287.938574056311,-1.9083995407149));
#9877=CARTESIAN_POINT('Ctrl Pts',(-6.04580022964255,288.076074056311,-3.52836682984752));
#9878=CARTESIAN_POINT('Ctrl Pts',(-5.10037718698415,288.213574056311,-5.14833411898014));
#9879=CARTESIAN_POINT('Ctrl Pts',(-3.47163317015249,288.351074056311,-6.07855542333959));
#9880=CARTESIAN_POINT('Ctrl Pts',(-1.84288915332082,288.488574056311,-7.00877672769905));
#9881=CARTESIAN_POINT('Ctrl Pts',(0.0327551936970409,288.626074056311,-7.));
#9882=CARTESIAN_POINT('Ctrl Pts',(1.9083995407149,288.763574056311,-6.99122327230096));
#9883=CARTESIAN_POINT('Ctrl Pts',(3.52836682984752,288.901074056311,-6.04580022964255));
#9884=CARTESIAN_POINT('Ctrl Pts',(5.14833411898014,289.038574056311,-5.10037718698415));
#9885=CARTESIAN_POINT('Ctrl Pts',(6.07855542333959,289.176074056311,-3.47163317015249));
#9886=CARTESIAN_POINT('Ctrl Pts',(7.00877672769905,289.313574056311,-1.84288915332082));
#9887=CARTESIAN_POINT('Ctrl Pts',(7.,289.451074056311,0.0327551936970405));
#9888=CARTESIAN_POINT('Ctrl Pts',(6.99122327230096,289.588574056311,1.9083995407149));
#9889=CARTESIAN_POINT('Ctrl Pts',(6.04580022964255,289.726074056311,3.52836682984752));
#9890=CARTESIAN_POINT('Ctrl Pts',(5.10037718698415,289.863574056311,5.14833411898013));
#9891=CARTESIAN_POINT('Ctrl Pts',(3.47163317015249,290.001074056311,6.07855542333959));
#9892=CARTESIAN_POINT('Ctrl Pts',(1.84288915332082,290.138574056311,7.00877672769905));
#9893=CARTESIAN_POINT('Ctrl Pts',(-0.03275519369704,290.276074056311,7.));
#9894=CARTESIAN_POINT('Ctrl Pts',(-1.9083995407149,290.413574056311,6.99122327230096));
#9895=CARTESIAN_POINT('Ctrl Pts',(-3.52836682984752,290.551074056311,6.04580022964255));
#9896=CARTESIAN_POINT('Ctrl Pts',(-5.14833411898014,290.688574056311,5.10037718698415));
#9897=CARTESIAN_POINT('Ctrl Pts',(-6.07855542333959,290.826074056311,3.47163317015249));
#9898=CARTESIAN_POINT('Ctrl Pts',(-7.00877672769905,290.963574056311,1.84288915332082));
#9899=CARTESIAN_POINT('Ctrl Pts',(-7.,291.101074056311,-0.0327551936970413));
#9900=CARTESIAN_POINT('Ctrl Pts',(-6.99122327230096,291.238574056311,-1.9083995407149));
#9901=CARTESIAN_POINT('Ctrl Pts',(-6.04580022964255,291.376074056311,-3.52836682984752));
#9902=CARTESIAN_POINT('Ctrl Pts',(-5.10037718698415,291.513574056311,-5.14833411898014));
#9903=CARTESIAN_POINT('Ctrl Pts',(-3.47163317015249,291.651074056311,-6.07855542333959));
#9904=CARTESIAN_POINT('Ctrl Pts',(-1.84288915332082,291.788574056311,-7.00877672769905));
#9905=CARTESIAN_POINT('Ctrl Pts',(0.0327551936970409,291.926074056311,-7.));
#9906=CARTESIAN_POINT('Ctrl Pts',(1.9083995407149,292.063574056311,-6.99122327230096));
#9907=CARTESIAN_POINT('Ctrl Pts',(3.52836682984752,292.201074056311,-6.04580022964255));
#9908=CARTESIAN_POINT('Ctrl Pts',(5.14833411898014,292.338574056311,-5.10037718698415));
#9909=CARTESIAN_POINT('Ctrl Pts',(6.07855542333959,292.476074056311,-3.47163317015249));
#9910=CARTESIAN_POINT('Ctrl Pts',(7.00877672769905,292.613574056311,-1.84288915332082));
#9911=CARTESIAN_POINT('Ctrl Pts',(7.,292.751074056311,0.0327551936970405));
#9912=CARTESIAN_POINT('Ctrl Pts',(6.99122327230096,292.888574056311,1.9083995407149));
#9913=CARTESIAN_POINT('Ctrl Pts',(6.04580022964255,293.026074056311,3.52836682984752));
#9914=CARTESIAN_POINT('Ctrl Pts',(5.10037718698415,293.163574056311,5.14833411898013));
#9915=CARTESIAN_POINT('Ctrl Pts',(3.47163317015249,293.301074056311,6.07855542333959));
#9916=CARTESIAN_POINT('Ctrl Pts',(1.84288915332082,293.438574056311,7.00877672769905));
#9917=CARTESIAN_POINT('Ctrl Pts',(-0.03275519369704,293.576074056311,7.));
#9918=CARTESIAN_POINT('Ctrl Pts',(-1.9083995407149,293.713574056311,6.99122327230096));
#9919=CARTESIAN_POINT('Ctrl Pts',(-3.52836682984752,293.851074056311,6.04580022964255));
#9920=CARTESIAN_POINT('Ctrl Pts',(-5.14833411898014,293.988574056311,5.10037718698415));
#9921=CARTESIAN_POINT('Ctrl Pts',(-6.07855542333959,294.126074056311,3.47163317015249));
#9922=CARTESIAN_POINT('Ctrl Pts',(-7.00877672769905,294.263574056311,1.84288915332082));
#9923=CARTESIAN_POINT('Ctrl Pts',(-7.,294.401074056311,-0.0327551936970413));
#9924=CARTESIAN_POINT('Ctrl Pts',(-6.99122327230096,294.538574056311,-1.9083995407149));
#9925=CARTESIAN_POINT('Ctrl Pts',(-6.04580022964255,294.676074056311,-3.52836682984752));
#9926=CARTESIAN_POINT('Ctrl Pts',(-5.10037718698415,294.813574056311,-5.14833411898014));
#9927=CARTESIAN_POINT('Ctrl Pts',(-3.47163317015249,294.951074056311,-6.07855542333959));
#9928=CARTESIAN_POINT('Ctrl Pts',(-1.84288915332082,295.088574056311,-7.00877672769905));
#9929=CARTESIAN_POINT('Ctrl Pts',(0.0327551936970409,295.226074056311,-7.));
#9930=CARTESIAN_POINT('Ctrl Pts',(1.9083995407149,295.363574056311,-6.99122327230096));
#9931=CARTESIAN_POINT('Ctrl Pts',(3.52836682984752,295.501074056311,-6.04580022964255));
#9932=CARTESIAN_POINT('Ctrl Pts',(5.14833411898014,295.638574056311,-5.10037718698415));
#9933=CARTESIAN_POINT('Ctrl Pts',(6.07855542333959,295.776074056311,-3.47163317015249));
#9934=CARTESIAN_POINT('Ctrl Pts',(7.00877672769905,295.913574056311,-1.84288915332082));
#9935=CARTESIAN_POINT('Ctrl Pts',(7.,296.051074056311,0.0327551936970405));
#9936=CARTESIAN_POINT('Ctrl Pts',(6.99122327230096,296.188574056311,1.9083995407149));
#9937=CARTESIAN_POINT('Ctrl Pts',(6.04580022964255,296.326074056311,3.52836682984752));
#9938=CARTESIAN_POINT('Ctrl Pts',(5.10037718698415,296.463574056311,5.14833411898013));
#9939=CARTESIAN_POINT('Ctrl Pts',(3.47163317015249,296.601074056311,6.07855542333959));
#9940=CARTESIAN_POINT('Ctrl Pts',(1.84288915332082,296.738574056311,7.00877672769905));
#9941=CARTESIAN_POINT('Ctrl Pts',(-0.03275519369704,296.876074056311,7.));
#9942=CARTESIAN_POINT('Ctrl Pts',(-1.9083995407149,297.013574056311,6.99122327230096));
#9943=CARTESIAN_POINT('Ctrl Pts',(-3.52836682984752,297.151074056311,6.04580022964255));
#9944=CARTESIAN_POINT('Ctrl Pts',(-5.14833411898014,297.288574056311,5.10037718698415));
#9945=CARTESIAN_POINT('Ctrl Pts',(-6.07855542333959,297.426074056311,3.47163317015249));
#9946=CARTESIAN_POINT('Ctrl Pts',(-7.00877672769905,297.563574056311,1.84288915332082));
#9947=CARTESIAN_POINT('Ctrl Pts',(-7.,297.701074056311,-0.0327551936970413));
#9948=CARTESIAN_POINT('Ctrl Pts',(-6.99122327230096,297.838574056311,-1.9083995407149));
#9949=CARTESIAN_POINT('Ctrl Pts',(-6.04580022964255,297.976074056311,-3.52836682984752));
#9950=CARTESIAN_POINT('Ctrl Pts',(-5.10037718698415,298.113574056311,-5.14833411898014));
#9951=CARTESIAN_POINT('Ctrl Pts',(-3.47163317015249,298.251074056311,-6.07855542333959));
#9952=CARTESIAN_POINT('Ctrl Pts',(-1.84288915332082,298.388574056311,-7.00877672769905));
#9953=CARTESIAN_POINT('Ctrl Pts',(0.0327551936970409,298.526074056311,-7.));
#9954=CARTESIAN_POINT('Ctrl Pts',(1.9083995407149,298.663574056311,-6.99122327230096));
#9955=CARTESIAN_POINT('Ctrl Pts',(3.52836682984752,298.801074056311,-6.04580022964255));
#9956=CARTESIAN_POINT('Ctrl Pts',(5.14833411898014,298.938574056311,-5.10037718698415));
#9957=CARTESIAN_POINT('Ctrl Pts',(6.07855542333959,299.076074056311,-3.47163317015249));
#9958=CARTESIAN_POINT('Ctrl Pts',(7.00877672769905,299.213574056311,-1.84288915332082));
#9959=CARTESIAN_POINT('Ctrl Pts',(7.,299.351074056311,0.0327551936970405));
#9960=CARTESIAN_POINT('Ctrl Pts',(6.99122327230096,299.488574056311,1.9083995407149));
#9961=CARTESIAN_POINT('Ctrl Pts',(6.04580022964255,299.626074056311,3.52836682984752));
#9962=CARTESIAN_POINT('Ctrl Pts',(5.10037718698415,299.763574056311,5.14833411898013));
#9963=CARTESIAN_POINT('Ctrl Pts',(3.47163317015249,299.901074056311,6.07855542333959));
#9964=CARTESIAN_POINT('Ctrl Pts',(1.84288915332082,300.038574056311,7.00877672769905));
#9965=CARTESIAN_POINT('Ctrl Pts',(-0.03275519369704,300.176074056311,7.));
#9966=CARTESIAN_POINT('Ctrl Pts',(-1.9083995407149,300.313574056311,6.99122327230096));
#9967=CARTESIAN_POINT('Ctrl Pts',(-3.52836682984752,300.451074056311,6.04580022964255));
#9968=CARTESIAN_POINT('Ctrl Pts',(-5.14833411898014,300.588574056311,5.10037718698415));
#9969=CARTESIAN_POINT('Ctrl Pts',(-6.07855542333959,300.726074056311,3.47163317015249));
#9970=CARTESIAN_POINT('Ctrl Pts',(-7.00877672769905,300.863574056311,1.84288915332082));
#9971=CARTESIAN_POINT('Ctrl Pts',(-7.,301.001074056311,-0.0327551936970413));
#9972=CARTESIAN_POINT('Ctrl Pts',(-6.99122327230096,301.138574056311,-1.9083995407149));
#9973=CARTESIAN_POINT('Ctrl Pts',(-6.04580022964255,301.276074056311,-3.52836682984752));
#9974=CARTESIAN_POINT('Ctrl Pts',(-5.10037718698415,301.413574056311,-5.14833411898014));
#9975=CARTESIAN_POINT('Ctrl Pts',(-3.47163317015249,301.551074056311,-6.07855542333959));
#9976=CARTESIAN_POINT('Ctrl Pts',(-1.84288915332082,301.688574056311,-7.00877672769905));
#9977=CARTESIAN_POINT('Ctrl Pts',(0.0327551936970409,301.826074056311,-7.));
#9978=CARTESIAN_POINT('Ctrl Pts',(1.9083995407149,301.963574056311,-6.99122327230096));
#9979=CARTESIAN_POINT('Ctrl Pts',(3.52836682984752,302.101074056311,-6.04580022964255));
#9980=CARTESIAN_POINT('Ctrl Pts',(5.14833411898014,302.238574056311,-5.10037718698415));
#9981=CARTESIAN_POINT('Ctrl Pts',(6.07855542333959,302.376074056311,-3.47163317015249));
#9982=CARTESIAN_POINT('Ctrl Pts',(7.00877672769905,302.513574056311,-1.84288915332082));
#9983=CARTESIAN_POINT('Ctrl Pts',(7.,302.651074056311,0.0327551936970405));
#9984=CARTESIAN_POINT('Ctrl Pts',(6.99122327230096,302.788574056311,1.9083995407149));
#9985=CARTESIAN_POINT('Ctrl Pts',(6.04580022964255,302.926074056311,3.52836682984752));
#9986=CARTESIAN_POINT('Ctrl Pts',(5.10037718698415,303.063574056311,5.14833411898013));
#9987=CARTESIAN_POINT('Ctrl Pts',(3.47163317015249,303.201074056311,6.07855542333959));
#9988=CARTESIAN_POINT('Ctrl Pts',(1.84288915332082,303.338574056311,7.00877672769905));
#9989=CARTESIAN_POINT('Ctrl Pts',(-0.03275519369704,303.476074056311,7.));
#9990=CARTESIAN_POINT('Ctrl Pts',(-1.9083995407149,303.613574056311,6.99122327230096));
#9991=CARTESIAN_POINT('Ctrl Pts',(-3.52836682984752,303.751074056311,6.04580022964255));
#9992=CARTESIAN_POINT('Ctrl Pts',(-5.14833411898014,303.888574056311,5.10037718698415));
#9993=CARTESIAN_POINT('Ctrl Pts',(-6.07855542333959,304.026074056311,3.47163317015249));
#9994=CARTESIAN_POINT('Ctrl Pts',(-7.00877672769905,304.163574056311,1.84288915332082));
#9995=CARTESIAN_POINT('Ctrl Pts',(-7.,304.301074056311,-0.0327551936970413));
#9996=CARTESIAN_POINT('Ctrl Pts',(-6.99122327230096,304.438574056311,-1.9083995407149));
#9997=CARTESIAN_POINT('Ctrl Pts',(-6.04580022964255,304.576074056311,-3.52836682984752));
#9998=CARTESIAN_POINT('Ctrl Pts',(-5.10037718698415,304.713574056311,-5.14833411898014));
#9999=CARTESIAN_POINT('Ctrl Pts',(-3.47163317015249,304.851074056311,-6.07855542333959));
#10000=CARTESIAN_POINT('Ctrl Pts',(-1.84288915332082,304.988574056311,-7.00877672769905));
#10001=CARTESIAN_POINT('Ctrl Pts',(0.0327551936970409,305.126074056311,
-7.));
#10002=CARTESIAN_POINT('Ctrl Pts',(1.9083995407149,305.263574056311,-6.99122327230096));
#10003=CARTESIAN_POINT('Ctrl Pts',(3.52836682984752,305.401074056311,-6.04580022964255));
#10004=CARTESIAN_POINT('Ctrl Pts',(5.14833411898014,305.538574056311,-5.10037718698415));
#10005=CARTESIAN_POINT('Ctrl Pts',(6.07855542333959,305.676074056311,-3.47163317015249));
#10006=CARTESIAN_POINT('Ctrl Pts',(7.00877672769905,305.813574056311,-1.84288915332082));
#10007=CARTESIAN_POINT('Ctrl Pts',(7.,305.951074056311,0.0327551936970405));
#10008=CARTESIAN_POINT('Ctrl Pts',(6.99122327230096,306.088574056311,1.9083995407149));
#10009=CARTESIAN_POINT('Ctrl Pts',(6.04580022964255,306.226074056311,3.52836682984752));
#10010=CARTESIAN_POINT('Ctrl Pts',(5.10037718698415,306.363574056311,5.14833411898013));
#10011=CARTESIAN_POINT('Ctrl Pts',(3.47163317015249,306.501074056311,6.07855542333959));
#10012=CARTESIAN_POINT('Ctrl Pts',(1.84288915332082,306.638574056311,7.00877672769905));
#10013=CARTESIAN_POINT('Ctrl Pts',(-0.03275519369704,306.776074056311,7.));
#10014=CARTESIAN_POINT('Ctrl Pts',(-1.9083995407149,306.913574056311,6.99122327230096));
#10015=CARTESIAN_POINT('Ctrl Pts',(-3.52836682984752,307.051074056311,6.04580022964255));
#10016=CARTESIAN_POINT('Ctrl Pts',(-5.14833411898014,307.188574056311,5.10037718698415));
#10017=CARTESIAN_POINT('Ctrl Pts',(-6.07855542333959,307.326074056311,3.47163317015249));
#10018=CARTESIAN_POINT('Ctrl Pts',(-7.00877672769905,307.463574056311,1.84288915332082));
#10019=CARTESIAN_POINT('Ctrl Pts',(-7.,307.601074056311,-0.0327551936970413));
#10020=CARTESIAN_POINT('Ctrl Pts',(-6.99122327230096,307.738574056311,-1.9083995407149));
#10021=CARTESIAN_POINT('Ctrl Pts',(-6.04580022964255,307.876074056311,-3.52836682984752));
#10022=CARTESIAN_POINT('Ctrl Pts',(-5.10037718698415,308.013574056311,-5.14833411898014));
#10023=CARTESIAN_POINT('Ctrl Pts',(-3.47163317015249,308.151074056311,-6.07855542333959));
#10024=CARTESIAN_POINT('Ctrl Pts',(-1.84288915332082,308.288574056311,-7.00877672769905));
#10025=CARTESIAN_POINT('Ctrl Pts',(0.0327551936970409,308.426074056311,
-7.));
#10026=CARTESIAN_POINT('Ctrl Pts',(1.9083995407149,308.563574056311,-6.99122327230096));
#10027=CARTESIAN_POINT('Ctrl Pts',(3.52836682984752,308.701074056311,-6.04580022964255));
#10028=CARTESIAN_POINT('Ctrl Pts',(5.14833411898014,308.838574056311,-5.10037718698415));
#10029=CARTESIAN_POINT('Ctrl Pts',(6.07855542333959,308.976074056311,-3.47163317015249));
#10030=CARTESIAN_POINT('Ctrl Pts',(7.00877672769905,309.113574056311,-1.84288915332082));
#10031=CARTESIAN_POINT('Ctrl Pts',(7.,309.251074056311,0.0327551936970405));
#10032=CARTESIAN_POINT('Ctrl Pts',(6.99122327230096,309.388574056311,1.9083995407149));
#10033=CARTESIAN_POINT('Ctrl Pts',(6.04580022964255,309.526074056311,3.52836682984752));
#10034=CARTESIAN_POINT('Ctrl Pts',(5.10037718698415,309.663574056311,5.14833411898013));
#10035=CARTESIAN_POINT('Ctrl Pts',(3.47163317015249,309.801074056311,6.07855542333959));
#10036=CARTESIAN_POINT('Ctrl Pts',(1.84288915332082,309.938574056311,7.00877672769905));
#10037=CARTESIAN_POINT('Ctrl Pts',(-0.03275519369704,310.076074056311,7.));
#10038=CARTESIAN_POINT('Ctrl Pts',(-1.9083995407149,310.213574056311,6.99122327230096));
#10039=CARTESIAN_POINT('Ctrl Pts',(-3.52836682984752,310.351074056311,6.04580022964255));
#10040=CARTESIAN_POINT('Ctrl Pts',(-5.14833411898014,310.488574056311,5.10037718698415));
#10041=CARTESIAN_POINT('Ctrl Pts',(-6.07855542333959,310.626074056311,3.47163317015249));
#10042=CARTESIAN_POINT('Ctrl Pts',(-7.00877672769905,310.763574056311,1.84288915332082));
#10043=CARTESIAN_POINT('Ctrl Pts',(-7.,310.901074056311,-0.0327551936970413));
#10044=CARTESIAN_POINT('Ctrl Pts',(-6.99122327230096,311.038574056311,-1.9083995407149));
#10045=CARTESIAN_POINT('Ctrl Pts',(-6.04580022964255,311.176074056311,-3.52836682984752));
#10046=CARTESIAN_POINT('Ctrl Pts',(-5.10037718698415,311.313574056311,-5.14833411898014));
#10047=CARTESIAN_POINT('Ctrl Pts',(-3.47163317015249,311.451074056311,-6.07855542333959));
#10048=CARTESIAN_POINT('Ctrl Pts',(-1.84288915332082,311.588574056311,-7.00877672769905));
#10049=CARTESIAN_POINT('Ctrl Pts',(0.0327551936970409,311.726074056311,
-7.));
#10050=CARTESIAN_POINT('Ctrl Pts',(1.9083995407149,311.863574056311,-6.99122327230096));
#10051=CARTESIAN_POINT('Ctrl Pts',(3.52836682984752,312.001074056311,-6.04580022964255));
#10052=CARTESIAN_POINT('Ctrl Pts',(5.14833411898014,312.138574056311,-5.10037718698415));
#10053=CARTESIAN_POINT('Ctrl Pts',(6.07855542333959,312.276074056311,-3.47163317015249));
#10054=CARTESIAN_POINT('Ctrl Pts',(7.00877672769905,312.413574056311,-1.84288915332082));
#10055=CARTESIAN_POINT('Ctrl Pts',(7.,312.551074056311,0.0327551936970405));
#10056=CARTESIAN_POINT('Ctrl Pts',(6.99122327230096,312.688574056311,1.9083995407149));
#10057=CARTESIAN_POINT('Ctrl Pts',(6.04580022964255,312.826074056311,3.52836682984752));
#10058=CARTESIAN_POINT('Ctrl Pts',(5.10037718698415,312.963574056311,5.14833411898013));
#10059=CARTESIAN_POINT('Ctrl Pts',(3.47163317015249,313.101074056311,6.07855542333959));
#10060=CARTESIAN_POINT('Ctrl Pts',(1.84288915332082,313.238574056311,7.00877672769905));
#10061=CARTESIAN_POINT('Ctrl Pts',(-0.03275519369704,313.376074056311,7.));
#10062=CARTESIAN_POINT('Ctrl Pts',(-1.9083995407149,313.513574056311,6.99122327230096));
#10063=CARTESIAN_POINT('Ctrl Pts',(-3.52836682984752,313.651074056311,6.04580022964255));
#10064=CARTESIAN_POINT('Ctrl Pts',(-5.14833411898014,313.788574056311,5.10037718698415));
#10065=CARTESIAN_POINT('Ctrl Pts',(-6.07855542333959,313.926074056311,3.47163317015249));
#10066=CARTESIAN_POINT('Ctrl Pts',(-7.00877672769905,314.063574056311,1.84288915332082));
#10067=CARTESIAN_POINT('Ctrl Pts',(-7.,314.201074056311,-0.0327551936970413));
#10068=CARTESIAN_POINT('Ctrl Pts',(-6.99122327230096,314.338574056311,-1.9083995407149));
#10069=CARTESIAN_POINT('Ctrl Pts',(-6.04580022964255,314.476074056311,-3.52836682984752));
#10070=CARTESIAN_POINT('Ctrl Pts',(-5.10037718698415,314.613574056311,-5.14833411898014));
#10071=CARTESIAN_POINT('Ctrl Pts',(-3.47163317015249,314.751074056311,-6.07855542333959));
#10072=CARTESIAN_POINT('Ctrl Pts',(-1.84288915332082,314.888574056311,-7.00877672769905));
#10073=CARTESIAN_POINT('Ctrl Pts',(0.0327551936970409,315.026074056311,
-7.));
#10074=CARTESIAN_POINT('Ctrl Pts',(1.9083995407149,315.163574056311,-6.99122327230096));
#10075=CARTESIAN_POINT('Ctrl Pts',(3.52836682984752,315.301074056311,-6.04580022964255));
#10076=CARTESIAN_POINT('Ctrl Pts',(5.14833411898014,315.438574056311,-5.10037718698415));
#10077=CARTESIAN_POINT('Ctrl Pts',(6.07855542333959,315.576074056311,-3.47163317015249));
#10078=CARTESIAN_POINT('Ctrl Pts',(7.00877672769905,315.713574056311,-1.84288915332082));
#10079=CARTESIAN_POINT('Ctrl Pts',(7.,315.851074056311,0.0327551936970405));
#10080=CARTESIAN_POINT('Ctrl Pts',(6.99122327230096,315.988574056311,1.9083995407149));
#10081=CARTESIAN_POINT('Ctrl Pts',(6.04580022964255,316.126074056311,3.52836682984752));
#10082=CARTESIAN_POINT('Ctrl Pts',(5.10037718698415,316.263574056311,5.14833411898013));
#10083=CARTESIAN_POINT('Ctrl Pts',(3.47163317015249,316.401074056311,6.07855542333959));
#10084=CARTESIAN_POINT('Ctrl Pts',(1.84288915332082,316.538574056311,7.00877672769905));
#10085=CARTESIAN_POINT('Ctrl Pts',(-0.03275519369704,316.676074056311,7.));
#10086=CARTESIAN_POINT('Ctrl Pts',(-1.9083995407149,316.813574056311,6.99122327230096));
#10087=CARTESIAN_POINT('Ctrl Pts',(-3.52836682984752,316.951074056311,6.04580022964255));
#10088=CARTESIAN_POINT('Ctrl Pts',(-5.14833411898014,317.088574056311,5.10037718698415));
#10089=CARTESIAN_POINT('Ctrl Pts',(-6.07855542333959,317.226074056311,3.47163317015249));
#10090=CARTESIAN_POINT('Ctrl Pts',(-7.00877672769905,317.363574056311,1.84288915332082));
#10091=CARTESIAN_POINT('Ctrl Pts',(-7.,317.501074056311,-0.0327551936970413));
#10092=CARTESIAN_POINT('Ctrl Pts',(-8.,284.501074056311,-0.0327551936970314));
#10093=CARTESIAN_POINT('Ctrl Pts',(-7.99122327230096,284.638574056311,-2.17634873314601));
#10094=CARTESIAN_POINT('Ctrl Pts',(-6.911825633427,284.776074056311,-4.02836682984751));
#10095=CARTESIAN_POINT('Ctrl Pts',(-5.83242799455303,284.913574056311,-5.88038492654901));
#10096=CARTESIAN_POINT('Ctrl Pts',(-3.97163317015249,285.051074056311,-6.94458082712403));
#10097=CARTESIAN_POINT('Ctrl Pts',(-2.11083834575195,285.188574056311,-8.00877672769905));
#10098=CARTESIAN_POINT('Ctrl Pts',(0.0327551936970309,285.326074056311,
-8.));
#10099=CARTESIAN_POINT('Ctrl Pts',(2.17634873314601,285.463574056311,-7.99122327230096));
#10100=CARTESIAN_POINT('Ctrl Pts',(4.02836682984751,285.601074056311,-6.911825633427));
#10101=CARTESIAN_POINT('Ctrl Pts',(5.88038492654901,285.738574056311,-5.83242799455303));
#10102=CARTESIAN_POINT('Ctrl Pts',(6.94458082712403,285.876074056311,-3.9716331701525));
#10103=CARTESIAN_POINT('Ctrl Pts',(8.00877672769905,286.013574056311,-2.11083834575195));
#10104=CARTESIAN_POINT('Ctrl Pts',(8.,286.151074056311,0.0327551936970304));
#10105=CARTESIAN_POINT('Ctrl Pts',(7.99122327230096,286.288574056311,2.17634873314601));
#10106=CARTESIAN_POINT('Ctrl Pts',(6.911825633427,286.426074056311,4.02836682984751));
#10107=CARTESIAN_POINT('Ctrl Pts',(5.83242799455304,286.563574056311,5.880384926549));
#10108=CARTESIAN_POINT('Ctrl Pts',(3.9716331701525,286.701074056311,6.94458082712403));
#10109=CARTESIAN_POINT('Ctrl Pts',(2.11083834575196,286.838574056311,8.00877672769905));
#10110=CARTESIAN_POINT('Ctrl Pts',(-0.0327551936970299,286.976074056311,
8.));
#10111=CARTESIAN_POINT('Ctrl Pts',(-2.17634873314601,287.113574056311,7.99122327230096));
#10112=CARTESIAN_POINT('Ctrl Pts',(-4.02836682984751,287.251074056311,6.911825633427));
#10113=CARTESIAN_POINT('Ctrl Pts',(-5.88038492654901,287.388574056311,5.83242799455303));
#10114=CARTESIAN_POINT('Ctrl Pts',(-6.94458082712403,287.526074056311,3.9716331701525));
#10115=CARTESIAN_POINT('Ctrl Pts',(-8.00877672769905,287.663574056311,2.11083834575196));
#10116=CARTESIAN_POINT('Ctrl Pts',(-8.,287.801074056311,-0.0327551936970314));
#10117=CARTESIAN_POINT('Ctrl Pts',(-7.99122327230096,287.938574056311,-2.17634873314601));
#10118=CARTESIAN_POINT('Ctrl Pts',(-6.911825633427,288.076074056311,-4.02836682984751));
#10119=CARTESIAN_POINT('Ctrl Pts',(-5.83242799455303,288.213574056311,-5.88038492654901));
#10120=CARTESIAN_POINT('Ctrl Pts',(-3.97163317015249,288.351074056311,-6.94458082712403));
#10121=CARTESIAN_POINT('Ctrl Pts',(-2.11083834575195,288.488574056311,-8.00877672769905));
#10122=CARTESIAN_POINT('Ctrl Pts',(0.0327551936970309,288.626074056311,
-8.));
#10123=CARTESIAN_POINT('Ctrl Pts',(2.17634873314601,288.763574056311,-7.99122327230096));
#10124=CARTESIAN_POINT('Ctrl Pts',(4.02836682984751,288.901074056311,-6.911825633427));
#10125=CARTESIAN_POINT('Ctrl Pts',(5.88038492654901,289.038574056311,-5.83242799455303));
#10126=CARTESIAN_POINT('Ctrl Pts',(6.94458082712403,289.176074056311,-3.9716331701525));
#10127=CARTESIAN_POINT('Ctrl Pts',(8.00877672769905,289.313574056311,-2.11083834575195));
#10128=CARTESIAN_POINT('Ctrl Pts',(8.,289.451074056311,0.0327551936970304));
#10129=CARTESIAN_POINT('Ctrl Pts',(7.99122327230096,289.588574056311,2.17634873314601));
#10130=CARTESIAN_POINT('Ctrl Pts',(6.911825633427,289.726074056311,4.02836682984751));
#10131=CARTESIAN_POINT('Ctrl Pts',(5.83242799455304,289.863574056311,5.880384926549));
#10132=CARTESIAN_POINT('Ctrl Pts',(3.9716331701525,290.001074056311,6.94458082712403));
#10133=CARTESIAN_POINT('Ctrl Pts',(2.11083834575196,290.138574056311,8.00877672769905));
#10134=CARTESIAN_POINT('Ctrl Pts',(-0.0327551936970299,290.276074056311,
8.));
#10135=CARTESIAN_POINT('Ctrl Pts',(-2.17634873314601,290.413574056311,7.99122327230096));
#10136=CARTESIAN_POINT('Ctrl Pts',(-4.02836682984751,290.551074056311,6.911825633427));
#10137=CARTESIAN_POINT('Ctrl Pts',(-5.88038492654901,290.688574056311,5.83242799455303));
#10138=CARTESIAN_POINT('Ctrl Pts',(-6.94458082712403,290.826074056311,3.9716331701525));
#10139=CARTESIAN_POINT('Ctrl Pts',(-8.00877672769905,290.963574056311,2.11083834575196));
#10140=CARTESIAN_POINT('Ctrl Pts',(-8.,291.101074056311,-0.0327551936970314));
#10141=CARTESIAN_POINT('Ctrl Pts',(-7.99122327230096,291.238574056311,-2.17634873314601));
#10142=CARTESIAN_POINT('Ctrl Pts',(-6.911825633427,291.376074056311,-4.02836682984751));
#10143=CARTESIAN_POINT('Ctrl Pts',(-5.83242799455303,291.513574056311,-5.88038492654901));
#10144=CARTESIAN_POINT('Ctrl Pts',(-3.97163317015249,291.651074056311,-6.94458082712403));
#10145=CARTESIAN_POINT('Ctrl Pts',(-2.11083834575195,291.788574056311,-8.00877672769905));
#10146=CARTESIAN_POINT('Ctrl Pts',(0.0327551936970309,291.926074056311,
-8.));
#10147=CARTESIAN_POINT('Ctrl Pts',(2.17634873314601,292.063574056311,-7.99122327230096));
#10148=CARTESIAN_POINT('Ctrl Pts',(4.02836682984751,292.201074056311,-6.911825633427));
#10149=CARTESIAN_POINT('Ctrl Pts',(5.88038492654901,292.338574056311,-5.83242799455303));
#10150=CARTESIAN_POINT('Ctrl Pts',(6.94458082712403,292.476074056311,-3.9716331701525));
#10151=CARTESIAN_POINT('Ctrl Pts',(8.00877672769905,292.613574056311,-2.11083834575195));
#10152=CARTESIAN_POINT('Ctrl Pts',(8.,292.751074056311,0.0327551936970304));
#10153=CARTESIAN_POINT('Ctrl Pts',(7.99122327230096,292.888574056311,2.17634873314601));
#10154=CARTESIAN_POINT('Ctrl Pts',(6.911825633427,293.026074056311,4.02836682984751));
#10155=CARTESIAN_POINT('Ctrl Pts',(5.83242799455304,293.163574056311,5.880384926549));
#10156=CARTESIAN_POINT('Ctrl Pts',(3.9716331701525,293.301074056311,6.94458082712403));
#10157=CARTESIAN_POINT('Ctrl Pts',(2.11083834575196,293.438574056311,8.00877672769905));
#10158=CARTESIAN_POINT('Ctrl Pts',(-0.0327551936970299,293.576074056311,
8.));
#10159=CARTESIAN_POINT('Ctrl Pts',(-2.17634873314601,293.713574056311,7.99122327230096));
#10160=CARTESIAN_POINT('Ctrl Pts',(-4.02836682984751,293.851074056311,6.911825633427));
#10161=CARTESIAN_POINT('Ctrl Pts',(-5.88038492654901,293.988574056311,5.83242799455303));
#10162=CARTESIAN_POINT('Ctrl Pts',(-6.94458082712403,294.126074056311,3.9716331701525));
#10163=CARTESIAN_POINT('Ctrl Pts',(-8.00877672769905,294.263574056311,2.11083834575196));
#10164=CARTESIAN_POINT('Ctrl Pts',(-8.,294.401074056311,-0.0327551936970314));
#10165=CARTESIAN_POINT('Ctrl Pts',(-7.99122327230096,294.538574056311,-2.17634873314601));
#10166=CARTESIAN_POINT('Ctrl Pts',(-6.911825633427,294.676074056311,-4.02836682984751));
#10167=CARTESIAN_POINT('Ctrl Pts',(-5.83242799455303,294.813574056311,-5.88038492654901));
#10168=CARTESIAN_POINT('Ctrl Pts',(-3.97163317015249,294.951074056311,-6.94458082712403));
#10169=CARTESIAN_POINT('Ctrl Pts',(-2.11083834575195,295.088574056311,-8.00877672769905));
#10170=CARTESIAN_POINT('Ctrl Pts',(0.0327551936970309,295.226074056311,
-8.));
#10171=CARTESIAN_POINT('Ctrl Pts',(2.17634873314601,295.363574056311,-7.99122327230096));
#10172=CARTESIAN_POINT('Ctrl Pts',(4.02836682984751,295.501074056311,-6.911825633427));
#10173=CARTESIAN_POINT('Ctrl Pts',(5.88038492654901,295.638574056311,-5.83242799455303));
#10174=CARTESIAN_POINT('Ctrl Pts',(6.94458082712403,295.776074056311,-3.9716331701525));
#10175=CARTESIAN_POINT('Ctrl Pts',(8.00877672769905,295.913574056311,-2.11083834575195));
#10176=CARTESIAN_POINT('Ctrl Pts',(8.,296.051074056311,0.0327551936970304));
#10177=CARTESIAN_POINT('Ctrl Pts',(7.99122327230096,296.188574056311,2.17634873314601));
#10178=CARTESIAN_POINT('Ctrl Pts',(6.911825633427,296.326074056311,4.02836682984751));
#10179=CARTESIAN_POINT('Ctrl Pts',(5.83242799455304,296.463574056311,5.880384926549));
#10180=CARTESIAN_POINT('Ctrl Pts',(3.9716331701525,296.601074056311,6.94458082712403));
#10181=CARTESIAN_POINT('Ctrl Pts',(2.11083834575196,296.738574056311,8.00877672769905));
#10182=CARTESIAN_POINT('Ctrl Pts',(-0.0327551936970299,296.876074056311,
8.));
#10183=CARTESIAN_POINT('Ctrl Pts',(-2.17634873314601,297.013574056311,7.99122327230096));
#10184=CARTESIAN_POINT('Ctrl Pts',(-4.02836682984751,297.151074056311,6.911825633427));
#10185=CARTESIAN_POINT('Ctrl Pts',(-5.88038492654901,297.288574056311,5.83242799455303));
#10186=CARTESIAN_POINT('Ctrl Pts',(-6.94458082712403,297.426074056311,3.9716331701525));
#10187=CARTESIAN_POINT('Ctrl Pts',(-8.00877672769905,297.563574056311,2.11083834575196));
#10188=CARTESIAN_POINT('Ctrl Pts',(-8.,297.701074056311,-0.0327551936970314));
#10189=CARTESIAN_POINT('Ctrl Pts',(-7.99122327230096,297.838574056311,-2.17634873314601));
#10190=CARTESIAN_POINT('Ctrl Pts',(-6.911825633427,297.976074056311,-4.02836682984751));
#10191=CARTESIAN_POINT('Ctrl Pts',(-5.83242799455303,298.113574056311,-5.88038492654901));
#10192=CARTESIAN_POINT('Ctrl Pts',(-3.97163317015249,298.251074056311,-6.94458082712403));
#10193=CARTESIAN_POINT('Ctrl Pts',(-2.11083834575195,298.388574056311,-8.00877672769905));
#10194=CARTESIAN_POINT('Ctrl Pts',(0.0327551936970309,298.526074056311,
-8.));
#10195=CARTESIAN_POINT('Ctrl Pts',(2.17634873314601,298.663574056311,-7.99122327230096));
#10196=CARTESIAN_POINT('Ctrl Pts',(4.02836682984751,298.801074056311,-6.911825633427));
#10197=CARTESIAN_POINT('Ctrl Pts',(5.88038492654901,298.938574056311,-5.83242799455303));
#10198=CARTESIAN_POINT('Ctrl Pts',(6.94458082712403,299.076074056311,-3.9716331701525));
#10199=CARTESIAN_POINT('Ctrl Pts',(8.00877672769905,299.213574056311,-2.11083834575195));
#10200=CARTESIAN_POINT('Ctrl Pts',(8.,299.351074056311,0.0327551936970304));
#10201=CARTESIAN_POINT('Ctrl Pts',(7.99122327230096,299.488574056311,2.17634873314601));
#10202=CARTESIAN_POINT('Ctrl Pts',(6.911825633427,299.626074056311,4.02836682984751));
#10203=CARTESIAN_POINT('Ctrl Pts',(5.83242799455304,299.763574056311,5.880384926549));
#10204=CARTESIAN_POINT('Ctrl Pts',(3.9716331701525,299.901074056311,6.94458082712403));
#10205=CARTESIAN_POINT('Ctrl Pts',(2.11083834575196,300.038574056311,8.00877672769905));
#10206=CARTESIAN_POINT('Ctrl Pts',(-0.0327551936970299,300.176074056311,
8.));
#10207=CARTESIAN_POINT('Ctrl Pts',(-2.17634873314601,300.313574056311,7.99122327230096));
#10208=CARTESIAN_POINT('Ctrl Pts',(-4.02836682984751,300.451074056311,6.911825633427));
#10209=CARTESIAN_POINT('Ctrl Pts',(-5.88038492654901,300.588574056311,5.83242799455303));
#10210=CARTESIAN_POINT('Ctrl Pts',(-6.94458082712403,300.726074056311,3.9716331701525));
#10211=CARTESIAN_POINT('Ctrl Pts',(-8.00877672769905,300.863574056311,2.11083834575196));
#10212=CARTESIAN_POINT('Ctrl Pts',(-8.,301.001074056311,-0.0327551936970314));
#10213=CARTESIAN_POINT('Ctrl Pts',(-7.99122327230096,301.138574056311,-2.17634873314601));
#10214=CARTESIAN_POINT('Ctrl Pts',(-6.911825633427,301.276074056311,-4.02836682984751));
#10215=CARTESIAN_POINT('Ctrl Pts',(-5.83242799455303,301.413574056311,-5.88038492654901));
#10216=CARTESIAN_POINT('Ctrl Pts',(-3.97163317015249,301.551074056311,-6.94458082712403));
#10217=CARTESIAN_POINT('Ctrl Pts',(-2.11083834575195,301.688574056311,-8.00877672769905));
#10218=CARTESIAN_POINT('Ctrl Pts',(0.0327551936970309,301.826074056311,
-8.));
#10219=CARTESIAN_POINT('Ctrl Pts',(2.17634873314601,301.963574056311,-7.99122327230096));
#10220=CARTESIAN_POINT('Ctrl Pts',(4.02836682984751,302.101074056311,-6.911825633427));
#10221=CARTESIAN_POINT('Ctrl Pts',(5.88038492654901,302.238574056311,-5.83242799455303));
#10222=CARTESIAN_POINT('Ctrl Pts',(6.94458082712403,302.376074056311,-3.9716331701525));
#10223=CARTESIAN_POINT('Ctrl Pts',(8.00877672769905,302.513574056311,-2.11083834575195));
#10224=CARTESIAN_POINT('Ctrl Pts',(8.,302.651074056311,0.0327551936970304));
#10225=CARTESIAN_POINT('Ctrl Pts',(7.99122327230096,302.788574056311,2.17634873314601));
#10226=CARTESIAN_POINT('Ctrl Pts',(6.911825633427,302.926074056311,4.02836682984751));
#10227=CARTESIAN_POINT('Ctrl Pts',(5.83242799455304,303.063574056311,5.880384926549));
#10228=CARTESIAN_POINT('Ctrl Pts',(3.9716331701525,303.201074056311,6.94458082712403));
#10229=CARTESIAN_POINT('Ctrl Pts',(2.11083834575196,303.338574056311,8.00877672769905));
#10230=CARTESIAN_POINT('Ctrl Pts',(-0.0327551936970299,303.476074056311,
8.));
#10231=CARTESIAN_POINT('Ctrl Pts',(-2.17634873314601,303.613574056311,7.99122327230096));
#10232=CARTESIAN_POINT('Ctrl Pts',(-4.02836682984751,303.751074056311,6.911825633427));
#10233=CARTESIAN_POINT('Ctrl Pts',(-5.88038492654901,303.888574056311,5.83242799455303));
#10234=CARTESIAN_POINT('Ctrl Pts',(-6.94458082712403,304.026074056311,3.9716331701525));
#10235=CARTESIAN_POINT('Ctrl Pts',(-8.00877672769905,304.163574056311,2.11083834575196));
#10236=CARTESIAN_POINT('Ctrl Pts',(-8.,304.301074056311,-0.0327551936970314));
#10237=CARTESIAN_POINT('Ctrl Pts',(-7.99122327230096,304.438574056311,-2.17634873314601));
#10238=CARTESIAN_POINT('Ctrl Pts',(-6.911825633427,304.576074056311,-4.02836682984751));
#10239=CARTESIAN_POINT('Ctrl Pts',(-5.83242799455303,304.713574056311,-5.88038492654901));
#10240=CARTESIAN_POINT('Ctrl Pts',(-3.97163317015249,304.851074056311,-6.94458082712403));
#10241=CARTESIAN_POINT('Ctrl Pts',(-2.11083834575195,304.988574056311,-8.00877672769905));
#10242=CARTESIAN_POINT('Ctrl Pts',(0.0327551936970309,305.126074056311,
-8.));
#10243=CARTESIAN_POINT('Ctrl Pts',(2.17634873314601,305.263574056311,-7.99122327230096));
#10244=CARTESIAN_POINT('Ctrl Pts',(4.02836682984751,305.401074056311,-6.911825633427));
#10245=CARTESIAN_POINT('Ctrl Pts',(5.88038492654901,305.538574056311,-5.83242799455303));
#10246=CARTESIAN_POINT('Ctrl Pts',(6.94458082712403,305.676074056311,-3.9716331701525));
#10247=CARTESIAN_POINT('Ctrl Pts',(8.00877672769905,305.813574056311,-2.11083834575195));
#10248=CARTESIAN_POINT('Ctrl Pts',(8.,305.951074056311,0.0327551936970304));
#10249=CARTESIAN_POINT('Ctrl Pts',(7.99122327230096,306.088574056311,2.17634873314601));
#10250=CARTESIAN_POINT('Ctrl Pts',(6.911825633427,306.226074056311,4.02836682984751));
#10251=CARTESIAN_POINT('Ctrl Pts',(5.83242799455304,306.363574056311,5.880384926549));
#10252=CARTESIAN_POINT('Ctrl Pts',(3.9716331701525,306.501074056311,6.94458082712403));
#10253=CARTESIAN_POINT('Ctrl Pts',(2.11083834575196,306.638574056311,8.00877672769905));
#10254=CARTESIAN_POINT('Ctrl Pts',(-0.0327551936970299,306.776074056311,
8.));
#10255=CARTESIAN_POINT('Ctrl Pts',(-2.17634873314601,306.913574056311,7.99122327230096));
#10256=CARTESIAN_POINT('Ctrl Pts',(-4.02836682984751,307.051074056311,6.911825633427));
#10257=CARTESIAN_POINT('Ctrl Pts',(-5.88038492654901,307.188574056311,5.83242799455303));
#10258=CARTESIAN_POINT('Ctrl Pts',(-6.94458082712403,307.326074056311,3.9716331701525));
#10259=CARTESIAN_POINT('Ctrl Pts',(-8.00877672769905,307.463574056311,2.11083834575196));
#10260=CARTESIAN_POINT('Ctrl Pts',(-8.,307.601074056311,-0.0327551936970314));
#10261=CARTESIAN_POINT('Ctrl Pts',(-7.99122327230096,307.738574056311,-2.17634873314601));
#10262=CARTESIAN_POINT('Ctrl Pts',(-6.911825633427,307.876074056311,-4.02836682984751));
#10263=CARTESIAN_POINT('Ctrl Pts',(-5.83242799455303,308.013574056311,-5.88038492654901));
#10264=CARTESIAN_POINT('Ctrl Pts',(-3.97163317015249,308.151074056311,-6.94458082712403));
#10265=CARTESIAN_POINT('Ctrl Pts',(-2.11083834575195,308.288574056311,-8.00877672769905));
#10266=CARTESIAN_POINT('Ctrl Pts',(0.0327551936970309,308.426074056311,
-8.));
#10267=CARTESIAN_POINT('Ctrl Pts',(2.17634873314601,308.563574056311,-7.99122327230096));
#10268=CARTESIAN_POINT('Ctrl Pts',(4.02836682984751,308.701074056311,-6.911825633427));
#10269=CARTESIAN_POINT('Ctrl Pts',(5.88038492654901,308.838574056311,-5.83242799455303));
#10270=CARTESIAN_POINT('Ctrl Pts',(6.94458082712403,308.976074056311,-3.9716331701525));
#10271=CARTESIAN_POINT('Ctrl Pts',(8.00877672769905,309.113574056311,-2.11083834575195));
#10272=CARTESIAN_POINT('Ctrl Pts',(8.,309.251074056311,0.0327551936970304));
#10273=CARTESIAN_POINT('Ctrl Pts',(7.99122327230096,309.388574056311,2.17634873314601));
#10274=CARTESIAN_POINT('Ctrl Pts',(6.911825633427,309.526074056311,4.02836682984751));
#10275=CARTESIAN_POINT('Ctrl Pts',(5.83242799455304,309.663574056311,5.880384926549));
#10276=CARTESIAN_POINT('Ctrl Pts',(3.9716331701525,309.801074056311,6.94458082712403));
#10277=CARTESIAN_POINT('Ctrl Pts',(2.11083834575196,309.938574056311,8.00877672769905));
#10278=CARTESIAN_POINT('Ctrl Pts',(-0.0327551936970299,310.076074056311,
8.));
#10279=CARTESIAN_POINT('Ctrl Pts',(-2.17634873314601,310.213574056311,7.99122327230096));
#10280=CARTESIAN_POINT('Ctrl Pts',(-4.02836682984751,310.351074056311,6.911825633427));
#10281=CARTESIAN_POINT('Ctrl Pts',(-5.88038492654901,310.488574056311,5.83242799455303));
#10282=CARTESIAN_POINT('Ctrl Pts',(-6.94458082712403,310.626074056311,3.9716331701525));
#10283=CARTESIAN_POINT('Ctrl Pts',(-8.00877672769905,310.763574056311,2.11083834575196));
#10284=CARTESIAN_POINT('Ctrl Pts',(-8.,310.901074056311,-0.0327551936970314));
#10285=CARTESIAN_POINT('Ctrl Pts',(-7.99122327230096,311.038574056311,-2.17634873314601));
#10286=CARTESIAN_POINT('Ctrl Pts',(-6.911825633427,311.176074056311,-4.02836682984751));
#10287=CARTESIAN_POINT('Ctrl Pts',(-5.83242799455303,311.313574056311,-5.88038492654901));
#10288=CARTESIAN_POINT('Ctrl Pts',(-3.97163317015249,311.451074056311,-6.94458082712403));
#10289=CARTESIAN_POINT('Ctrl Pts',(-2.11083834575195,311.588574056311,-8.00877672769905));
#10290=CARTESIAN_POINT('Ctrl Pts',(0.0327551936970309,311.726074056311,
-8.));
#10291=CARTESIAN_POINT('Ctrl Pts',(2.17634873314601,311.863574056311,-7.99122327230096));
#10292=CARTESIAN_POINT('Ctrl Pts',(4.02836682984751,312.001074056311,-6.911825633427));
#10293=CARTESIAN_POINT('Ctrl Pts',(5.88038492654901,312.138574056311,-5.83242799455303));
#10294=CARTESIAN_POINT('Ctrl Pts',(6.94458082712403,312.276074056311,-3.9716331701525));
#10295=CARTESIAN_POINT('Ctrl Pts',(8.00877672769905,312.413574056311,-2.11083834575195));
#10296=CARTESIAN_POINT('Ctrl Pts',(8.,312.551074056311,0.0327551936970304));
#10297=CARTESIAN_POINT('Ctrl Pts',(7.99122327230096,312.688574056311,2.17634873314601));
#10298=CARTESIAN_POINT('Ctrl Pts',(6.911825633427,312.826074056311,4.02836682984751));
#10299=CARTESIAN_POINT('Ctrl Pts',(5.83242799455304,312.963574056311,5.880384926549));
#10300=CARTESIAN_POINT('Ctrl Pts',(3.9716331701525,313.101074056311,6.94458082712403));
#10301=CARTESIAN_POINT('Ctrl Pts',(2.11083834575196,313.238574056311,8.00877672769905));
#10302=CARTESIAN_POINT('Ctrl Pts',(-0.0327551936970299,313.376074056311,
8.));
#10303=CARTESIAN_POINT('Ctrl Pts',(-2.17634873314601,313.513574056311,7.99122327230096));
#10304=CARTESIAN_POINT('Ctrl Pts',(-4.02836682984751,313.651074056311,6.911825633427));
#10305=CARTESIAN_POINT('Ctrl Pts',(-5.88038492654901,313.788574056311,5.83242799455303));
#10306=CARTESIAN_POINT('Ctrl Pts',(-6.94458082712403,313.926074056311,3.9716331701525));
#10307=CARTESIAN_POINT('Ctrl Pts',(-8.00877672769905,314.063574056311,2.11083834575196));
#10308=CARTESIAN_POINT('Ctrl Pts',(-8.,314.201074056311,-0.0327551936970314));
#10309=CARTESIAN_POINT('Ctrl Pts',(-7.99122327230096,314.338574056311,-2.17634873314601));
#10310=CARTESIAN_POINT('Ctrl Pts',(-6.911825633427,314.476074056311,-4.02836682984751));
#10311=CARTESIAN_POINT('Ctrl Pts',(-5.83242799455303,314.613574056311,-5.88038492654901));
#10312=CARTESIAN_POINT('Ctrl Pts',(-3.97163317015249,314.751074056311,-6.94458082712403));
#10313=CARTESIAN_POINT('Ctrl Pts',(-2.11083834575195,314.888574056311,-8.00877672769905));
#10314=CARTESIAN_POINT('Ctrl Pts',(0.0327551936970309,315.026074056311,
-8.));
#10315=CARTESIAN_POINT('Ctrl Pts',(2.17634873314601,315.163574056311,-7.99122327230096));
#10316=CARTESIAN_POINT('Ctrl Pts',(4.02836682984751,315.301074056311,-6.911825633427));
#10317=CARTESIAN_POINT('Ctrl Pts',(5.88038492654901,315.438574056311,-5.83242799455303));
#10318=CARTESIAN_POINT('Ctrl Pts',(6.94458082712403,315.576074056311,-3.9716331701525));
#10319=CARTESIAN_POINT('Ctrl Pts',(8.00877672769905,315.713574056311,-2.11083834575195));
#10320=CARTESIAN_POINT('Ctrl Pts',(8.,315.851074056311,0.0327551936970304));
#10321=CARTESIAN_POINT('Ctrl Pts',(7.99122327230096,315.988574056311,2.17634873314601));
#10322=CARTESIAN_POINT('Ctrl Pts',(6.911825633427,316.126074056311,4.02836682984751));
#10323=CARTESIAN_POINT('Ctrl Pts',(5.83242799455304,316.263574056311,5.880384926549));
#10324=CARTESIAN_POINT('Ctrl Pts',(3.9716331701525,316.401074056311,6.94458082712403));
#10325=CARTESIAN_POINT('Ctrl Pts',(2.11083834575196,316.538574056311,8.00877672769905));
#10326=CARTESIAN_POINT('Ctrl Pts',(-0.0327551936970299,316.676074056311,
8.));
#10327=CARTESIAN_POINT('Ctrl Pts',(-2.17634873314601,316.813574056311,7.99122327230096));
#10328=CARTESIAN_POINT('Ctrl Pts',(-4.02836682984751,316.951074056311,6.911825633427));
#10329=CARTESIAN_POINT('Ctrl Pts',(-5.88038492654901,317.088574056311,5.83242799455303));
#10330=CARTESIAN_POINT('Ctrl Pts',(-6.94458082712403,317.226074056311,3.9716331701525));
#10331=CARTESIAN_POINT('Ctrl Pts',(-8.00877672769905,317.363574056311,2.11083834575196));
#10332=CARTESIAN_POINT('Ctrl Pts',(-8.,317.501074056311,-0.0327551936970314));
#10333=CARTESIAN_POINT('Ctrl Pts',(-9.,284.501074056311,-0.0327551936970214));
#10334=CARTESIAN_POINT('Ctrl Pts',(-8.99122327230096,284.638574056311,-2.44429792557713));
#10335=CARTESIAN_POINT('Ctrl Pts',(-7.77785103721144,284.776074056311,-4.5283668298475));
#10336=CARTESIAN_POINT('Ctrl Pts',(-6.56447880212192,284.913574056311,-6.61243573411788));
#10337=CARTESIAN_POINT('Ctrl Pts',(-4.4716331701525,285.051074056311,-7.81060623090846));
#10338=CARTESIAN_POINT('Ctrl Pts',(-2.37878753818309,285.188574056311,-9.00877672769904));
#10339=CARTESIAN_POINT('Ctrl Pts',(0.0327551936970209,285.326074056311,
-9.));
#10340=CARTESIAN_POINT('Ctrl Pts',(2.44429792557713,285.463574056311,-8.99122327230096));
#10341=CARTESIAN_POINT('Ctrl Pts',(4.5283668298475,285.601074056311,-7.77785103721144));
#10342=CARTESIAN_POINT('Ctrl Pts',(6.61243573411788,285.738574056311,-6.56447880212192));
#10343=CARTESIAN_POINT('Ctrl Pts',(7.81060623090846,285.876074056311,-4.4716331701525));
#10344=CARTESIAN_POINT('Ctrl Pts',(9.00877672769904,286.013574056311,-2.37878753818309));
#10345=CARTESIAN_POINT('Ctrl Pts',(9.,286.151074056311,0.0327551936970203));
#10346=CARTESIAN_POINT('Ctrl Pts',(8.99122327230096,286.288574056311,2.44429792557712));
#10347=CARTESIAN_POINT('Ctrl Pts',(7.77785103721144,286.426074056311,4.5283668298475));
#10348=CARTESIAN_POINT('Ctrl Pts',(6.56447880212192,286.563574056311,6.61243573411788));
#10349=CARTESIAN_POINT('Ctrl Pts',(4.47163317015251,286.701074056311,7.81060623090846));
#10350=CARTESIAN_POINT('Ctrl Pts',(2.37878753818309,286.838574056311,9.00877672769904));
#10351=CARTESIAN_POINT('Ctrl Pts',(-0.0327551936970198,286.976074056311,
9.));
#10352=CARTESIAN_POINT('Ctrl Pts',(-2.44429792557712,287.113574056311,8.99122327230096));
#10353=CARTESIAN_POINT('Ctrl Pts',(-4.5283668298475,287.251074056311,7.77785103721144));
#10354=CARTESIAN_POINT('Ctrl Pts',(-6.61243573411788,287.388574056311,6.56447880212192));
#10355=CARTESIAN_POINT('Ctrl Pts',(-7.81060623090846,287.526074056311,4.47163317015251));
#10356=CARTESIAN_POINT('Ctrl Pts',(-9.00877672769904,287.663574056311,2.37878753818309));
#10357=CARTESIAN_POINT('Ctrl Pts',(-9.,287.801074056311,-0.0327551936970214));
#10358=CARTESIAN_POINT('Ctrl Pts',(-8.99122327230096,287.938574056311,-2.44429792557713));
#10359=CARTESIAN_POINT('Ctrl Pts',(-7.77785103721144,288.076074056311,-4.5283668298475));
#10360=CARTESIAN_POINT('Ctrl Pts',(-6.56447880212192,288.213574056311,-6.61243573411788));
#10361=CARTESIAN_POINT('Ctrl Pts',(-4.4716331701525,288.351074056311,-7.81060623090846));
#10362=CARTESIAN_POINT('Ctrl Pts',(-2.37878753818309,288.488574056311,-9.00877672769904));
#10363=CARTESIAN_POINT('Ctrl Pts',(0.0327551936970209,288.626074056311,
-9.));
#10364=CARTESIAN_POINT('Ctrl Pts',(2.44429792557713,288.763574056311,-8.99122327230096));
#10365=CARTESIAN_POINT('Ctrl Pts',(4.5283668298475,288.901074056311,-7.77785103721144));
#10366=CARTESIAN_POINT('Ctrl Pts',(6.61243573411788,289.038574056311,-6.56447880212192));
#10367=CARTESIAN_POINT('Ctrl Pts',(7.81060623090846,289.176074056311,-4.4716331701525));
#10368=CARTESIAN_POINT('Ctrl Pts',(9.00877672769904,289.313574056311,-2.37878753818309));
#10369=CARTESIAN_POINT('Ctrl Pts',(9.,289.451074056311,0.0327551936970203));
#10370=CARTESIAN_POINT('Ctrl Pts',(8.99122327230096,289.588574056311,2.44429792557712));
#10371=CARTESIAN_POINT('Ctrl Pts',(7.77785103721144,289.726074056311,4.5283668298475));
#10372=CARTESIAN_POINT('Ctrl Pts',(6.56447880212192,289.863574056311,6.61243573411788));
#10373=CARTESIAN_POINT('Ctrl Pts',(4.47163317015251,290.001074056311,7.81060623090846));
#10374=CARTESIAN_POINT('Ctrl Pts',(2.37878753818309,290.138574056311,9.00877672769904));
#10375=CARTESIAN_POINT('Ctrl Pts',(-0.0327551936970198,290.276074056311,
9.));
#10376=CARTESIAN_POINT('Ctrl Pts',(-2.44429792557712,290.413574056311,8.99122327230096));
#10377=CARTESIAN_POINT('Ctrl Pts',(-4.5283668298475,290.551074056311,7.77785103721144));
#10378=CARTESIAN_POINT('Ctrl Pts',(-6.61243573411788,290.688574056311,6.56447880212192));
#10379=CARTESIAN_POINT('Ctrl Pts',(-7.81060623090846,290.826074056311,4.47163317015251));
#10380=CARTESIAN_POINT('Ctrl Pts',(-9.00877672769904,290.963574056311,2.37878753818309));
#10381=CARTESIAN_POINT('Ctrl Pts',(-9.,291.101074056311,-0.0327551936970214));
#10382=CARTESIAN_POINT('Ctrl Pts',(-8.99122327230096,291.238574056311,-2.44429792557713));
#10383=CARTESIAN_POINT('Ctrl Pts',(-7.77785103721144,291.376074056311,-4.5283668298475));
#10384=CARTESIAN_POINT('Ctrl Pts',(-6.56447880212192,291.513574056311,-6.61243573411788));
#10385=CARTESIAN_POINT('Ctrl Pts',(-4.4716331701525,291.651074056311,-7.81060623090846));
#10386=CARTESIAN_POINT('Ctrl Pts',(-2.37878753818309,291.788574056311,-9.00877672769904));
#10387=CARTESIAN_POINT('Ctrl Pts',(0.0327551936970209,291.926074056311,
-9.));
#10388=CARTESIAN_POINT('Ctrl Pts',(2.44429792557713,292.063574056311,-8.99122327230096));
#10389=CARTESIAN_POINT('Ctrl Pts',(4.5283668298475,292.201074056311,-7.77785103721144));
#10390=CARTESIAN_POINT('Ctrl Pts',(6.61243573411788,292.338574056311,-6.56447880212192));
#10391=CARTESIAN_POINT('Ctrl Pts',(7.81060623090846,292.476074056311,-4.4716331701525));
#10392=CARTESIAN_POINT('Ctrl Pts',(9.00877672769904,292.613574056311,-2.37878753818309));
#10393=CARTESIAN_POINT('Ctrl Pts',(9.,292.751074056311,0.0327551936970203));
#10394=CARTESIAN_POINT('Ctrl Pts',(8.99122327230096,292.888574056311,2.44429792557712));
#10395=CARTESIAN_POINT('Ctrl Pts',(7.77785103721144,293.026074056311,4.5283668298475));
#10396=CARTESIAN_POINT('Ctrl Pts',(6.56447880212192,293.163574056311,6.61243573411788));
#10397=CARTESIAN_POINT('Ctrl Pts',(4.47163317015251,293.301074056311,7.81060623090846));
#10398=CARTESIAN_POINT('Ctrl Pts',(2.37878753818309,293.438574056311,9.00877672769904));
#10399=CARTESIAN_POINT('Ctrl Pts',(-0.0327551936970198,293.576074056311,
9.));
#10400=CARTESIAN_POINT('Ctrl Pts',(-2.44429792557712,293.713574056311,8.99122327230096));
#10401=CARTESIAN_POINT('Ctrl Pts',(-4.5283668298475,293.851074056311,7.77785103721144));
#10402=CARTESIAN_POINT('Ctrl Pts',(-6.61243573411788,293.988574056311,6.56447880212192));
#10403=CARTESIAN_POINT('Ctrl Pts',(-7.81060623090846,294.126074056311,4.47163317015251));
#10404=CARTESIAN_POINT('Ctrl Pts',(-9.00877672769904,294.263574056311,2.37878753818309));
#10405=CARTESIAN_POINT('Ctrl Pts',(-9.,294.401074056311,-0.0327551936970214));
#10406=CARTESIAN_POINT('Ctrl Pts',(-8.99122327230096,294.538574056311,-2.44429792557713));
#10407=CARTESIAN_POINT('Ctrl Pts',(-7.77785103721144,294.676074056311,-4.5283668298475));
#10408=CARTESIAN_POINT('Ctrl Pts',(-6.56447880212192,294.813574056311,-6.61243573411788));
#10409=CARTESIAN_POINT('Ctrl Pts',(-4.4716331701525,294.951074056311,-7.81060623090846));
#10410=CARTESIAN_POINT('Ctrl Pts',(-2.37878753818309,295.088574056311,-9.00877672769904));
#10411=CARTESIAN_POINT('Ctrl Pts',(0.0327551936970209,295.226074056311,
-9.));
#10412=CARTESIAN_POINT('Ctrl Pts',(2.44429792557713,295.363574056311,-8.99122327230096));
#10413=CARTESIAN_POINT('Ctrl Pts',(4.5283668298475,295.501074056311,-7.77785103721144));
#10414=CARTESIAN_POINT('Ctrl Pts',(6.61243573411788,295.638574056311,-6.56447880212192));
#10415=CARTESIAN_POINT('Ctrl Pts',(7.81060623090846,295.776074056311,-4.4716331701525));
#10416=CARTESIAN_POINT('Ctrl Pts',(9.00877672769904,295.913574056311,-2.37878753818309));
#10417=CARTESIAN_POINT('Ctrl Pts',(9.,296.051074056311,0.0327551936970203));
#10418=CARTESIAN_POINT('Ctrl Pts',(8.99122327230096,296.188574056311,2.44429792557712));
#10419=CARTESIAN_POINT('Ctrl Pts',(7.77785103721144,296.326074056311,4.5283668298475));
#10420=CARTESIAN_POINT('Ctrl Pts',(6.56447880212192,296.463574056311,6.61243573411788));
#10421=CARTESIAN_POINT('Ctrl Pts',(4.47163317015251,296.601074056311,7.81060623090846));
#10422=CARTESIAN_POINT('Ctrl Pts',(2.37878753818309,296.738574056311,9.00877672769904));
#10423=CARTESIAN_POINT('Ctrl Pts',(-0.0327551936970198,296.876074056311,
9.));
#10424=CARTESIAN_POINT('Ctrl Pts',(-2.44429792557712,297.013574056311,8.99122327230096));
#10425=CARTESIAN_POINT('Ctrl Pts',(-4.5283668298475,297.151074056311,7.77785103721144));
#10426=CARTESIAN_POINT('Ctrl Pts',(-6.61243573411788,297.288574056311,6.56447880212192));
#10427=CARTESIAN_POINT('Ctrl Pts',(-7.81060623090846,297.426074056311,4.47163317015251));
#10428=CARTESIAN_POINT('Ctrl Pts',(-9.00877672769904,297.563574056311,2.37878753818309));
#10429=CARTESIAN_POINT('Ctrl Pts',(-9.,297.701074056311,-0.0327551936970214));
#10430=CARTESIAN_POINT('Ctrl Pts',(-8.99122327230096,297.838574056311,-2.44429792557713));
#10431=CARTESIAN_POINT('Ctrl Pts',(-7.77785103721144,297.976074056311,-4.5283668298475));
#10432=CARTESIAN_POINT('Ctrl Pts',(-6.56447880212192,298.113574056311,-6.61243573411788));
#10433=CARTESIAN_POINT('Ctrl Pts',(-4.4716331701525,298.251074056311,-7.81060623090846));
#10434=CARTESIAN_POINT('Ctrl Pts',(-2.37878753818309,298.388574056311,-9.00877672769904));
#10435=CARTESIAN_POINT('Ctrl Pts',(0.0327551936970209,298.526074056311,
-9.));
#10436=CARTESIAN_POINT('Ctrl Pts',(2.44429792557713,298.663574056311,-8.99122327230096));
#10437=CARTESIAN_POINT('Ctrl Pts',(4.5283668298475,298.801074056311,-7.77785103721144));
#10438=CARTESIAN_POINT('Ctrl Pts',(6.61243573411788,298.938574056311,-6.56447880212192));
#10439=CARTESIAN_POINT('Ctrl Pts',(7.81060623090846,299.076074056311,-4.4716331701525));
#10440=CARTESIAN_POINT('Ctrl Pts',(9.00877672769904,299.213574056311,-2.37878753818309));
#10441=CARTESIAN_POINT('Ctrl Pts',(9.,299.351074056311,0.0327551936970203));
#10442=CARTESIAN_POINT('Ctrl Pts',(8.99122327230096,299.488574056311,2.44429792557712));
#10443=CARTESIAN_POINT('Ctrl Pts',(7.77785103721144,299.626074056311,4.5283668298475));
#10444=CARTESIAN_POINT('Ctrl Pts',(6.56447880212192,299.763574056311,6.61243573411788));
#10445=CARTESIAN_POINT('Ctrl Pts',(4.47163317015251,299.901074056311,7.81060623090846));
#10446=CARTESIAN_POINT('Ctrl Pts',(2.37878753818309,300.038574056311,9.00877672769904));
#10447=CARTESIAN_POINT('Ctrl Pts',(-0.0327551936970198,300.176074056311,
9.));
#10448=CARTESIAN_POINT('Ctrl Pts',(-2.44429792557712,300.313574056311,8.99122327230096));
#10449=CARTESIAN_POINT('Ctrl Pts',(-4.5283668298475,300.451074056311,7.77785103721144));
#10450=CARTESIAN_POINT('Ctrl Pts',(-6.61243573411788,300.588574056311,6.56447880212192));
#10451=CARTESIAN_POINT('Ctrl Pts',(-7.81060623090846,300.726074056311,4.47163317015251));
#10452=CARTESIAN_POINT('Ctrl Pts',(-9.00877672769904,300.863574056311,2.37878753818309));
#10453=CARTESIAN_POINT('Ctrl Pts',(-9.,301.001074056311,-0.0327551936970214));
#10454=CARTESIAN_POINT('Ctrl Pts',(-8.99122327230096,301.138574056311,-2.44429792557713));
#10455=CARTESIAN_POINT('Ctrl Pts',(-7.77785103721144,301.276074056311,-4.5283668298475));
#10456=CARTESIAN_POINT('Ctrl Pts',(-6.56447880212192,301.413574056311,-6.61243573411788));
#10457=CARTESIAN_POINT('Ctrl Pts',(-4.4716331701525,301.551074056311,-7.81060623090846));
#10458=CARTESIAN_POINT('Ctrl Pts',(-2.37878753818309,301.688574056311,-9.00877672769904));
#10459=CARTESIAN_POINT('Ctrl Pts',(0.0327551936970209,301.826074056311,
-9.));
#10460=CARTESIAN_POINT('Ctrl Pts',(2.44429792557713,301.963574056311,-8.99122327230096));
#10461=CARTESIAN_POINT('Ctrl Pts',(4.5283668298475,302.101074056311,-7.77785103721144));
#10462=CARTESIAN_POINT('Ctrl Pts',(6.61243573411788,302.238574056311,-6.56447880212192));
#10463=CARTESIAN_POINT('Ctrl Pts',(7.81060623090846,302.376074056311,-4.4716331701525));
#10464=CARTESIAN_POINT('Ctrl Pts',(9.00877672769904,302.513574056311,-2.37878753818309));
#10465=CARTESIAN_POINT('Ctrl Pts',(9.,302.651074056311,0.0327551936970203));
#10466=CARTESIAN_POINT('Ctrl Pts',(8.99122327230096,302.788574056311,2.44429792557712));
#10467=CARTESIAN_POINT('Ctrl Pts',(7.77785103721144,302.926074056311,4.5283668298475));
#10468=CARTESIAN_POINT('Ctrl Pts',(6.56447880212192,303.063574056311,6.61243573411788));
#10469=CARTESIAN_POINT('Ctrl Pts',(4.47163317015251,303.201074056311,7.81060623090846));
#10470=CARTESIAN_POINT('Ctrl Pts',(2.37878753818309,303.338574056311,9.00877672769904));
#10471=CARTESIAN_POINT('Ctrl Pts',(-0.0327551936970198,303.476074056311,
9.));
#10472=CARTESIAN_POINT('Ctrl Pts',(-2.44429792557712,303.613574056311,8.99122327230096));
#10473=CARTESIAN_POINT('Ctrl Pts',(-4.5283668298475,303.751074056311,7.77785103721144));
#10474=CARTESIAN_POINT('Ctrl Pts',(-6.61243573411788,303.888574056311,6.56447880212192));
#10475=CARTESIAN_POINT('Ctrl Pts',(-7.81060623090846,304.026074056311,4.47163317015251));
#10476=CARTESIAN_POINT('Ctrl Pts',(-9.00877672769904,304.163574056311,2.37878753818309));
#10477=CARTESIAN_POINT('Ctrl Pts',(-9.,304.301074056311,-0.0327551936970214));
#10478=CARTESIAN_POINT('Ctrl Pts',(-8.99122327230096,304.438574056311,-2.44429792557713));
#10479=CARTESIAN_POINT('Ctrl Pts',(-7.77785103721144,304.576074056311,-4.5283668298475));
#10480=CARTESIAN_POINT('Ctrl Pts',(-6.56447880212192,304.713574056311,-6.61243573411788));
#10481=CARTESIAN_POINT('Ctrl Pts',(-4.4716331701525,304.851074056311,-7.81060623090846));
#10482=CARTESIAN_POINT('Ctrl Pts',(-2.37878753818309,304.988574056311,-9.00877672769904));
#10483=CARTESIAN_POINT('Ctrl Pts',(0.0327551936970209,305.126074056311,
-9.));
#10484=CARTESIAN_POINT('Ctrl Pts',(2.44429792557713,305.263574056311,-8.99122327230096));
#10485=CARTESIAN_POINT('Ctrl Pts',(4.5283668298475,305.401074056311,-7.77785103721144));
#10486=CARTESIAN_POINT('Ctrl Pts',(6.61243573411788,305.538574056311,-6.56447880212192));
#10487=CARTESIAN_POINT('Ctrl Pts',(7.81060623090846,305.676074056311,-4.4716331701525));
#10488=CARTESIAN_POINT('Ctrl Pts',(9.00877672769904,305.813574056311,-2.37878753818309));
#10489=CARTESIAN_POINT('Ctrl Pts',(9.,305.951074056311,0.0327551936970203));
#10490=CARTESIAN_POINT('Ctrl Pts',(8.99122327230096,306.088574056311,2.44429792557712));
#10491=CARTESIAN_POINT('Ctrl Pts',(7.77785103721144,306.226074056311,4.5283668298475));
#10492=CARTESIAN_POINT('Ctrl Pts',(6.56447880212192,306.363574056311,6.61243573411788));
#10493=CARTESIAN_POINT('Ctrl Pts',(4.47163317015251,306.501074056311,7.81060623090846));
#10494=CARTESIAN_POINT('Ctrl Pts',(2.37878753818309,306.638574056311,9.00877672769904));
#10495=CARTESIAN_POINT('Ctrl Pts',(-0.0327551936970198,306.776074056311,
9.));
#10496=CARTESIAN_POINT('Ctrl Pts',(-2.44429792557712,306.913574056311,8.99122327230096));
#10497=CARTESIAN_POINT('Ctrl Pts',(-4.5283668298475,307.051074056311,7.77785103721144));
#10498=CARTESIAN_POINT('Ctrl Pts',(-6.61243573411788,307.188574056311,6.56447880212192));
#10499=CARTESIAN_POINT('Ctrl Pts',(-7.81060623090846,307.326074056311,4.47163317015251));
#10500=CARTESIAN_POINT('Ctrl Pts',(-9.00877672769904,307.463574056311,2.37878753818309));
#10501=CARTESIAN_POINT('Ctrl Pts',(-9.,307.601074056311,-0.0327551936970214));
#10502=CARTESIAN_POINT('Ctrl Pts',(-8.99122327230096,307.738574056311,-2.44429792557713));
#10503=CARTESIAN_POINT('Ctrl Pts',(-7.77785103721144,307.876074056311,-4.5283668298475));
#10504=CARTESIAN_POINT('Ctrl Pts',(-6.56447880212192,308.013574056311,-6.61243573411788));
#10505=CARTESIAN_POINT('Ctrl Pts',(-4.4716331701525,308.151074056311,-7.81060623090846));
#10506=CARTESIAN_POINT('Ctrl Pts',(-2.37878753818309,308.288574056311,-9.00877672769904));
#10507=CARTESIAN_POINT('Ctrl Pts',(0.0327551936970209,308.426074056311,
-9.));
#10508=CARTESIAN_POINT('Ctrl Pts',(2.44429792557713,308.563574056311,-8.99122327230096));
#10509=CARTESIAN_POINT('Ctrl Pts',(4.5283668298475,308.701074056311,-7.77785103721144));
#10510=CARTESIAN_POINT('Ctrl Pts',(6.61243573411788,308.838574056311,-6.56447880212192));
#10511=CARTESIAN_POINT('Ctrl Pts',(7.81060623090846,308.976074056311,-4.4716331701525));
#10512=CARTESIAN_POINT('Ctrl Pts',(9.00877672769904,309.113574056311,-2.37878753818309));
#10513=CARTESIAN_POINT('Ctrl Pts',(9.,309.251074056311,0.0327551936970203));
#10514=CARTESIAN_POINT('Ctrl Pts',(8.99122327230096,309.388574056311,2.44429792557712));
#10515=CARTESIAN_POINT('Ctrl Pts',(7.77785103721144,309.526074056311,4.5283668298475));
#10516=CARTESIAN_POINT('Ctrl Pts',(6.56447880212192,309.663574056311,6.61243573411788));
#10517=CARTESIAN_POINT('Ctrl Pts',(4.47163317015251,309.801074056311,7.81060623090846));
#10518=CARTESIAN_POINT('Ctrl Pts',(2.37878753818309,309.938574056311,9.00877672769904));
#10519=CARTESIAN_POINT('Ctrl Pts',(-0.0327551936970198,310.076074056311,
9.));
#10520=CARTESIAN_POINT('Ctrl Pts',(-2.44429792557712,310.213574056311,8.99122327230096));
#10521=CARTESIAN_POINT('Ctrl Pts',(-4.5283668298475,310.351074056311,7.77785103721144));
#10522=CARTESIAN_POINT('Ctrl Pts',(-6.61243573411788,310.488574056311,6.56447880212192));
#10523=CARTESIAN_POINT('Ctrl Pts',(-7.81060623090846,310.626074056311,4.47163317015251));
#10524=CARTESIAN_POINT('Ctrl Pts',(-9.00877672769904,310.763574056311,2.37878753818309));
#10525=CARTESIAN_POINT('Ctrl Pts',(-9.,310.901074056311,-0.0327551936970214));
#10526=CARTESIAN_POINT('Ctrl Pts',(-8.99122327230096,311.038574056311,-2.44429792557713));
#10527=CARTESIAN_POINT('Ctrl Pts',(-7.77785103721144,311.176074056311,-4.5283668298475));
#10528=CARTESIAN_POINT('Ctrl Pts',(-6.56447880212192,311.313574056311,-6.61243573411788));
#10529=CARTESIAN_POINT('Ctrl Pts',(-4.4716331701525,311.451074056311,-7.81060623090846));
#10530=CARTESIAN_POINT('Ctrl Pts',(-2.37878753818309,311.588574056311,-9.00877672769904));
#10531=CARTESIAN_POINT('Ctrl Pts',(0.0327551936970209,311.726074056311,
-9.));
#10532=CARTESIAN_POINT('Ctrl Pts',(2.44429792557713,311.863574056311,-8.99122327230096));
#10533=CARTESIAN_POINT('Ctrl Pts',(4.5283668298475,312.001074056311,-7.77785103721144));
#10534=CARTESIAN_POINT('Ctrl Pts',(6.61243573411788,312.138574056311,-6.56447880212192));
#10535=CARTESIAN_POINT('Ctrl Pts',(7.81060623090846,312.276074056311,-4.4716331701525));
#10536=CARTESIAN_POINT('Ctrl Pts',(9.00877672769904,312.413574056311,-2.37878753818309));
#10537=CARTESIAN_POINT('Ctrl Pts',(9.,312.551074056311,0.0327551936970203));
#10538=CARTESIAN_POINT('Ctrl Pts',(8.99122327230096,312.688574056311,2.44429792557712));
#10539=CARTESIAN_POINT('Ctrl Pts',(7.77785103721144,312.826074056311,4.5283668298475));
#10540=CARTESIAN_POINT('Ctrl Pts',(6.56447880212192,312.963574056311,6.61243573411788));
#10541=CARTESIAN_POINT('Ctrl Pts',(4.47163317015251,313.101074056311,7.81060623090846));
#10542=CARTESIAN_POINT('Ctrl Pts',(2.37878753818309,313.238574056311,9.00877672769904));
#10543=CARTESIAN_POINT('Ctrl Pts',(-0.0327551936970198,313.376074056311,
9.));
#10544=CARTESIAN_POINT('Ctrl Pts',(-2.44429792557712,313.513574056311,8.99122327230096));
#10545=CARTESIAN_POINT('Ctrl Pts',(-4.5283668298475,313.651074056311,7.77785103721144));
#10546=CARTESIAN_POINT('Ctrl Pts',(-6.61243573411788,313.788574056311,6.56447880212192));
#10547=CARTESIAN_POINT('Ctrl Pts',(-7.81060623090846,313.926074056311,4.47163317015251));
#10548=CARTESIAN_POINT('Ctrl Pts',(-9.00877672769904,314.063574056311,2.37878753818309));
#10549=CARTESIAN_POINT('Ctrl Pts',(-9.,314.201074056311,-0.0327551936970214));
#10550=CARTESIAN_POINT('Ctrl Pts',(-8.99122327230096,314.338574056311,-2.44429792557713));
#10551=CARTESIAN_POINT('Ctrl Pts',(-7.77785103721144,314.476074056311,-4.5283668298475));
#10552=CARTESIAN_POINT('Ctrl Pts',(-6.56447880212192,314.613574056311,-6.61243573411788));
#10553=CARTESIAN_POINT('Ctrl Pts',(-4.4716331701525,314.751074056311,-7.81060623090846));
#10554=CARTESIAN_POINT('Ctrl Pts',(-2.37878753818309,314.888574056311,-9.00877672769904));
#10555=CARTESIAN_POINT('Ctrl Pts',(0.0327551936970209,315.026074056311,
-9.));
#10556=CARTESIAN_POINT('Ctrl Pts',(2.44429792557713,315.163574056311,-8.99122327230096));
#10557=CARTESIAN_POINT('Ctrl Pts',(4.5283668298475,315.301074056311,-7.77785103721144));
#10558=CARTESIAN_POINT('Ctrl Pts',(6.61243573411788,315.438574056311,-6.56447880212192));
#10559=CARTESIAN_POINT('Ctrl Pts',(7.81060623090846,315.576074056311,-4.4716331701525));
#10560=CARTESIAN_POINT('Ctrl Pts',(9.00877672769904,315.713574056311,-2.37878753818309));
#10561=CARTESIAN_POINT('Ctrl Pts',(9.,315.851074056311,0.0327551936970203));
#10562=CARTESIAN_POINT('Ctrl Pts',(8.99122327230096,315.988574056311,2.44429792557712));
#10563=CARTESIAN_POINT('Ctrl Pts',(7.77785103721144,316.126074056311,4.5283668298475));
#10564=CARTESIAN_POINT('Ctrl Pts',(6.56447880212192,316.263574056311,6.61243573411788));
#10565=CARTESIAN_POINT('Ctrl Pts',(4.47163317015251,316.401074056311,7.81060623090846));
#10566=CARTESIAN_POINT('Ctrl Pts',(2.37878753818309,316.538574056311,9.00877672769904));
#10567=CARTESIAN_POINT('Ctrl Pts',(-0.0327551936970198,316.676074056311,
9.));
#10568=CARTESIAN_POINT('Ctrl Pts',(-2.44429792557712,316.813574056311,8.99122327230096));
#10569=CARTESIAN_POINT('Ctrl Pts',(-4.5283668298475,316.951074056311,7.77785103721144));
#10570=CARTESIAN_POINT('Ctrl Pts',(-6.61243573411788,317.088574056311,6.56447880212192));
#10571=CARTESIAN_POINT('Ctrl Pts',(-7.81060623090846,317.226074056311,4.47163317015251));
#10572=CARTESIAN_POINT('Ctrl Pts',(-9.00877672769904,317.363574056311,2.37878753818309));
#10573=CARTESIAN_POINT('Ctrl Pts',(-9.,317.501074056311,-0.0327551936970214));
#10574=CARTESIAN_POINT('Ctrl Pts',(-9.,285.498925943689,0.0327551936972079));
#10575=CARTESIAN_POINT('Ctrl Pts',(-9.0087767276991,285.636425943689,-2.3787875381829));
#10576=CARTESIAN_POINT('Ctrl Pts',(-7.81060623090856,285.773925943689,-4.47163317015234));
#10577=CARTESIAN_POINT('Ctrl Pts',(-6.61243573411802,285.911425943689,-6.56447880212179));
#10578=CARTESIAN_POINT('Ctrl Pts',(-4.52836682984766,286.048925943689,-7.77785103721135));
#10579=CARTESIAN_POINT('Ctrl Pts',(-2.44429792557731,286.186425943689,-8.99122327230091));
#10580=CARTESIAN_POINT('Ctrl Pts',(-0.0327551936972084,286.323925943689,
-9.));
#10581=CARTESIAN_POINT('Ctrl Pts',(2.3787875381829,286.461425943689,-9.0087767276991));
#10582=CARTESIAN_POINT('Ctrl Pts',(4.47163317015234,286.598925943689,-7.81060623090856));
#10583=CARTESIAN_POINT('Ctrl Pts',(6.56447880212178,286.736425943689,-6.61243573411802));
#10584=CARTESIAN_POINT('Ctrl Pts',(7.77785103721135,286.873925943689,-4.52836682984767));
#10585=CARTESIAN_POINT('Ctrl Pts',(8.99122327230091,287.011425943689,-2.44429792557732));
#10586=CARTESIAN_POINT('Ctrl Pts',(9.,287.148925943689,-0.032755193697209));
#10587=CARTESIAN_POINT('Ctrl Pts',(9.0087767276991,287.286425943689,2.37878753818289));
#10588=CARTESIAN_POINT('Ctrl Pts',(7.81060623090856,287.423925943689,4.47163317015234));
#10589=CARTESIAN_POINT('Ctrl Pts',(6.61243573411802,287.561425943689,6.56447880212178));
#10590=CARTESIAN_POINT('Ctrl Pts',(4.52836682984767,287.698925943689,7.77785103721135));
#10591=CARTESIAN_POINT('Ctrl Pts',(2.44429792557732,287.836425943689,8.99122327230091));
#10592=CARTESIAN_POINT('Ctrl Pts',(0.0327551936972095,287.973925943689,
9.));
#10593=CARTESIAN_POINT('Ctrl Pts',(-2.37878753818289,288.111425943689,9.0087767276991));
#10594=CARTESIAN_POINT('Ctrl Pts',(-4.47163317015233,288.248925943689,7.81060623090856));
#10595=CARTESIAN_POINT('Ctrl Pts',(-6.56447880212178,288.386425943689,6.61243573411802));
#10596=CARTESIAN_POINT('Ctrl Pts',(-7.77785103721135,288.523925943689,4.52836682984767));
#10597=CARTESIAN_POINT('Ctrl Pts',(-8.99122327230091,288.661425943689,2.44429792557732));
#10598=CARTESIAN_POINT('Ctrl Pts',(-9.,288.798925943689,0.0327551936972079));
#10599=CARTESIAN_POINT('Ctrl Pts',(-9.0087767276991,288.936425943689,-2.3787875381829));
#10600=CARTESIAN_POINT('Ctrl Pts',(-7.81060623090856,289.073925943689,-4.47163317015234));
#10601=CARTESIAN_POINT('Ctrl Pts',(-6.61243573411802,289.211425943689,-6.56447880212179));
#10602=CARTESIAN_POINT('Ctrl Pts',(-4.52836682984766,289.348925943689,-7.77785103721135));
#10603=CARTESIAN_POINT('Ctrl Pts',(-2.44429792557731,289.486425943689,-8.99122327230091));
#10604=CARTESIAN_POINT('Ctrl Pts',(-0.0327551936972084,289.623925943689,
-9.));
#10605=CARTESIAN_POINT('Ctrl Pts',(2.3787875381829,289.761425943689,-9.0087767276991));
#10606=CARTESIAN_POINT('Ctrl Pts',(4.47163317015234,289.898925943689,-7.81060623090856));
#10607=CARTESIAN_POINT('Ctrl Pts',(6.56447880212178,290.036425943689,-6.61243573411802));
#10608=CARTESIAN_POINT('Ctrl Pts',(7.77785103721135,290.173925943689,-4.52836682984767));
#10609=CARTESIAN_POINT('Ctrl Pts',(8.99122327230091,290.311425943689,-2.44429792557732));
#10610=CARTESIAN_POINT('Ctrl Pts',(9.,290.448925943689,-0.032755193697209));
#10611=CARTESIAN_POINT('Ctrl Pts',(9.0087767276991,290.586425943689,2.37878753818289));
#10612=CARTESIAN_POINT('Ctrl Pts',(7.81060623090856,290.723925943689,4.47163317015234));
#10613=CARTESIAN_POINT('Ctrl Pts',(6.61243573411802,290.861425943689,6.56447880212178));
#10614=CARTESIAN_POINT('Ctrl Pts',(4.52836682984767,290.998925943689,7.77785103721135));
#10615=CARTESIAN_POINT('Ctrl Pts',(2.44429792557732,291.136425943689,8.99122327230091));
#10616=CARTESIAN_POINT('Ctrl Pts',(0.0327551936972095,291.273925943689,
9.));
#10617=CARTESIAN_POINT('Ctrl Pts',(-2.37878753818289,291.411425943689,9.0087767276991));
#10618=CARTESIAN_POINT('Ctrl Pts',(-4.47163317015233,291.548925943689,7.81060623090856));
#10619=CARTESIAN_POINT('Ctrl Pts',(-6.56447880212178,291.686425943689,6.61243573411802));
#10620=CARTESIAN_POINT('Ctrl Pts',(-7.77785103721135,291.823925943689,4.52836682984767));
#10621=CARTESIAN_POINT('Ctrl Pts',(-8.99122327230091,291.961425943689,2.44429792557732));
#10622=CARTESIAN_POINT('Ctrl Pts',(-9.,292.098925943689,0.0327551936972079));
#10623=CARTESIAN_POINT('Ctrl Pts',(-9.0087767276991,292.236425943689,-2.3787875381829));
#10624=CARTESIAN_POINT('Ctrl Pts',(-7.81060623090856,292.373925943689,-4.47163317015234));
#10625=CARTESIAN_POINT('Ctrl Pts',(-6.61243573411802,292.511425943689,-6.56447880212179));
#10626=CARTESIAN_POINT('Ctrl Pts',(-4.52836682984766,292.648925943689,-7.77785103721135));
#10627=CARTESIAN_POINT('Ctrl Pts',(-2.44429792557731,292.786425943689,-8.99122327230091));
#10628=CARTESIAN_POINT('Ctrl Pts',(-0.0327551936972084,292.923925943689,
-9.));
#10629=CARTESIAN_POINT('Ctrl Pts',(2.3787875381829,293.061425943689,-9.0087767276991));
#10630=CARTESIAN_POINT('Ctrl Pts',(4.47163317015234,293.198925943689,-7.81060623090856));
#10631=CARTESIAN_POINT('Ctrl Pts',(6.56447880212178,293.336425943689,-6.61243573411802));
#10632=CARTESIAN_POINT('Ctrl Pts',(7.77785103721135,293.473925943689,-4.52836682984767));
#10633=CARTESIAN_POINT('Ctrl Pts',(8.99122327230091,293.611425943689,-2.44429792557732));
#10634=CARTESIAN_POINT('Ctrl Pts',(9.,293.748925943689,-0.032755193697209));
#10635=CARTESIAN_POINT('Ctrl Pts',(9.0087767276991,293.886425943689,2.37878753818289));
#10636=CARTESIAN_POINT('Ctrl Pts',(7.81060623090856,294.023925943689,4.47163317015234));
#10637=CARTESIAN_POINT('Ctrl Pts',(6.61243573411802,294.161425943689,6.56447880212178));
#10638=CARTESIAN_POINT('Ctrl Pts',(4.52836682984767,294.298925943689,7.77785103721135));
#10639=CARTESIAN_POINT('Ctrl Pts',(2.44429792557732,294.436425943689,8.99122327230091));
#10640=CARTESIAN_POINT('Ctrl Pts',(0.0327551936972095,294.573925943689,
9.));
#10641=CARTESIAN_POINT('Ctrl Pts',(-2.37878753818289,294.711425943689,9.0087767276991));
#10642=CARTESIAN_POINT('Ctrl Pts',(-4.47163317015233,294.848925943689,7.81060623090856));
#10643=CARTESIAN_POINT('Ctrl Pts',(-6.56447880212178,294.986425943689,6.61243573411802));
#10644=CARTESIAN_POINT('Ctrl Pts',(-7.77785103721135,295.123925943689,4.52836682984767));
#10645=CARTESIAN_POINT('Ctrl Pts',(-8.99122327230091,295.261425943689,2.44429792557732));
#10646=CARTESIAN_POINT('Ctrl Pts',(-9.,295.398925943689,0.0327551936972079));
#10647=CARTESIAN_POINT('Ctrl Pts',(-9.0087767276991,295.536425943689,-2.3787875381829));
#10648=CARTESIAN_POINT('Ctrl Pts',(-7.81060623090856,295.673925943689,-4.47163317015234));
#10649=CARTESIAN_POINT('Ctrl Pts',(-6.61243573411802,295.811425943689,-6.56447880212179));
#10650=CARTESIAN_POINT('Ctrl Pts',(-4.52836682984766,295.948925943689,-7.77785103721135));
#10651=CARTESIAN_POINT('Ctrl Pts',(-2.44429792557731,296.086425943689,-8.99122327230091));
#10652=CARTESIAN_POINT('Ctrl Pts',(-0.0327551936972084,296.223925943689,
-9.));
#10653=CARTESIAN_POINT('Ctrl Pts',(2.3787875381829,296.361425943689,-9.0087767276991));
#10654=CARTESIAN_POINT('Ctrl Pts',(4.47163317015234,296.498925943689,-7.81060623090856));
#10655=CARTESIAN_POINT('Ctrl Pts',(6.56447880212178,296.636425943689,-6.61243573411802));
#10656=CARTESIAN_POINT('Ctrl Pts',(7.77785103721135,296.773925943689,-4.52836682984767));
#10657=CARTESIAN_POINT('Ctrl Pts',(8.99122327230091,296.911425943689,-2.44429792557732));
#10658=CARTESIAN_POINT('Ctrl Pts',(9.,297.048925943689,-0.032755193697209));
#10659=CARTESIAN_POINT('Ctrl Pts',(9.0087767276991,297.186425943689,2.37878753818289));
#10660=CARTESIAN_POINT('Ctrl Pts',(7.81060623090856,297.323925943689,4.47163317015234));
#10661=CARTESIAN_POINT('Ctrl Pts',(6.61243573411802,297.461425943689,6.56447880212178));
#10662=CARTESIAN_POINT('Ctrl Pts',(4.52836682984767,297.598925943689,7.77785103721135));
#10663=CARTESIAN_POINT('Ctrl Pts',(2.44429792557732,297.736425943689,8.99122327230091));
#10664=CARTESIAN_POINT('Ctrl Pts',(0.0327551936972095,297.873925943689,
9.));
#10665=CARTESIAN_POINT('Ctrl Pts',(-2.37878753818289,298.011425943689,9.0087767276991));
#10666=CARTESIAN_POINT('Ctrl Pts',(-4.47163317015233,298.148925943689,7.81060623090856));
#10667=CARTESIAN_POINT('Ctrl Pts',(-6.56447880212178,298.286425943689,6.61243573411802));
#10668=CARTESIAN_POINT('Ctrl Pts',(-7.77785103721135,298.423925943689,4.52836682984767));
#10669=CARTESIAN_POINT('Ctrl Pts',(-8.99122327230091,298.561425943689,2.44429792557732));
#10670=CARTESIAN_POINT('Ctrl Pts',(-9.,298.698925943689,0.0327551936972079));
#10671=CARTESIAN_POINT('Ctrl Pts',(-9.0087767276991,298.836425943689,-2.3787875381829));
#10672=CARTESIAN_POINT('Ctrl Pts',(-7.81060623090856,298.973925943689,-4.47163317015234));
#10673=CARTESIAN_POINT('Ctrl Pts',(-6.61243573411802,299.111425943689,-6.56447880212179));
#10674=CARTESIAN_POINT('Ctrl Pts',(-4.52836682984766,299.248925943689,-7.77785103721135));
#10675=CARTESIAN_POINT('Ctrl Pts',(-2.44429792557731,299.386425943689,-8.99122327230091));
#10676=CARTESIAN_POINT('Ctrl Pts',(-0.0327551936972084,299.523925943689,
-9.));
#10677=CARTESIAN_POINT('Ctrl Pts',(2.3787875381829,299.661425943689,-9.0087767276991));
#10678=CARTESIAN_POINT('Ctrl Pts',(4.47163317015234,299.798925943689,-7.81060623090856));
#10679=CARTESIAN_POINT('Ctrl Pts',(6.56447880212178,299.936425943689,-6.61243573411802));
#10680=CARTESIAN_POINT('Ctrl Pts',(7.77785103721135,300.073925943689,-4.52836682984767));
#10681=CARTESIAN_POINT('Ctrl Pts',(8.99122327230091,300.211425943689,-2.44429792557732));
#10682=CARTESIAN_POINT('Ctrl Pts',(9.,300.348925943689,-0.032755193697209));
#10683=CARTESIAN_POINT('Ctrl Pts',(9.0087767276991,300.486425943689,2.37878753818289));
#10684=CARTESIAN_POINT('Ctrl Pts',(7.81060623090856,300.623925943689,4.47163317015234));
#10685=CARTESIAN_POINT('Ctrl Pts',(6.61243573411802,300.761425943689,6.56447880212178));
#10686=CARTESIAN_POINT('Ctrl Pts',(4.52836682984767,300.898925943689,7.77785103721135));
#10687=CARTESIAN_POINT('Ctrl Pts',(2.44429792557732,301.036425943689,8.99122327230091));
#10688=CARTESIAN_POINT('Ctrl Pts',(0.0327551936972095,301.173925943689,
9.));
#10689=CARTESIAN_POINT('Ctrl Pts',(-2.37878753818289,301.311425943689,9.0087767276991));
#10690=CARTESIAN_POINT('Ctrl Pts',(-4.47163317015233,301.448925943689,7.81060623090856));
#10691=CARTESIAN_POINT('Ctrl Pts',(-6.56447880212178,301.586425943689,6.61243573411802));
#10692=CARTESIAN_POINT('Ctrl Pts',(-7.77785103721135,301.723925943689,4.52836682984767));
#10693=CARTESIAN_POINT('Ctrl Pts',(-8.99122327230091,301.861425943689,2.44429792557732));
#10694=CARTESIAN_POINT('Ctrl Pts',(-9.,301.998925943689,0.0327551936972079));
#10695=CARTESIAN_POINT('Ctrl Pts',(-9.0087767276991,302.136425943689,-2.3787875381829));
#10696=CARTESIAN_POINT('Ctrl Pts',(-7.81060623090856,302.273925943689,-4.47163317015234));
#10697=CARTESIAN_POINT('Ctrl Pts',(-6.61243573411802,302.411425943689,-6.56447880212179));
#10698=CARTESIAN_POINT('Ctrl Pts',(-4.52836682984766,302.548925943689,-7.77785103721135));
#10699=CARTESIAN_POINT('Ctrl Pts',(-2.44429792557731,302.686425943689,-8.99122327230091));
#10700=CARTESIAN_POINT('Ctrl Pts',(-0.0327551936972084,302.823925943689,
-9.));
#10701=CARTESIAN_POINT('Ctrl Pts',(2.3787875381829,302.961425943689,-9.0087767276991));
#10702=CARTESIAN_POINT('Ctrl Pts',(4.47163317015234,303.098925943689,-7.81060623090856));
#10703=CARTESIAN_POINT('Ctrl Pts',(6.56447880212178,303.236425943689,-6.61243573411802));
#10704=CARTESIAN_POINT('Ctrl Pts',(7.77785103721135,303.373925943689,-4.52836682984767));
#10705=CARTESIAN_POINT('Ctrl Pts',(8.99122327230091,303.511425943689,-2.44429792557732));
#10706=CARTESIAN_POINT('Ctrl Pts',(9.,303.648925943689,-0.032755193697209));
#10707=CARTESIAN_POINT('Ctrl Pts',(9.0087767276991,303.786425943689,2.37878753818289));
#10708=CARTESIAN_POINT('Ctrl Pts',(7.81060623090856,303.923925943689,4.47163317015234));
#10709=CARTESIAN_POINT('Ctrl Pts',(6.61243573411802,304.061425943689,6.56447880212178));
#10710=CARTESIAN_POINT('Ctrl Pts',(4.52836682984767,304.198925943689,7.77785103721135));
#10711=CARTESIAN_POINT('Ctrl Pts',(2.44429792557732,304.336425943689,8.99122327230091));
#10712=CARTESIAN_POINT('Ctrl Pts',(0.0327551936972095,304.473925943689,
9.));
#10713=CARTESIAN_POINT('Ctrl Pts',(-2.37878753818289,304.611425943689,9.0087767276991));
#10714=CARTESIAN_POINT('Ctrl Pts',(-4.47163317015233,304.748925943689,7.81060623090856));
#10715=CARTESIAN_POINT('Ctrl Pts',(-6.56447880212178,304.886425943689,6.61243573411802));
#10716=CARTESIAN_POINT('Ctrl Pts',(-7.77785103721135,305.023925943689,4.52836682984767));
#10717=CARTESIAN_POINT('Ctrl Pts',(-8.99122327230091,305.161425943689,2.44429792557732));
#10718=CARTESIAN_POINT('Ctrl Pts',(-9.,305.298925943689,0.0327551936972079));
#10719=CARTESIAN_POINT('Ctrl Pts',(-9.0087767276991,305.436425943689,-2.3787875381829));
#10720=CARTESIAN_POINT('Ctrl Pts',(-7.81060623090856,305.573925943689,-4.47163317015234));
#10721=CARTESIAN_POINT('Ctrl Pts',(-6.61243573411802,305.711425943689,-6.56447880212179));
#10722=CARTESIAN_POINT('Ctrl Pts',(-4.52836682984766,305.848925943689,-7.77785103721135));
#10723=CARTESIAN_POINT('Ctrl Pts',(-2.44429792557731,305.986425943689,-8.99122327230091));
#10724=CARTESIAN_POINT('Ctrl Pts',(-0.0327551936972084,306.123925943689,
-9.));
#10725=CARTESIAN_POINT('Ctrl Pts',(2.3787875381829,306.261425943689,-9.0087767276991));
#10726=CARTESIAN_POINT('Ctrl Pts',(4.47163317015234,306.398925943689,-7.81060623090856));
#10727=CARTESIAN_POINT('Ctrl Pts',(6.56447880212178,306.536425943689,-6.61243573411802));
#10728=CARTESIAN_POINT('Ctrl Pts',(7.77785103721135,306.673925943689,-4.52836682984767));
#10729=CARTESIAN_POINT('Ctrl Pts',(8.99122327230091,306.811425943689,-2.44429792557732));
#10730=CARTESIAN_POINT('Ctrl Pts',(9.,306.948925943689,-0.032755193697209));
#10731=CARTESIAN_POINT('Ctrl Pts',(9.0087767276991,307.086425943689,2.37878753818289));
#10732=CARTESIAN_POINT('Ctrl Pts',(7.81060623090856,307.223925943689,4.47163317015234));
#10733=CARTESIAN_POINT('Ctrl Pts',(6.61243573411802,307.361425943689,6.56447880212178));
#10734=CARTESIAN_POINT('Ctrl Pts',(4.52836682984767,307.498925943689,7.77785103721135));
#10735=CARTESIAN_POINT('Ctrl Pts',(2.44429792557732,307.636425943689,8.99122327230091));
#10736=CARTESIAN_POINT('Ctrl Pts',(0.0327551936972095,307.773925943689,
9.));
#10737=CARTESIAN_POINT('Ctrl Pts',(-2.37878753818289,307.911425943689,9.0087767276991));
#10738=CARTESIAN_POINT('Ctrl Pts',(-4.47163317015233,308.048925943689,7.81060623090856));
#10739=CARTESIAN_POINT('Ctrl Pts',(-6.56447880212178,308.186425943689,6.61243573411802));
#10740=CARTESIAN_POINT('Ctrl Pts',(-7.77785103721135,308.323925943689,4.52836682984767));
#10741=CARTESIAN_POINT('Ctrl Pts',(-8.99122327230091,308.461425943689,2.44429792557732));
#10742=CARTESIAN_POINT('Ctrl Pts',(-9.,308.598925943689,0.0327551936972079));
#10743=CARTESIAN_POINT('Ctrl Pts',(-9.0087767276991,308.736425943689,-2.3787875381829));
#10744=CARTESIAN_POINT('Ctrl Pts',(-7.81060623090856,308.873925943689,-4.47163317015234));
#10745=CARTESIAN_POINT('Ctrl Pts',(-6.61243573411802,309.011425943689,-6.56447880212179));
#10746=CARTESIAN_POINT('Ctrl Pts',(-4.52836682984766,309.148925943689,-7.77785103721135));
#10747=CARTESIAN_POINT('Ctrl Pts',(-2.44429792557731,309.286425943689,-8.99122327230091));
#10748=CARTESIAN_POINT('Ctrl Pts',(-0.0327551936972084,309.423925943689,
-9.));
#10749=CARTESIAN_POINT('Ctrl Pts',(2.3787875381829,309.561425943689,-9.0087767276991));
#10750=CARTESIAN_POINT('Ctrl Pts',(4.47163317015234,309.698925943689,-7.81060623090856));
#10751=CARTESIAN_POINT('Ctrl Pts',(6.56447880212178,309.836425943689,-6.61243573411802));
#10752=CARTESIAN_POINT('Ctrl Pts',(7.77785103721135,309.973925943689,-4.52836682984767));
#10753=CARTESIAN_POINT('Ctrl Pts',(8.99122327230091,310.111425943689,-2.44429792557732));
#10754=CARTESIAN_POINT('Ctrl Pts',(9.,310.248925943689,-0.032755193697209));
#10755=CARTESIAN_POINT('Ctrl Pts',(9.0087767276991,310.386425943689,2.37878753818289));
#10756=CARTESIAN_POINT('Ctrl Pts',(7.81060623090856,310.523925943689,4.47163317015234));
#10757=CARTESIAN_POINT('Ctrl Pts',(6.61243573411802,310.661425943689,6.56447880212178));
#10758=CARTESIAN_POINT('Ctrl Pts',(4.52836682984767,310.798925943689,7.77785103721135));
#10759=CARTESIAN_POINT('Ctrl Pts',(2.44429792557732,310.936425943689,8.99122327230091));
#10760=CARTESIAN_POINT('Ctrl Pts',(0.0327551936972095,311.073925943689,
9.));
#10761=CARTESIAN_POINT('Ctrl Pts',(-2.37878753818289,311.211425943689,9.0087767276991));
#10762=CARTESIAN_POINT('Ctrl Pts',(-4.47163317015233,311.348925943689,7.81060623090856));
#10763=CARTESIAN_POINT('Ctrl Pts',(-6.56447880212178,311.486425943689,6.61243573411802));
#10764=CARTESIAN_POINT('Ctrl Pts',(-7.77785103721135,311.623925943689,4.52836682984767));
#10765=CARTESIAN_POINT('Ctrl Pts',(-8.99122327230091,311.761425943689,2.44429792557732));
#10766=CARTESIAN_POINT('Ctrl Pts',(-9.,311.898925943689,0.0327551936972079));
#10767=CARTESIAN_POINT('Ctrl Pts',(-9.0087767276991,312.036425943689,-2.3787875381829));
#10768=CARTESIAN_POINT('Ctrl Pts',(-7.81060623090856,312.173925943689,-4.47163317015234));
#10769=CARTESIAN_POINT('Ctrl Pts',(-6.61243573411802,312.311425943689,-6.56447880212179));
#10770=CARTESIAN_POINT('Ctrl Pts',(-4.52836682984766,312.448925943689,-7.77785103721135));
#10771=CARTESIAN_POINT('Ctrl Pts',(-2.44429792557731,312.586425943689,-8.99122327230091));
#10772=CARTESIAN_POINT('Ctrl Pts',(-0.0327551936972084,312.723925943689,
-9.));
#10773=CARTESIAN_POINT('Ctrl Pts',(2.3787875381829,312.861425943689,-9.0087767276991));
#10774=CARTESIAN_POINT('Ctrl Pts',(4.47163317015234,312.998925943689,-7.81060623090856));
#10775=CARTESIAN_POINT('Ctrl Pts',(6.56447880212178,313.136425943689,-6.61243573411802));
#10776=CARTESIAN_POINT('Ctrl Pts',(7.77785103721135,313.273925943689,-4.52836682984767));
#10777=CARTESIAN_POINT('Ctrl Pts',(8.99122327230091,313.411425943689,-2.44429792557732));
#10778=CARTESIAN_POINT('Ctrl Pts',(9.,313.548925943689,-0.032755193697209));
#10779=CARTESIAN_POINT('Ctrl Pts',(9.0087767276991,313.686425943689,2.37878753818289));
#10780=CARTESIAN_POINT('Ctrl Pts',(7.81060623090856,313.823925943689,4.47163317015234));
#10781=CARTESIAN_POINT('Ctrl Pts',(6.61243573411802,313.961425943689,6.56447880212178));
#10782=CARTESIAN_POINT('Ctrl Pts',(4.52836682984767,314.098925943689,7.77785103721135));
#10783=CARTESIAN_POINT('Ctrl Pts',(2.44429792557732,314.236425943689,8.99122327230091));
#10784=CARTESIAN_POINT('Ctrl Pts',(0.0327551936972095,314.373925943689,
9.));
#10785=CARTESIAN_POINT('Ctrl Pts',(-2.37878753818289,314.511425943689,9.0087767276991));
#10786=CARTESIAN_POINT('Ctrl Pts',(-4.47163317015233,314.648925943689,7.81060623090856));
#10787=CARTESIAN_POINT('Ctrl Pts',(-6.56447880212178,314.786425943689,6.61243573411802));
#10788=CARTESIAN_POINT('Ctrl Pts',(-7.77785103721135,314.923925943689,4.52836682984767));
#10789=CARTESIAN_POINT('Ctrl Pts',(-8.99122327230091,315.061425943689,2.44429792557732));
#10790=CARTESIAN_POINT('Ctrl Pts',(-9.,315.198925943689,0.0327551936972079));
#10791=CARTESIAN_POINT('Ctrl Pts',(-9.0087767276991,315.336425943689,-2.3787875381829));
#10792=CARTESIAN_POINT('Ctrl Pts',(-7.81060623090856,315.473925943689,-4.47163317015234));
#10793=CARTESIAN_POINT('Ctrl Pts',(-6.61243573411802,315.611425943689,-6.56447880212179));
#10794=CARTESIAN_POINT('Ctrl Pts',(-4.52836682984766,315.748925943689,-7.77785103721135));
#10795=CARTESIAN_POINT('Ctrl Pts',(-2.44429792557731,315.886425943689,-8.99122327230091));
#10796=CARTESIAN_POINT('Ctrl Pts',(-0.0327551936972084,316.023925943689,
-9.));
#10797=CARTESIAN_POINT('Ctrl Pts',(2.3787875381829,316.161425943689,-9.0087767276991));
#10798=CARTESIAN_POINT('Ctrl Pts',(4.47163317015234,316.298925943689,-7.81060623090856));
#10799=CARTESIAN_POINT('Ctrl Pts',(6.56447880212178,316.436425943689,-6.61243573411802));
#10800=CARTESIAN_POINT('Ctrl Pts',(7.77785103721135,316.573925943689,-4.52836682984767));
#10801=CARTESIAN_POINT('Ctrl Pts',(8.99122327230091,316.711425943689,-2.44429792557732));
#10802=CARTESIAN_POINT('Ctrl Pts',(9.,316.848925943689,-0.032755193697209));
#10803=CARTESIAN_POINT('Ctrl Pts',(9.0087767276991,316.986425943689,2.37878753818289));
#10804=CARTESIAN_POINT('Ctrl Pts',(7.81060623090856,317.123925943689,4.47163317015234));
#10805=CARTESIAN_POINT('Ctrl Pts',(6.61243573411802,317.261425943689,6.56447880212178));
#10806=CARTESIAN_POINT('Ctrl Pts',(4.52836682984767,317.398925943689,7.77785103721135));
#10807=CARTESIAN_POINT('Ctrl Pts',(2.44429792557732,317.536425943689,8.99122327230091));
#10808=CARTESIAN_POINT('Ctrl Pts',(0.0327551936972095,317.673925943689,
9.));
#10809=CARTESIAN_POINT('Ctrl Pts',(-2.37878753818289,317.811425943689,9.0087767276991));
#10810=CARTESIAN_POINT('Ctrl Pts',(-4.47163317015233,317.948925943689,7.81060623090856));
#10811=CARTESIAN_POINT('Ctrl Pts',(-6.56447880212178,318.086425943689,6.61243573411802));
#10812=CARTESIAN_POINT('Ctrl Pts',(-7.77785103721135,318.223925943689,4.52836682984767));
#10813=CARTESIAN_POINT('Ctrl Pts',(-8.99122327230091,318.361425943689,2.44429792557732));
#10814=CARTESIAN_POINT('Ctrl Pts',(-9.,318.498925943689,0.0327551936972079));
#10815=CARTESIAN_POINT('Ctrl Pts',(-8.,285.498925943689,0.0327551936971979));
#10816=CARTESIAN_POINT('Ctrl Pts',(-8.00877672769909,285.636425943689,-2.11083834575178));
#10817=CARTESIAN_POINT('Ctrl Pts',(-6.94458082712411,285.773925943689,-3.97163317015235));
#10818=CARTESIAN_POINT('Ctrl Pts',(-5.88038492654913,285.911425943689,-5.83242799455291));
#10819=CARTESIAN_POINT('Ctrl Pts',(-4.02836682984766,286.048925943689,-6.91182563342691));
#10820=CARTESIAN_POINT('Ctrl Pts',(-2.17634873314618,286.186425943689,-7.99122327230091));
#10821=CARTESIAN_POINT('Ctrl Pts',(-0.0327551936971984,286.323925943689,
-8.));
#10822=CARTESIAN_POINT('Ctrl Pts',(2.11083834575178,286.461425943689,-8.00877672769909));
#10823=CARTESIAN_POINT('Ctrl Pts',(3.97163317015235,286.598925943689,-6.94458082712411));
#10824=CARTESIAN_POINT('Ctrl Pts',(5.83242799455291,286.736425943689,-5.88038492654913));
#10825=CARTESIAN_POINT('Ctrl Pts',(6.91182563342691,286.873925943689,-4.02836682984766));
#10826=CARTESIAN_POINT('Ctrl Pts',(7.99122327230091,287.011425943689,-2.17634873314618));
#10827=CARTESIAN_POINT('Ctrl Pts',(8.,287.148925943689,-0.0327551936971989));
#10828=CARTESIAN_POINT('Ctrl Pts',(8.00877672769909,287.286425943689,2.11083834575178));
#10829=CARTESIAN_POINT('Ctrl Pts',(6.94458082712411,287.423925943689,3.97163317015235));
#10830=CARTESIAN_POINT('Ctrl Pts',(5.88038492654913,287.561425943689,5.83242799455291));
#10831=CARTESIAN_POINT('Ctrl Pts',(4.02836682984766,287.698925943689,6.91182563342691));
#10832=CARTESIAN_POINT('Ctrl Pts',(2.17634873314619,287.836425943689,7.99122327230091));
#10833=CARTESIAN_POINT('Ctrl Pts',(0.0327551936971994,287.973925943689,
8.));
#10834=CARTESIAN_POINT('Ctrl Pts',(-2.11083834575178,288.111425943689,8.00877672769909));
#10835=CARTESIAN_POINT('Ctrl Pts',(-3.97163317015234,288.248925943689,6.94458082712412));
#10836=CARTESIAN_POINT('Ctrl Pts',(-5.83242799455291,288.386425943689,5.88038492654913));
#10837=CARTESIAN_POINT('Ctrl Pts',(-6.91182563342691,288.523925943689,4.02836682984766));
#10838=CARTESIAN_POINT('Ctrl Pts',(-7.99122327230091,288.661425943689,2.17634873314619));
#10839=CARTESIAN_POINT('Ctrl Pts',(-8.,288.798925943689,0.0327551936971979));
#10840=CARTESIAN_POINT('Ctrl Pts',(-8.00877672769909,288.936425943689,-2.11083834575178));
#10841=CARTESIAN_POINT('Ctrl Pts',(-6.94458082712411,289.073925943689,-3.97163317015235));
#10842=CARTESIAN_POINT('Ctrl Pts',(-5.88038492654913,289.211425943689,-5.83242799455291));
#10843=CARTESIAN_POINT('Ctrl Pts',(-4.02836682984766,289.348925943689,-6.91182563342691));
#10844=CARTESIAN_POINT('Ctrl Pts',(-2.17634873314618,289.486425943689,-7.99122327230091));
#10845=CARTESIAN_POINT('Ctrl Pts',(-0.0327551936971984,289.623925943689,
-8.));
#10846=CARTESIAN_POINT('Ctrl Pts',(2.11083834575178,289.761425943689,-8.00877672769909));
#10847=CARTESIAN_POINT('Ctrl Pts',(3.97163317015235,289.898925943689,-6.94458082712411));
#10848=CARTESIAN_POINT('Ctrl Pts',(5.83242799455291,290.036425943689,-5.88038492654913));
#10849=CARTESIAN_POINT('Ctrl Pts',(6.91182563342691,290.173925943689,-4.02836682984766));
#10850=CARTESIAN_POINT('Ctrl Pts',(7.99122327230091,290.311425943689,-2.17634873314618));
#10851=CARTESIAN_POINT('Ctrl Pts',(8.,290.448925943689,-0.0327551936971989));
#10852=CARTESIAN_POINT('Ctrl Pts',(8.00877672769909,290.586425943689,2.11083834575178));
#10853=CARTESIAN_POINT('Ctrl Pts',(6.94458082712411,290.723925943689,3.97163317015235));
#10854=CARTESIAN_POINT('Ctrl Pts',(5.88038492654913,290.861425943689,5.83242799455291));
#10855=CARTESIAN_POINT('Ctrl Pts',(4.02836682984766,290.998925943689,6.91182563342691));
#10856=CARTESIAN_POINT('Ctrl Pts',(2.17634873314619,291.136425943689,7.99122327230091));
#10857=CARTESIAN_POINT('Ctrl Pts',(0.0327551936971994,291.273925943689,
8.));
#10858=CARTESIAN_POINT('Ctrl Pts',(-2.11083834575178,291.411425943689,8.00877672769909));
#10859=CARTESIAN_POINT('Ctrl Pts',(-3.97163317015234,291.548925943689,6.94458082712412));
#10860=CARTESIAN_POINT('Ctrl Pts',(-5.83242799455291,291.686425943689,5.88038492654913));
#10861=CARTESIAN_POINT('Ctrl Pts',(-6.91182563342691,291.823925943689,4.02836682984766));
#10862=CARTESIAN_POINT('Ctrl Pts',(-7.99122327230091,291.961425943689,2.17634873314619));
#10863=CARTESIAN_POINT('Ctrl Pts',(-8.,292.098925943689,0.0327551936971979));
#10864=CARTESIAN_POINT('Ctrl Pts',(-8.00877672769909,292.236425943689,-2.11083834575178));
#10865=CARTESIAN_POINT('Ctrl Pts',(-6.94458082712411,292.373925943689,-3.97163317015235));
#10866=CARTESIAN_POINT('Ctrl Pts',(-5.88038492654913,292.511425943689,-5.83242799455291));
#10867=CARTESIAN_POINT('Ctrl Pts',(-4.02836682984766,292.648925943689,-6.91182563342691));
#10868=CARTESIAN_POINT('Ctrl Pts',(-2.17634873314618,292.786425943689,-7.99122327230091));
#10869=CARTESIAN_POINT('Ctrl Pts',(-0.0327551936971984,292.923925943689,
-8.));
#10870=CARTESIAN_POINT('Ctrl Pts',(2.11083834575178,293.061425943689,-8.00877672769909));
#10871=CARTESIAN_POINT('Ctrl Pts',(3.97163317015235,293.198925943689,-6.94458082712411));
#10872=CARTESIAN_POINT('Ctrl Pts',(5.83242799455291,293.336425943689,-5.88038492654913));
#10873=CARTESIAN_POINT('Ctrl Pts',(6.91182563342691,293.473925943689,-4.02836682984766));
#10874=CARTESIAN_POINT('Ctrl Pts',(7.99122327230091,293.611425943689,-2.17634873314618));
#10875=CARTESIAN_POINT('Ctrl Pts',(8.,293.748925943689,-0.0327551936971989));
#10876=CARTESIAN_POINT('Ctrl Pts',(8.00877672769909,293.886425943689,2.11083834575178));
#10877=CARTESIAN_POINT('Ctrl Pts',(6.94458082712411,294.023925943689,3.97163317015235));
#10878=CARTESIAN_POINT('Ctrl Pts',(5.88038492654913,294.161425943689,5.83242799455291));
#10879=CARTESIAN_POINT('Ctrl Pts',(4.02836682984766,294.298925943689,6.91182563342691));
#10880=CARTESIAN_POINT('Ctrl Pts',(2.17634873314619,294.436425943689,7.99122327230091));
#10881=CARTESIAN_POINT('Ctrl Pts',(0.0327551936971994,294.573925943689,
8.));
#10882=CARTESIAN_POINT('Ctrl Pts',(-2.11083834575178,294.711425943689,8.00877672769909));
#10883=CARTESIAN_POINT('Ctrl Pts',(-3.97163317015234,294.848925943689,6.94458082712412));
#10884=CARTESIAN_POINT('Ctrl Pts',(-5.83242799455291,294.986425943689,5.88038492654913));
#10885=CARTESIAN_POINT('Ctrl Pts',(-6.91182563342691,295.123925943689,4.02836682984766));
#10886=CARTESIAN_POINT('Ctrl Pts',(-7.99122327230091,295.261425943689,2.17634873314619));
#10887=CARTESIAN_POINT('Ctrl Pts',(-8.,295.398925943689,0.0327551936971979));
#10888=CARTESIAN_POINT('Ctrl Pts',(-8.00877672769909,295.536425943689,-2.11083834575178));
#10889=CARTESIAN_POINT('Ctrl Pts',(-6.94458082712411,295.673925943689,-3.97163317015235));
#10890=CARTESIAN_POINT('Ctrl Pts',(-5.88038492654913,295.811425943689,-5.83242799455291));
#10891=CARTESIAN_POINT('Ctrl Pts',(-4.02836682984766,295.948925943689,-6.91182563342691));
#10892=CARTESIAN_POINT('Ctrl Pts',(-2.17634873314618,296.086425943689,-7.99122327230091));
#10893=CARTESIAN_POINT('Ctrl Pts',(-0.0327551936971984,296.223925943689,
-8.));
#10894=CARTESIAN_POINT('Ctrl Pts',(2.11083834575178,296.361425943689,-8.00877672769909));
#10895=CARTESIAN_POINT('Ctrl Pts',(3.97163317015235,296.498925943689,-6.94458082712411));
#10896=CARTESIAN_POINT('Ctrl Pts',(5.83242799455291,296.636425943689,-5.88038492654913));
#10897=CARTESIAN_POINT('Ctrl Pts',(6.91182563342691,296.773925943689,-4.02836682984766));
#10898=CARTESIAN_POINT('Ctrl Pts',(7.99122327230091,296.911425943689,-2.17634873314618));
#10899=CARTESIAN_POINT('Ctrl Pts',(8.,297.048925943689,-0.0327551936971989));
#10900=CARTESIAN_POINT('Ctrl Pts',(8.00877672769909,297.186425943689,2.11083834575178));
#10901=CARTESIAN_POINT('Ctrl Pts',(6.94458082712411,297.323925943689,3.97163317015235));
#10902=CARTESIAN_POINT('Ctrl Pts',(5.88038492654913,297.461425943689,5.83242799455291));
#10903=CARTESIAN_POINT('Ctrl Pts',(4.02836682984766,297.598925943689,6.91182563342691));
#10904=CARTESIAN_POINT('Ctrl Pts',(2.17634873314619,297.736425943689,7.99122327230091));
#10905=CARTESIAN_POINT('Ctrl Pts',(0.0327551936971994,297.873925943689,
8.));
#10906=CARTESIAN_POINT('Ctrl Pts',(-2.11083834575178,298.011425943689,8.00877672769909));
#10907=CARTESIAN_POINT('Ctrl Pts',(-3.97163317015234,298.148925943689,6.94458082712412));
#10908=CARTESIAN_POINT('Ctrl Pts',(-5.83242799455291,298.286425943689,5.88038492654913));
#10909=CARTESIAN_POINT('Ctrl Pts',(-6.91182563342691,298.423925943689,4.02836682984766));
#10910=CARTESIAN_POINT('Ctrl Pts',(-7.99122327230091,298.561425943689,2.17634873314619));
#10911=CARTESIAN_POINT('Ctrl Pts',(-8.,298.698925943689,0.0327551936971979));
#10912=CARTESIAN_POINT('Ctrl Pts',(-8.00877672769909,298.836425943689,-2.11083834575178));
#10913=CARTESIAN_POINT('Ctrl Pts',(-6.94458082712411,298.973925943689,-3.97163317015235));
#10914=CARTESIAN_POINT('Ctrl Pts',(-5.88038492654913,299.111425943689,-5.83242799455291));
#10915=CARTESIAN_POINT('Ctrl Pts',(-4.02836682984766,299.248925943689,-6.91182563342691));
#10916=CARTESIAN_POINT('Ctrl Pts',(-2.17634873314618,299.386425943689,-7.99122327230091));
#10917=CARTESIAN_POINT('Ctrl Pts',(-0.0327551936971984,299.523925943689,
-8.));
#10918=CARTESIAN_POINT('Ctrl Pts',(2.11083834575178,299.661425943689,-8.00877672769909));
#10919=CARTESIAN_POINT('Ctrl Pts',(3.97163317015235,299.798925943689,-6.94458082712411));
#10920=CARTESIAN_POINT('Ctrl Pts',(5.83242799455291,299.936425943689,-5.88038492654913));
#10921=CARTESIAN_POINT('Ctrl Pts',(6.91182563342691,300.073925943689,-4.02836682984766));
#10922=CARTESIAN_POINT('Ctrl Pts',(7.99122327230091,300.211425943689,-2.17634873314618));
#10923=CARTESIAN_POINT('Ctrl Pts',(8.,300.348925943689,-0.0327551936971989));
#10924=CARTESIAN_POINT('Ctrl Pts',(8.00877672769909,300.486425943689,2.11083834575178));
#10925=CARTESIAN_POINT('Ctrl Pts',(6.94458082712411,300.623925943689,3.97163317015235));
#10926=CARTESIAN_POINT('Ctrl Pts',(5.88038492654913,300.761425943689,5.83242799455291));
#10927=CARTESIAN_POINT('Ctrl Pts',(4.02836682984766,300.898925943689,6.91182563342691));
#10928=CARTESIAN_POINT('Ctrl Pts',(2.17634873314619,301.036425943689,7.99122327230091));
#10929=CARTESIAN_POINT('Ctrl Pts',(0.0327551936971994,301.173925943689,
8.));
#10930=CARTESIAN_POINT('Ctrl Pts',(-2.11083834575178,301.311425943689,8.00877672769909));
#10931=CARTESIAN_POINT('Ctrl Pts',(-3.97163317015234,301.448925943689,6.94458082712412));
#10932=CARTESIAN_POINT('Ctrl Pts',(-5.83242799455291,301.586425943689,5.88038492654913));
#10933=CARTESIAN_POINT('Ctrl Pts',(-6.91182563342691,301.723925943689,4.02836682984766));
#10934=CARTESIAN_POINT('Ctrl Pts',(-7.99122327230091,301.861425943689,2.17634873314619));
#10935=CARTESIAN_POINT('Ctrl Pts',(-8.,301.998925943689,0.0327551936971979));
#10936=CARTESIAN_POINT('Ctrl Pts',(-8.00877672769909,302.136425943689,-2.11083834575178));
#10937=CARTESIAN_POINT('Ctrl Pts',(-6.94458082712411,302.273925943689,-3.97163317015235));
#10938=CARTESIAN_POINT('Ctrl Pts',(-5.88038492654913,302.411425943689,-5.83242799455291));
#10939=CARTESIAN_POINT('Ctrl Pts',(-4.02836682984766,302.548925943689,-6.91182563342691));
#10940=CARTESIAN_POINT('Ctrl Pts',(-2.17634873314618,302.686425943689,-7.99122327230091));
#10941=CARTESIAN_POINT('Ctrl Pts',(-0.0327551936971984,302.823925943689,
-8.));
#10942=CARTESIAN_POINT('Ctrl Pts',(2.11083834575178,302.961425943689,-8.00877672769909));
#10943=CARTESIAN_POINT('Ctrl Pts',(3.97163317015235,303.098925943689,-6.94458082712411));
#10944=CARTESIAN_POINT('Ctrl Pts',(5.83242799455291,303.236425943689,-5.88038492654913));
#10945=CARTESIAN_POINT('Ctrl Pts',(6.91182563342691,303.373925943689,-4.02836682984766));
#10946=CARTESIAN_POINT('Ctrl Pts',(7.99122327230091,303.511425943689,-2.17634873314618));
#10947=CARTESIAN_POINT('Ctrl Pts',(8.,303.648925943689,-0.0327551936971989));
#10948=CARTESIAN_POINT('Ctrl Pts',(8.00877672769909,303.786425943689,2.11083834575178));
#10949=CARTESIAN_POINT('Ctrl Pts',(6.94458082712411,303.923925943689,3.97163317015235));
#10950=CARTESIAN_POINT('Ctrl Pts',(5.88038492654913,304.061425943689,5.83242799455291));
#10951=CARTESIAN_POINT('Ctrl Pts',(4.02836682984766,304.198925943689,6.91182563342691));
#10952=CARTESIAN_POINT('Ctrl Pts',(2.17634873314619,304.336425943689,7.99122327230091));
#10953=CARTESIAN_POINT('Ctrl Pts',(0.0327551936971994,304.473925943689,
8.));
#10954=CARTESIAN_POINT('Ctrl Pts',(-2.11083834575178,304.611425943689,8.00877672769909));
#10955=CARTESIAN_POINT('Ctrl Pts',(-3.97163317015234,304.748925943689,6.94458082712412));
#10956=CARTESIAN_POINT('Ctrl Pts',(-5.83242799455291,304.886425943689,5.88038492654913));
#10957=CARTESIAN_POINT('Ctrl Pts',(-6.91182563342691,305.023925943689,4.02836682984766));
#10958=CARTESIAN_POINT('Ctrl Pts',(-7.99122327230091,305.161425943689,2.17634873314619));
#10959=CARTESIAN_POINT('Ctrl Pts',(-8.,305.298925943689,0.0327551936971979));
#10960=CARTESIAN_POINT('Ctrl Pts',(-8.00877672769909,305.436425943689,-2.11083834575178));
#10961=CARTESIAN_POINT('Ctrl Pts',(-6.94458082712411,305.573925943689,-3.97163317015235));
#10962=CARTESIAN_POINT('Ctrl Pts',(-5.88038492654913,305.711425943689,-5.83242799455291));
#10963=CARTESIAN_POINT('Ctrl Pts',(-4.02836682984766,305.848925943689,-6.91182563342691));
#10964=CARTESIAN_POINT('Ctrl Pts',(-2.17634873314618,305.986425943689,-7.99122327230091));
#10965=CARTESIAN_POINT('Ctrl Pts',(-0.0327551936971984,306.123925943689,
-8.));
#10966=CARTESIAN_POINT('Ctrl Pts',(2.11083834575178,306.261425943689,-8.00877672769909));
#10967=CARTESIAN_POINT('Ctrl Pts',(3.97163317015235,306.398925943689,-6.94458082712411));
#10968=CARTESIAN_POINT('Ctrl Pts',(5.83242799455291,306.536425943689,-5.88038492654913));
#10969=CARTESIAN_POINT('Ctrl Pts',(6.91182563342691,306.673925943689,-4.02836682984766));
#10970=CARTESIAN_POINT('Ctrl Pts',(7.99122327230091,306.811425943689,-2.17634873314618));
#10971=CARTESIAN_POINT('Ctrl Pts',(8.,306.948925943689,-0.0327551936971989));
#10972=CARTESIAN_POINT('Ctrl Pts',(8.00877672769909,307.086425943689,2.11083834575178));
#10973=CARTESIAN_POINT('Ctrl Pts',(6.94458082712411,307.223925943689,3.97163317015235));
#10974=CARTESIAN_POINT('Ctrl Pts',(5.88038492654913,307.361425943689,5.83242799455291));
#10975=CARTESIAN_POINT('Ctrl Pts',(4.02836682984766,307.498925943689,6.91182563342691));
#10976=CARTESIAN_POINT('Ctrl Pts',(2.17634873314619,307.636425943689,7.99122327230091));
#10977=CARTESIAN_POINT('Ctrl Pts',(0.0327551936971994,307.773925943689,
8.));
#10978=CARTESIAN_POINT('Ctrl Pts',(-2.11083834575178,307.911425943689,8.00877672769909));
#10979=CARTESIAN_POINT('Ctrl Pts',(-3.97163317015234,308.048925943689,6.94458082712412));
#10980=CARTESIAN_POINT('Ctrl Pts',(-5.83242799455291,308.186425943689,5.88038492654913));
#10981=CARTESIAN_POINT('Ctrl Pts',(-6.91182563342691,308.323925943689,4.02836682984766));
#10982=CARTESIAN_POINT('Ctrl Pts',(-7.99122327230091,308.461425943689,2.17634873314619));
#10983=CARTESIAN_POINT('Ctrl Pts',(-8.,308.598925943689,0.0327551936971979));
#10984=CARTESIAN_POINT('Ctrl Pts',(-8.00877672769909,308.736425943689,-2.11083834575178));
#10985=CARTESIAN_POINT('Ctrl Pts',(-6.94458082712411,308.873925943689,-3.97163317015235));
#10986=CARTESIAN_POINT('Ctrl Pts',(-5.88038492654913,309.011425943689,-5.83242799455291));
#10987=CARTESIAN_POINT('Ctrl Pts',(-4.02836682984766,309.148925943689,-6.91182563342691));
#10988=CARTESIAN_POINT('Ctrl Pts',(-2.17634873314618,309.286425943689,-7.99122327230091));
#10989=CARTESIAN_POINT('Ctrl Pts',(-0.0327551936971984,309.423925943689,
-8.));
#10990=CARTESIAN_POINT('Ctrl Pts',(2.11083834575178,309.561425943689,-8.00877672769909));
#10991=CARTESIAN_POINT('Ctrl Pts',(3.97163317015235,309.698925943689,-6.94458082712411));
#10992=CARTESIAN_POINT('Ctrl Pts',(5.83242799455291,309.836425943689,-5.88038492654913));
#10993=CARTESIAN_POINT('Ctrl Pts',(6.91182563342691,309.973925943689,-4.02836682984766));
#10994=CARTESIAN_POINT('Ctrl Pts',(7.99122327230091,310.111425943689,-2.17634873314618));
#10995=CARTESIAN_POINT('Ctrl Pts',(8.,310.248925943689,-0.0327551936971989));
#10996=CARTESIAN_POINT('Ctrl Pts',(8.00877672769909,310.386425943689,2.11083834575178));
#10997=CARTESIAN_POINT('Ctrl Pts',(6.94458082712411,310.523925943689,3.97163317015235));
#10998=CARTESIAN_POINT('Ctrl Pts',(5.88038492654913,310.661425943689,5.83242799455291));
#10999=CARTESIAN_POINT('Ctrl Pts',(4.02836682984766,310.798925943689,6.91182563342691));
#11000=CARTESIAN_POINT('Ctrl Pts',(2.17634873314619,310.936425943689,7.99122327230091));
#11001=CARTESIAN_POINT('Ctrl Pts',(0.0327551936971994,311.073925943689,
8.));
#11002=CARTESIAN_POINT('Ctrl Pts',(-2.11083834575178,311.211425943689,8.00877672769909));
#11003=CARTESIAN_POINT('Ctrl Pts',(-3.97163317015234,311.348925943689,6.94458082712412));
#11004=CARTESIAN_POINT('Ctrl Pts',(-5.83242799455291,311.486425943689,5.88038492654913));
#11005=CARTESIAN_POINT('Ctrl Pts',(-6.91182563342691,311.623925943689,4.02836682984766));
#11006=CARTESIAN_POINT('Ctrl Pts',(-7.99122327230091,311.761425943689,2.17634873314619));
#11007=CARTESIAN_POINT('Ctrl Pts',(-8.,311.898925943689,0.0327551936971979));
#11008=CARTESIAN_POINT('Ctrl Pts',(-8.00877672769909,312.036425943689,-2.11083834575178));
#11009=CARTESIAN_POINT('Ctrl Pts',(-6.94458082712411,312.173925943689,-3.97163317015235));
#11010=CARTESIAN_POINT('Ctrl Pts',(-5.88038492654913,312.311425943689,-5.83242799455291));
#11011=CARTESIAN_POINT('Ctrl Pts',(-4.02836682984766,312.448925943689,-6.91182563342691));
#11012=CARTESIAN_POINT('Ctrl Pts',(-2.17634873314618,312.586425943689,-7.99122327230091));
#11013=CARTESIAN_POINT('Ctrl Pts',(-0.0327551936971984,312.723925943689,
-8.));
#11014=CARTESIAN_POINT('Ctrl Pts',(2.11083834575178,312.861425943689,-8.00877672769909));
#11015=CARTESIAN_POINT('Ctrl Pts',(3.97163317015235,312.998925943689,-6.94458082712411));
#11016=CARTESIAN_POINT('Ctrl Pts',(5.83242799455291,313.136425943689,-5.88038492654913));
#11017=CARTESIAN_POINT('Ctrl Pts',(6.91182563342691,313.273925943689,-4.02836682984766));
#11018=CARTESIAN_POINT('Ctrl Pts',(7.99122327230091,313.411425943689,-2.17634873314618));
#11019=CARTESIAN_POINT('Ctrl Pts',(8.,313.548925943689,-0.0327551936971989));
#11020=CARTESIAN_POINT('Ctrl Pts',(8.00877672769909,313.686425943689,2.11083834575178));
#11021=CARTESIAN_POINT('Ctrl Pts',(6.94458082712411,313.823925943689,3.97163317015235));
#11022=CARTESIAN_POINT('Ctrl Pts',(5.88038492654913,313.961425943689,5.83242799455291));
#11023=CARTESIAN_POINT('Ctrl Pts',(4.02836682984766,314.098925943689,6.91182563342691));
#11024=CARTESIAN_POINT('Ctrl Pts',(2.17634873314619,314.236425943689,7.99122327230091));
#11025=CARTESIAN_POINT('Ctrl Pts',(0.0327551936971994,314.373925943689,
8.));
#11026=CARTESIAN_POINT('Ctrl Pts',(-2.11083834575178,314.511425943689,8.00877672769909));
#11027=CARTESIAN_POINT('Ctrl Pts',(-3.97163317015234,314.648925943689,6.94458082712412));
#11028=CARTESIAN_POINT('Ctrl Pts',(-5.83242799455291,314.786425943689,5.88038492654913));
#11029=CARTESIAN_POINT('Ctrl Pts',(-6.91182563342691,314.923925943689,4.02836682984766));
#11030=CARTESIAN_POINT('Ctrl Pts',(-7.99122327230091,315.061425943689,2.17634873314619));
#11031=CARTESIAN_POINT('Ctrl Pts',(-8.,315.198925943689,0.0327551936971979));
#11032=CARTESIAN_POINT('Ctrl Pts',(-8.00877672769909,315.336425943689,-2.11083834575178));
#11033=CARTESIAN_POINT('Ctrl Pts',(-6.94458082712411,315.473925943689,-3.97163317015235));
#11034=CARTESIAN_POINT('Ctrl Pts',(-5.88038492654913,315.611425943689,-5.83242799455291));
#11035=CARTESIAN_POINT('Ctrl Pts',(-4.02836682984766,315.748925943689,-6.91182563342691));
#11036=CARTESIAN_POINT('Ctrl Pts',(-2.17634873314618,315.886425943689,-7.99122327230091));
#11037=CARTESIAN_POINT('Ctrl Pts',(-0.0327551936971984,316.023925943689,
-8.));
#11038=CARTESIAN_POINT('Ctrl Pts',(2.11083834575178,316.161425943689,-8.00877672769909));
#11039=CARTESIAN_POINT('Ctrl Pts',(3.97163317015235,316.298925943689,-6.94458082712411));
#11040=CARTESIAN_POINT('Ctrl Pts',(5.83242799455291,316.436425943689,-5.88038492654913));
#11041=CARTESIAN_POINT('Ctrl Pts',(6.91182563342691,316.573925943689,-4.02836682984766));
#11042=CARTESIAN_POINT('Ctrl Pts',(7.99122327230091,316.711425943689,-2.17634873314618));
#11043=CARTESIAN_POINT('Ctrl Pts',(8.,316.848925943689,-0.0327551936971989));
#11044=CARTESIAN_POINT('Ctrl Pts',(8.00877672769909,316.986425943689,2.11083834575178));
#11045=CARTESIAN_POINT('Ctrl Pts',(6.94458082712411,317.123925943689,3.97163317015235));
#11046=CARTESIAN_POINT('Ctrl Pts',(5.88038492654913,317.261425943689,5.83242799455291));
#11047=CARTESIAN_POINT('Ctrl Pts',(4.02836682984766,317.398925943689,6.91182563342691));
#11048=CARTESIAN_POINT('Ctrl Pts',(2.17634873314619,317.536425943689,7.99122327230091));
#11049=CARTESIAN_POINT('Ctrl Pts',(0.0327551936971994,317.673925943689,
8.));
#11050=CARTESIAN_POINT('Ctrl Pts',(-2.11083834575178,317.811425943689,8.00877672769909));
#11051=CARTESIAN_POINT('Ctrl Pts',(-3.97163317015234,317.948925943689,6.94458082712412));
#11052=CARTESIAN_POINT('Ctrl Pts',(-5.83242799455291,318.086425943689,5.88038492654913));
#11053=CARTESIAN_POINT('Ctrl Pts',(-6.91182563342691,318.223925943689,4.02836682984766));
#11054=CARTESIAN_POINT('Ctrl Pts',(-7.99122327230091,318.361425943689,2.17634873314619));
#11055=CARTESIAN_POINT('Ctrl Pts',(-8.,318.498925943689,0.0327551936971979));
#11056=CARTESIAN_POINT('',(-7.50000000000002,285.,7.09974019720158E-14));
#11057=CARTESIAN_POINT('',(-4.63461213585577,285.,-6.52084682022915));
#11058=CARTESIAN_POINT('Ctrl Pts',(-7.50000000000001,285.,6.80011602582908E-14));
#11059=CARTESIAN_POINT('Ctrl Pts',(-7.50000000000002,285.,-0.640878818835817));
#11060=CARTESIAN_POINT('Ctrl Pts',(-7.42362312326954,284.999999999915,-1.27925531817836));
#11061=CARTESIAN_POINT('Ctrl Pts',(-7.13891193975039,284.999999999915,-2.46203415496977));
#11062=CARTESIAN_POINT('Ctrl Pts',(-6.94590651594617,285.,-3.00519525865999));
#11063=CARTESIAN_POINT('Ctrl Pts',(-6.26573749532748,285.,-4.43472731642613));
#11064=CARTESIAN_POINT('Ctrl Pts',(-5.73854794084772,285.,-5.12189946350785));
#11065=CARTESIAN_POINT('Ctrl Pts',(-5.09309463692861,285.,-5.88949436501166));
#11066=CARTESIAN_POINT('Ctrl Pts',(-4.87997203238035,285.,-6.11853899605642));
#11067=CARTESIAN_POINT('Ctrl Pts',(-4.70123367905775,285.,-6.34515496162355));
#11068=CARTESIAN_POINT('Ctrl Pts',(-4.66326630707557,284.999999999928,-6.39956489306395));
#11069=CARTESIAN_POINT('Ctrl Pts',(-4.63521738668531,284.999999999928,-6.45935774756588));
#11070=CARTESIAN_POINT('Ctrl Pts',(-4.6295370291925,285.,-6.47584643979257));
#11071=CARTESIAN_POINT('Ctrl Pts',(-4.6275602093536,285.,-6.49596857752024));
#11072=CARTESIAN_POINT('Ctrl Pts',(-4.62763059707101,285.,-6.50190778381856));
#11073=CARTESIAN_POINT('Ctrl Pts',(-4.62938802811186,285.,-6.51001336052072));
#11074=CARTESIAN_POINT('Ctrl Pts',(-4.63013379953918,285.,-6.51240227717505));
#11075=CARTESIAN_POINT('Ctrl Pts',(-4.63207907295903,285.,-6.51687345550803));
#11076=CARTESIAN_POINT('Ctrl Pts',(-4.63323085894002,285.,-6.51892013394952));
#11077=CARTESIAN_POINT('Ctrl Pts',(-4.63461213585325,285.,-6.52084682023095));
#11078=CARTESIAN_POINT('',(-8.,317.501074056311,-0.0327551936970314));
#11079=CARTESIAN_POINT('Ctrl Pts',(-4.63461213585577,285.,-6.52084682022915));
#11080=CARTESIAN_POINT('Ctrl Pts',(-4.31355406079092,285.025808443012,-6.7490349209516));
#11081=CARTESIAN_POINT('Ctrl Pts',(-3.97163317015249,285.051074056311,-6.94458082712403));
#11082=CARTESIAN_POINT('Ctrl Pts',(-2.11083834575195,285.188574056311,-8.00877672769905));
#11083=CARTESIAN_POINT('Ctrl Pts',(0.0327551936970309,285.326074056311,
-8.));
#11084=CARTESIAN_POINT('Ctrl Pts',(2.17634873314601,285.463574056311,-7.99122327230096));
#11085=CARTESIAN_POINT('Ctrl Pts',(4.02836682984751,285.601074056311,-6.911825633427));
#11086=CARTESIAN_POINT('Ctrl Pts',(5.88038492654901,285.738574056311,-5.83242799455303));
#11087=CARTESIAN_POINT('Ctrl Pts',(6.94458082712403,285.876074056311,-3.9716331701525));
#11088=CARTESIAN_POINT('Ctrl Pts',(8.00877672769905,286.013574056311,-2.11083834575195));
#11089=CARTESIAN_POINT('Ctrl Pts',(8.,286.151074056311,0.0327551936970304));
#11090=CARTESIAN_POINT('Ctrl Pts',(7.99122327230096,286.288574056311,2.17634873314601));
#11091=CARTESIAN_POINT('Ctrl Pts',(6.911825633427,286.426074056311,4.02836682984751));
#11092=CARTESIAN_POINT('Ctrl Pts',(5.83242799455304,286.563574056311,5.880384926549));
#11093=CARTESIAN_POINT('Ctrl Pts',(3.9716331701525,286.701074056311,6.94458082712403));
#11094=CARTESIAN_POINT('Ctrl Pts',(2.11083834575196,286.838574056311,8.00877672769905));
#11095=CARTESIAN_POINT('Ctrl Pts',(-0.0327551936970299,286.976074056311,
8.));
#11096=CARTESIAN_POINT('Ctrl Pts',(-2.17634873314601,287.113574056311,7.99122327230096));
#11097=CARTESIAN_POINT('Ctrl Pts',(-4.02836682984751,287.251074056311,6.911825633427));
#11098=CARTESIAN_POINT('Ctrl Pts',(-5.88038492654901,287.388574056311,5.83242799455303));
#11099=CARTESIAN_POINT('Ctrl Pts',(-6.94458082712403,287.526074056311,3.9716331701525));
#11100=CARTESIAN_POINT('Ctrl Pts',(-8.00877672769905,287.663574056311,2.11083834575196));
#11101=CARTESIAN_POINT('Ctrl Pts',(-8.,287.801074056311,-0.0327551936970314));
#11102=CARTESIAN_POINT('Ctrl Pts',(-7.99122327230096,287.938574056311,-2.17634873314601));
#11103=CARTESIAN_POINT('Ctrl Pts',(-6.911825633427,288.076074056311,-4.02836682984751));
#11104=CARTESIAN_POINT('Ctrl Pts',(-5.83242799455303,288.213574056311,-5.88038492654901));
#11105=CARTESIAN_POINT('Ctrl Pts',(-3.97163317015249,288.351074056311,-6.94458082712403));
#11106=CARTESIAN_POINT('Ctrl Pts',(-2.11083834575195,288.488574056311,-8.00877672769905));
#11107=CARTESIAN_POINT('Ctrl Pts',(0.0327551936970309,288.626074056311,
-8.));
#11108=CARTESIAN_POINT('Ctrl Pts',(2.17634873314601,288.763574056311,-7.99122327230096));
#11109=CARTESIAN_POINT('Ctrl Pts',(4.02836682984751,288.901074056311,-6.911825633427));
#11110=CARTESIAN_POINT('Ctrl Pts',(5.88038492654901,289.038574056311,-5.83242799455303));
#11111=CARTESIAN_POINT('Ctrl Pts',(6.94458082712403,289.176074056311,-3.9716331701525));
#11112=CARTESIAN_POINT('Ctrl Pts',(8.00877672769905,289.313574056311,-2.11083834575195));
#11113=CARTESIAN_POINT('Ctrl Pts',(8.,289.451074056311,0.0327551936970304));
#11114=CARTESIAN_POINT('Ctrl Pts',(7.99122327230096,289.588574056311,2.17634873314601));
#11115=CARTESIAN_POINT('Ctrl Pts',(6.911825633427,289.726074056311,4.02836682984751));
#11116=CARTESIAN_POINT('Ctrl Pts',(5.83242799455304,289.863574056311,5.880384926549));
#11117=CARTESIAN_POINT('Ctrl Pts',(3.9716331701525,290.001074056311,6.94458082712403));
#11118=CARTESIAN_POINT('Ctrl Pts',(2.11083834575196,290.138574056311,8.00877672769905));
#11119=CARTESIAN_POINT('Ctrl Pts',(-0.0327551936970299,290.276074056311,
8.));
#11120=CARTESIAN_POINT('Ctrl Pts',(-2.17634873314601,290.413574056311,7.99122327230096));
#11121=CARTESIAN_POINT('Ctrl Pts',(-4.02836682984751,290.551074056311,6.911825633427));
#11122=CARTESIAN_POINT('Ctrl Pts',(-5.88038492654901,290.688574056311,5.83242799455303));
#11123=CARTESIAN_POINT('Ctrl Pts',(-6.94458082712403,290.826074056311,3.9716331701525));
#11124=CARTESIAN_POINT('Ctrl Pts',(-8.00877672769905,290.963574056311,2.11083834575196));
#11125=CARTESIAN_POINT('Ctrl Pts',(-8.,291.101074056311,-0.0327551936970314));
#11126=CARTESIAN_POINT('Ctrl Pts',(-7.99122327230096,291.238574056311,-2.17634873314601));
#11127=CARTESIAN_POINT('Ctrl Pts',(-6.911825633427,291.376074056311,-4.02836682984751));
#11128=CARTESIAN_POINT('Ctrl Pts',(-5.83242799455303,291.513574056311,-5.88038492654901));
#11129=CARTESIAN_POINT('Ctrl Pts',(-3.97163317015249,291.651074056311,-6.94458082712403));
#11130=CARTESIAN_POINT('Ctrl Pts',(-2.11083834575195,291.788574056311,-8.00877672769905));
#11131=CARTESIAN_POINT('Ctrl Pts',(0.0327551936970309,291.926074056311,
-8.));
#11132=CARTESIAN_POINT('Ctrl Pts',(2.17634873314601,292.063574056311,-7.99122327230096));
#11133=CARTESIAN_POINT('Ctrl Pts',(4.02836682984751,292.201074056311,-6.911825633427));
#11134=CARTESIAN_POINT('Ctrl Pts',(5.88038492654901,292.338574056311,-5.83242799455303));
#11135=CARTESIAN_POINT('Ctrl Pts',(6.94458082712403,292.476074056311,-3.9716331701525));
#11136=CARTESIAN_POINT('Ctrl Pts',(8.00877672769905,292.613574056311,-2.11083834575195));
#11137=CARTESIAN_POINT('Ctrl Pts',(8.,292.751074056311,0.0327551936970304));
#11138=CARTESIAN_POINT('Ctrl Pts',(7.99122327230096,292.888574056311,2.17634873314601));
#11139=CARTESIAN_POINT('Ctrl Pts',(6.911825633427,293.026074056311,4.02836682984751));
#11140=CARTESIAN_POINT('Ctrl Pts',(5.83242799455304,293.163574056311,5.880384926549));
#11141=CARTESIAN_POINT('Ctrl Pts',(3.9716331701525,293.301074056311,6.94458082712403));
#11142=CARTESIAN_POINT('Ctrl Pts',(2.11083834575196,293.438574056311,8.00877672769905));
#11143=CARTESIAN_POINT('Ctrl Pts',(-0.0327551936970299,293.576074056311,
8.));
#11144=CARTESIAN_POINT('Ctrl Pts',(-2.17634873314601,293.713574056311,7.99122327230096));
#11145=CARTESIAN_POINT('Ctrl Pts',(-4.02836682984751,293.851074056311,6.911825633427));
#11146=CARTESIAN_POINT('Ctrl Pts',(-5.88038492654901,293.988574056311,5.83242799455303));
#11147=CARTESIAN_POINT('Ctrl Pts',(-6.94458082712403,294.126074056311,3.9716331701525));
#11148=CARTESIAN_POINT('Ctrl Pts',(-8.00877672769905,294.263574056311,2.11083834575196));
#11149=CARTESIAN_POINT('Ctrl Pts',(-8.,294.401074056311,-0.0327551936970314));
#11150=CARTESIAN_POINT('Ctrl Pts',(-7.99122327230096,294.538574056311,-2.17634873314601));
#11151=CARTESIAN_POINT('Ctrl Pts',(-6.911825633427,294.676074056311,-4.02836682984751));
#11152=CARTESIAN_POINT('Ctrl Pts',(-5.83242799455303,294.813574056311,-5.88038492654901));
#11153=CARTESIAN_POINT('Ctrl Pts',(-3.97163317015249,294.951074056311,-6.94458082712403));
#11154=CARTESIAN_POINT('Ctrl Pts',(-2.11083834575195,295.088574056311,-8.00877672769905));
#11155=CARTESIAN_POINT('Ctrl Pts',(0.0327551936970309,295.226074056311,
-8.));
#11156=CARTESIAN_POINT('Ctrl Pts',(2.17634873314601,295.363574056311,-7.99122327230096));
#11157=CARTESIAN_POINT('Ctrl Pts',(4.02836682984751,295.501074056311,-6.911825633427));
#11158=CARTESIAN_POINT('Ctrl Pts',(5.88038492654901,295.638574056311,-5.83242799455303));
#11159=CARTESIAN_POINT('Ctrl Pts',(6.94458082712403,295.776074056311,-3.9716331701525));
#11160=CARTESIAN_POINT('Ctrl Pts',(8.00877672769905,295.913574056311,-2.11083834575195));
#11161=CARTESIAN_POINT('Ctrl Pts',(8.,296.051074056311,0.0327551936970304));
#11162=CARTESIAN_POINT('Ctrl Pts',(7.99122327230096,296.188574056311,2.17634873314601));
#11163=CARTESIAN_POINT('Ctrl Pts',(6.911825633427,296.326074056311,4.02836682984751));
#11164=CARTESIAN_POINT('Ctrl Pts',(5.83242799455304,296.463574056311,5.880384926549));
#11165=CARTESIAN_POINT('Ctrl Pts',(3.9716331701525,296.601074056311,6.94458082712403));
#11166=CARTESIAN_POINT('Ctrl Pts',(2.11083834575196,296.738574056311,8.00877672769905));
#11167=CARTESIAN_POINT('Ctrl Pts',(-0.0327551936970299,296.876074056311,
8.));
#11168=CARTESIAN_POINT('Ctrl Pts',(-2.17634873314601,297.013574056311,7.99122327230096));
#11169=CARTESIAN_POINT('Ctrl Pts',(-4.02836682984751,297.151074056311,6.911825633427));
#11170=CARTESIAN_POINT('Ctrl Pts',(-5.88038492654901,297.288574056311,5.83242799455303));
#11171=CARTESIAN_POINT('Ctrl Pts',(-6.94458082712403,297.426074056311,3.9716331701525));
#11172=CARTESIAN_POINT('Ctrl Pts',(-8.00877672769905,297.563574056311,2.11083834575196));
#11173=CARTESIAN_POINT('Ctrl Pts',(-8.,297.701074056311,-0.0327551936970314));
#11174=CARTESIAN_POINT('Ctrl Pts',(-7.99122327230096,297.838574056311,-2.17634873314601));
#11175=CARTESIAN_POINT('Ctrl Pts',(-6.911825633427,297.976074056311,-4.02836682984751));
#11176=CARTESIAN_POINT('Ctrl Pts',(-5.83242799455303,298.113574056311,-5.88038492654901));
#11177=CARTESIAN_POINT('Ctrl Pts',(-3.97163317015249,298.251074056311,-6.94458082712403));
#11178=CARTESIAN_POINT('Ctrl Pts',(-2.11083834575195,298.388574056311,-8.00877672769905));
#11179=CARTESIAN_POINT('Ctrl Pts',(0.0327551936970309,298.526074056311,
-8.));
#11180=CARTESIAN_POINT('Ctrl Pts',(2.17634873314601,298.663574056311,-7.99122327230096));
#11181=CARTESIAN_POINT('Ctrl Pts',(4.02836682984751,298.801074056311,-6.911825633427));
#11182=CARTESIAN_POINT('Ctrl Pts',(5.88038492654901,298.938574056311,-5.83242799455303));
#11183=CARTESIAN_POINT('Ctrl Pts',(6.94458082712403,299.076074056311,-3.9716331701525));
#11184=CARTESIAN_POINT('Ctrl Pts',(8.00877672769905,299.213574056311,-2.11083834575195));
#11185=CARTESIAN_POINT('Ctrl Pts',(8.,299.351074056311,0.0327551936970304));
#11186=CARTESIAN_POINT('Ctrl Pts',(7.99122327230096,299.488574056311,2.17634873314601));
#11187=CARTESIAN_POINT('Ctrl Pts',(6.911825633427,299.626074056311,4.02836682984751));
#11188=CARTESIAN_POINT('Ctrl Pts',(5.83242799455304,299.763574056311,5.880384926549));
#11189=CARTESIAN_POINT('Ctrl Pts',(3.9716331701525,299.901074056311,6.94458082712403));
#11190=CARTESIAN_POINT('Ctrl Pts',(2.11083834575196,300.038574056311,8.00877672769905));
#11191=CARTESIAN_POINT('Ctrl Pts',(-0.0327551936970299,300.176074056311,
8.));
#11192=CARTESIAN_POINT('Ctrl Pts',(-2.17634873314601,300.313574056311,7.99122327230096));
#11193=CARTESIAN_POINT('Ctrl Pts',(-4.02836682984751,300.451074056311,6.911825633427));
#11194=CARTESIAN_POINT('Ctrl Pts',(-5.88038492654901,300.588574056311,5.83242799455303));
#11195=CARTESIAN_POINT('Ctrl Pts',(-6.94458082712403,300.726074056311,3.9716331701525));
#11196=CARTESIAN_POINT('Ctrl Pts',(-8.00877672769905,300.863574056311,2.11083834575196));
#11197=CARTESIAN_POINT('Ctrl Pts',(-8.,301.001074056311,-0.0327551936970314));
#11198=CARTESIAN_POINT('Ctrl Pts',(-7.99122327230096,301.138574056311,-2.17634873314601));
#11199=CARTESIAN_POINT('Ctrl Pts',(-6.911825633427,301.276074056311,-4.02836682984751));
#11200=CARTESIAN_POINT('Ctrl Pts',(-5.83242799455303,301.413574056311,-5.88038492654901));
#11201=CARTESIAN_POINT('Ctrl Pts',(-3.97163317015249,301.551074056311,-6.94458082712403));
#11202=CARTESIAN_POINT('Ctrl Pts',(-2.11083834575195,301.688574056311,-8.00877672769905));
#11203=CARTESIAN_POINT('Ctrl Pts',(0.0327551936970309,301.826074056311,
-8.));
#11204=CARTESIAN_POINT('Ctrl Pts',(2.17634873314601,301.963574056311,-7.99122327230096));
#11205=CARTESIAN_POINT('Ctrl Pts',(4.02836682984751,302.101074056311,-6.911825633427));
#11206=CARTESIAN_POINT('Ctrl Pts',(5.88038492654901,302.238574056311,-5.83242799455303));
#11207=CARTESIAN_POINT('Ctrl Pts',(6.94458082712403,302.376074056311,-3.9716331701525));
#11208=CARTESIAN_POINT('Ctrl Pts',(8.00877672769905,302.513574056311,-2.11083834575195));
#11209=CARTESIAN_POINT('Ctrl Pts',(8.,302.651074056311,0.0327551936970304));
#11210=CARTESIAN_POINT('Ctrl Pts',(7.99122327230096,302.788574056311,2.17634873314601));
#11211=CARTESIAN_POINT('Ctrl Pts',(6.911825633427,302.926074056311,4.02836682984751));
#11212=CARTESIAN_POINT('Ctrl Pts',(5.83242799455304,303.063574056311,5.880384926549));
#11213=CARTESIAN_POINT('Ctrl Pts',(3.9716331701525,303.201074056311,6.94458082712403));
#11214=CARTESIAN_POINT('Ctrl Pts',(2.11083834575196,303.338574056311,8.00877672769905));
#11215=CARTESIAN_POINT('Ctrl Pts',(-0.0327551936970299,303.476074056311,
8.));
#11216=CARTESIAN_POINT('Ctrl Pts',(-2.17634873314601,303.613574056311,7.99122327230096));
#11217=CARTESIAN_POINT('Ctrl Pts',(-4.02836682984751,303.751074056311,6.911825633427));
#11218=CARTESIAN_POINT('Ctrl Pts',(-5.88038492654901,303.888574056311,5.83242799455303));
#11219=CARTESIAN_POINT('Ctrl Pts',(-6.94458082712403,304.026074056311,3.9716331701525));
#11220=CARTESIAN_POINT('Ctrl Pts',(-8.00877672769905,304.163574056311,2.11083834575196));
#11221=CARTESIAN_POINT('Ctrl Pts',(-8.,304.301074056311,-0.0327551936970314));
#11222=CARTESIAN_POINT('Ctrl Pts',(-7.99122327230096,304.438574056311,-2.17634873314601));
#11223=CARTESIAN_POINT('Ctrl Pts',(-6.911825633427,304.576074056311,-4.02836682984751));
#11224=CARTESIAN_POINT('Ctrl Pts',(-5.83242799455303,304.713574056311,-5.88038492654901));
#11225=CARTESIAN_POINT('Ctrl Pts',(-3.97163317015249,304.851074056311,-6.94458082712403));
#11226=CARTESIAN_POINT('Ctrl Pts',(-2.11083834575195,304.988574056311,-8.00877672769905));
#11227=CARTESIAN_POINT('Ctrl Pts',(0.0327551936970309,305.126074056311,
-8.));
#11228=CARTESIAN_POINT('Ctrl Pts',(2.17634873314601,305.263574056311,-7.99122327230096));
#11229=CARTESIAN_POINT('Ctrl Pts',(4.02836682984751,305.401074056311,-6.911825633427));
#11230=CARTESIAN_POINT('Ctrl Pts',(5.88038492654901,305.538574056311,-5.83242799455303));
#11231=CARTESIAN_POINT('Ctrl Pts',(6.94458082712403,305.676074056311,-3.9716331701525));
#11232=CARTESIAN_POINT('Ctrl Pts',(8.00877672769905,305.813574056311,-2.11083834575195));
#11233=CARTESIAN_POINT('Ctrl Pts',(8.,305.951074056311,0.0327551936970304));
#11234=CARTESIAN_POINT('Ctrl Pts',(7.99122327230096,306.088574056311,2.17634873314601));
#11235=CARTESIAN_POINT('Ctrl Pts',(6.911825633427,306.226074056311,4.02836682984751));
#11236=CARTESIAN_POINT('Ctrl Pts',(5.83242799455304,306.363574056311,5.880384926549));
#11237=CARTESIAN_POINT('Ctrl Pts',(3.9716331701525,306.501074056311,6.94458082712403));
#11238=CARTESIAN_POINT('Ctrl Pts',(2.11083834575196,306.638574056311,8.00877672769905));
#11239=CARTESIAN_POINT('Ctrl Pts',(-0.0327551936970299,306.776074056311,
8.));
#11240=CARTESIAN_POINT('Ctrl Pts',(-2.17634873314601,306.913574056311,7.99122327230096));
#11241=CARTESIAN_POINT('Ctrl Pts',(-4.02836682984751,307.051074056311,6.911825633427));
#11242=CARTESIAN_POINT('Ctrl Pts',(-5.88038492654901,307.188574056311,5.83242799455303));
#11243=CARTESIAN_POINT('Ctrl Pts',(-6.94458082712403,307.326074056311,3.9716331701525));
#11244=CARTESIAN_POINT('Ctrl Pts',(-8.00877672769905,307.463574056311,2.11083834575196));
#11245=CARTESIAN_POINT('Ctrl Pts',(-8.,307.601074056311,-0.0327551936970314));
#11246=CARTESIAN_POINT('Ctrl Pts',(-7.99122327230096,307.738574056311,-2.17634873314601));
#11247=CARTESIAN_POINT('Ctrl Pts',(-6.911825633427,307.876074056311,-4.02836682984751));
#11248=CARTESIAN_POINT('Ctrl Pts',(-5.83242799455303,308.013574056311,-5.88038492654901));
#11249=CARTESIAN_POINT('Ctrl Pts',(-3.97163317015249,308.151074056311,-6.94458082712403));
#11250=CARTESIAN_POINT('Ctrl Pts',(-2.11083834575195,308.288574056311,-8.00877672769905));
#11251=CARTESIAN_POINT('Ctrl Pts',(0.0327551936970309,308.426074056311,
-8.));
#11252=CARTESIAN_POINT('Ctrl Pts',(2.17634873314601,308.563574056311,-7.99122327230096));
#11253=CARTESIAN_POINT('Ctrl Pts',(4.02836682984751,308.701074056311,-6.911825633427));
#11254=CARTESIAN_POINT('Ctrl Pts',(5.88038492654901,308.838574056311,-5.83242799455303));
#11255=CARTESIAN_POINT('Ctrl Pts',(6.94458082712403,308.976074056311,-3.9716331701525));
#11256=CARTESIAN_POINT('Ctrl Pts',(8.00877672769905,309.113574056311,-2.11083834575195));
#11257=CARTESIAN_POINT('Ctrl Pts',(8.,309.251074056311,0.0327551936970304));
#11258=CARTESIAN_POINT('Ctrl Pts',(7.99122327230096,309.388574056311,2.17634873314601));
#11259=CARTESIAN_POINT('Ctrl Pts',(6.911825633427,309.526074056311,4.02836682984751));
#11260=CARTESIAN_POINT('Ctrl Pts',(5.83242799455304,309.663574056311,5.880384926549));
#11261=CARTESIAN_POINT('Ctrl Pts',(3.9716331701525,309.801074056311,6.94458082712403));
#11262=CARTESIAN_POINT('Ctrl Pts',(2.11083834575196,309.938574056311,8.00877672769905));
#11263=CARTESIAN_POINT('Ctrl Pts',(-0.0327551936970299,310.076074056311,
8.));
#11264=CARTESIAN_POINT('Ctrl Pts',(-2.17634873314601,310.213574056311,7.99122327230096));
#11265=CARTESIAN_POINT('Ctrl Pts',(-4.02836682984751,310.351074056311,6.911825633427));
#11266=CARTESIAN_POINT('Ctrl Pts',(-5.88038492654901,310.488574056311,5.83242799455303));
#11267=CARTESIAN_POINT('Ctrl Pts',(-6.94458082712403,310.626074056311,3.9716331701525));
#11268=CARTESIAN_POINT('Ctrl Pts',(-8.00877672769905,310.763574056311,2.11083834575196));
#11269=CARTESIAN_POINT('Ctrl Pts',(-8.,310.901074056311,-0.0327551936970314));
#11270=CARTESIAN_POINT('Ctrl Pts',(-7.99122327230096,311.038574056311,-2.17634873314601));
#11271=CARTESIAN_POINT('Ctrl Pts',(-6.911825633427,311.176074056311,-4.02836682984751));
#11272=CARTESIAN_POINT('Ctrl Pts',(-5.83242799455303,311.313574056311,-5.88038492654901));
#11273=CARTESIAN_POINT('Ctrl Pts',(-3.97163317015249,311.451074056311,-6.94458082712403));
#11274=CARTESIAN_POINT('Ctrl Pts',(-2.11083834575195,311.588574056311,-8.00877672769905));
#11275=CARTESIAN_POINT('Ctrl Pts',(0.0327551936970309,311.726074056311,
-8.));
#11276=CARTESIAN_POINT('Ctrl Pts',(2.17634873314601,311.863574056311,-7.99122327230096));
#11277=CARTESIAN_POINT('Ctrl Pts',(4.02836682984751,312.001074056311,-6.911825633427));
#11278=CARTESIAN_POINT('Ctrl Pts',(5.88038492654901,312.138574056311,-5.83242799455303));
#11279=CARTESIAN_POINT('Ctrl Pts',(6.94458082712403,312.276074056311,-3.9716331701525));
#11280=CARTESIAN_POINT('Ctrl Pts',(8.00877672769905,312.413574056311,-2.11083834575195));
#11281=CARTESIAN_POINT('Ctrl Pts',(8.,312.551074056311,0.0327551936970304));
#11282=CARTESIAN_POINT('Ctrl Pts',(7.99122327230096,312.688574056311,2.17634873314601));
#11283=CARTESIAN_POINT('Ctrl Pts',(6.911825633427,312.826074056311,4.02836682984751));
#11284=CARTESIAN_POINT('Ctrl Pts',(5.83242799455304,312.963574056311,5.880384926549));
#11285=CARTESIAN_POINT('Ctrl Pts',(3.9716331701525,313.101074056311,6.94458082712403));
#11286=CARTESIAN_POINT('Ctrl Pts',(2.11083834575196,313.238574056311,8.00877672769905));
#11287=CARTESIAN_POINT('Ctrl Pts',(-0.0327551936970299,313.376074056311,
8.));
#11288=CARTESIAN_POINT('Ctrl Pts',(-2.17634873314601,313.513574056311,7.99122327230096));
#11289=CARTESIAN_POINT('Ctrl Pts',(-4.02836682984751,313.651074056311,6.911825633427));
#11290=CARTESIAN_POINT('Ctrl Pts',(-5.88038492654901,313.788574056311,5.83242799455303));
#11291=CARTESIAN_POINT('Ctrl Pts',(-6.94458082712403,313.926074056311,3.9716331701525));
#11292=CARTESIAN_POINT('Ctrl Pts',(-8.00877672769905,314.063574056311,2.11083834575196));
#11293=CARTESIAN_POINT('Ctrl Pts',(-8.,314.201074056311,-0.0327551936970314));
#11294=CARTESIAN_POINT('Ctrl Pts',(-7.99122327230096,314.338574056311,-2.17634873314601));
#11295=CARTESIAN_POINT('Ctrl Pts',(-6.911825633427,314.476074056311,-4.02836682984751));
#11296=CARTESIAN_POINT('Ctrl Pts',(-5.83242799455303,314.613574056311,-5.88038492654901));
#11297=CARTESIAN_POINT('Ctrl Pts',(-3.97163317015249,314.751074056311,-6.94458082712403));
#11298=CARTESIAN_POINT('Ctrl Pts',(-2.11083834575195,314.888574056311,-8.00877672769905));
#11299=CARTESIAN_POINT('Ctrl Pts',(0.0327551936970309,315.026074056311,
-8.));
#11300=CARTESIAN_POINT('Ctrl Pts',(2.17634873314601,315.163574056311,-7.99122327230096));
#11301=CARTESIAN_POINT('Ctrl Pts',(4.02836682984751,315.301074056311,-6.911825633427));
#11302=CARTESIAN_POINT('Ctrl Pts',(5.88038492654901,315.438574056311,-5.83242799455303));
#11303=CARTESIAN_POINT('Ctrl Pts',(6.94458082712403,315.576074056311,-3.9716331701525));
#11304=CARTESIAN_POINT('Ctrl Pts',(8.00877672769905,315.713574056311,-2.11083834575195));
#11305=CARTESIAN_POINT('Ctrl Pts',(8.,315.851074056311,0.0327551936970304));
#11306=CARTESIAN_POINT('Ctrl Pts',(7.99122327230096,315.988574056311,2.17634873314601));
#11307=CARTESIAN_POINT('Ctrl Pts',(6.911825633427,316.126074056311,4.02836682984751));
#11308=CARTESIAN_POINT('Ctrl Pts',(5.83242799455304,316.263574056311,5.880384926549));
#11309=CARTESIAN_POINT('Ctrl Pts',(3.9716331701525,316.401074056311,6.94458082712403));
#11310=CARTESIAN_POINT('Ctrl Pts',(2.11083834575196,316.538574056311,8.00877672769905));
#11311=CARTESIAN_POINT('Ctrl Pts',(-0.0327551936970299,316.676074056311,
8.));
#11312=CARTESIAN_POINT('Ctrl Pts',(-2.17634873314601,316.813574056311,7.99122327230096));
#11313=CARTESIAN_POINT('Ctrl Pts',(-4.02836682984751,316.951074056311,6.911825633427));
#11314=CARTESIAN_POINT('Ctrl Pts',(-5.88038492654901,317.088574056311,5.83242799455303));
#11315=CARTESIAN_POINT('Ctrl Pts',(-6.94458082712403,317.226074056311,3.9716331701525));
#11316=CARTESIAN_POINT('Ctrl Pts',(-8.00877672769905,317.363574056311,2.11083834575196));
#11317=CARTESIAN_POINT('Ctrl Pts',(-8.,317.501074056311,-0.0327551936970314));
#11318=CARTESIAN_POINT('',(-8.,318.498925943689,0.0327551936971979));
#11319=CARTESIAN_POINT('Origin',(-8.,318.,8.32667268468867E-14));
#11320=CARTESIAN_POINT('',(-8.,285.498925943689,0.0327551936971979));
#11321=CARTESIAN_POINT('Ctrl Pts',(-8.,285.498925943689,0.0327551936971979));
#11322=CARTESIAN_POINT('Ctrl Pts',(-8.00877672769909,285.636425943689,-2.11083834575179));
#11323=CARTESIAN_POINT('Ctrl Pts',(-6.94458082712411,285.773925943689,-3.97163317015235));
#11324=CARTESIAN_POINT('Ctrl Pts',(-5.88038492654913,285.911425943689,-5.83242799455291));
#11325=CARTESIAN_POINT('Ctrl Pts',(-4.02836682984766,286.048925943689,-6.91182563342691));
#11326=CARTESIAN_POINT('Ctrl Pts',(-2.17634873314618,286.186425943689,-7.99122327230091));
#11327=CARTESIAN_POINT('Ctrl Pts',(-0.0327551936971984,286.323925943689,
-8.));
#11328=CARTESIAN_POINT('Ctrl Pts',(2.11083834575178,286.461425943689,-8.00877672769909));
#11329=CARTESIAN_POINT('Ctrl Pts',(3.97163317015235,286.598925943689,-6.94458082712411));
#11330=CARTESIAN_POINT('Ctrl Pts',(5.83242799455291,286.736425943689,-5.88038492654913));
#11331=CARTESIAN_POINT('Ctrl Pts',(6.91182563342691,286.873925943689,-4.02836682984766));
#11332=CARTESIAN_POINT('Ctrl Pts',(7.99122327230091,287.011425943689,-2.17634873314618));
#11333=CARTESIAN_POINT('Ctrl Pts',(8.,287.148925943689,-0.0327551936971989));
#11334=CARTESIAN_POINT('Ctrl Pts',(8.00877672769909,287.286425943689,2.11083834575178));
#11335=CARTESIAN_POINT('Ctrl Pts',(6.94458082712411,287.423925943689,3.97163317015235));
#11336=CARTESIAN_POINT('Ctrl Pts',(5.88038492654913,287.561425943689,5.83242799455291));
#11337=CARTESIAN_POINT('Ctrl Pts',(4.02836682984766,287.698925943689,6.91182563342691));
#11338=CARTESIAN_POINT('Ctrl Pts',(2.17634873314619,287.836425943689,7.99122327230091));
#11339=CARTESIAN_POINT('Ctrl Pts',(0.0327551936971994,287.973925943689,
8.));
#11340=CARTESIAN_POINT('Ctrl Pts',(-2.11083834575178,288.111425943689,8.00877672769909));
#11341=CARTESIAN_POINT('Ctrl Pts',(-3.97163317015234,288.248925943689,6.94458082712412));
#11342=CARTESIAN_POINT('Ctrl Pts',(-5.83242799455291,288.386425943689,5.88038492654913));
#11343=CARTESIAN_POINT('Ctrl Pts',(-6.91182563342691,288.523925943689,4.02836682984766));
#11344=CARTESIAN_POINT('Ctrl Pts',(-7.99122327230091,288.661425943689,2.17634873314619));
#11345=CARTESIAN_POINT('Ctrl Pts',(-8.,288.798925943689,0.0327551936971979));
#11346=CARTESIAN_POINT('Ctrl Pts',(-8.00877672769909,288.936425943689,-2.11083834575178));
#11347=CARTESIAN_POINT('Ctrl Pts',(-6.94458082712411,289.073925943689,-3.97163317015235));
#11348=CARTESIAN_POINT('Ctrl Pts',(-5.88038492654913,289.211425943689,-5.83242799455291));
#11349=CARTESIAN_POINT('Ctrl Pts',(-4.02836682984766,289.348925943689,-6.91182563342691));
#11350=CARTESIAN_POINT('Ctrl Pts',(-2.17634873314618,289.486425943689,-7.99122327230091));
#11351=CARTESIAN_POINT('Ctrl Pts',(-0.0327551936971984,289.623925943689,
-8.));
#11352=CARTESIAN_POINT('Ctrl Pts',(2.11083834575178,289.761425943689,-8.00877672769909));
#11353=CARTESIAN_POINT('Ctrl Pts',(3.97163317015235,289.898925943689,-6.94458082712411));
#11354=CARTESIAN_POINT('Ctrl Pts',(5.83242799455291,290.036425943689,-5.88038492654913));
#11355=CARTESIAN_POINT('Ctrl Pts',(6.91182563342691,290.173925943689,-4.02836682984766));
#11356=CARTESIAN_POINT('Ctrl Pts',(7.99122327230091,290.311425943689,-2.17634873314618));
#11357=CARTESIAN_POINT('Ctrl Pts',(8.,290.448925943689,-0.0327551936971989));
#11358=CARTESIAN_POINT('Ctrl Pts',(8.00877672769909,290.586425943689,2.11083834575178));
#11359=CARTESIAN_POINT('Ctrl Pts',(6.94458082712411,290.723925943689,3.97163317015235));
#11360=CARTESIAN_POINT('Ctrl Pts',(5.88038492654913,290.861425943689,5.83242799455291));
#11361=CARTESIAN_POINT('Ctrl Pts',(4.02836682984766,290.998925943689,6.91182563342691));
#11362=CARTESIAN_POINT('Ctrl Pts',(2.17634873314619,291.136425943689,7.99122327230091));
#11363=CARTESIAN_POINT('Ctrl Pts',(0.0327551936971994,291.273925943689,
8.));
#11364=CARTESIAN_POINT('Ctrl Pts',(-2.11083834575178,291.411425943689,8.00877672769909));
#11365=CARTESIAN_POINT('Ctrl Pts',(-3.97163317015234,291.548925943689,6.94458082712412));
#11366=CARTESIAN_POINT('Ctrl Pts',(-5.83242799455291,291.686425943689,5.88038492654913));
#11367=CARTESIAN_POINT('Ctrl Pts',(-6.91182563342691,291.823925943689,4.02836682984766));
#11368=CARTESIAN_POINT('Ctrl Pts',(-7.99122327230091,291.961425943689,2.17634873314619));
#11369=CARTESIAN_POINT('Ctrl Pts',(-8.,292.098925943689,0.0327551936971979));
#11370=CARTESIAN_POINT('Ctrl Pts',(-8.00877672769909,292.236425943689,-2.11083834575178));
#11371=CARTESIAN_POINT('Ctrl Pts',(-6.94458082712411,292.373925943689,-3.97163317015235));
#11372=CARTESIAN_POINT('Ctrl Pts',(-5.88038492654913,292.511425943689,-5.83242799455291));
#11373=CARTESIAN_POINT('Ctrl Pts',(-4.02836682984766,292.648925943689,-6.91182563342691));
#11374=CARTESIAN_POINT('Ctrl Pts',(-2.17634873314618,292.786425943689,-7.99122327230091));
#11375=CARTESIAN_POINT('Ctrl Pts',(-0.0327551936971984,292.923925943689,
-8.));
#11376=CARTESIAN_POINT('Ctrl Pts',(2.11083834575178,293.061425943689,-8.00877672769909));
#11377=CARTESIAN_POINT('Ctrl Pts',(3.97163317015235,293.198925943689,-6.94458082712411));
#11378=CARTESIAN_POINT('Ctrl Pts',(5.83242799455291,293.336425943689,-5.88038492654913));
#11379=CARTESIAN_POINT('Ctrl Pts',(6.91182563342691,293.473925943689,-4.02836682984766));
#11380=CARTESIAN_POINT('Ctrl Pts',(7.99122327230091,293.611425943689,-2.17634873314618));
#11381=CARTESIAN_POINT('Ctrl Pts',(8.,293.748925943689,-0.0327551936971989));
#11382=CARTESIAN_POINT('Ctrl Pts',(8.00877672769909,293.886425943689,2.11083834575178));
#11383=CARTESIAN_POINT('Ctrl Pts',(6.94458082712411,294.023925943689,3.97163317015235));
#11384=CARTESIAN_POINT('Ctrl Pts',(5.88038492654913,294.161425943689,5.83242799455291));
#11385=CARTESIAN_POINT('Ctrl Pts',(4.02836682984766,294.298925943689,6.91182563342691));
#11386=CARTESIAN_POINT('Ctrl Pts',(2.17634873314619,294.436425943689,7.99122327230091));
#11387=CARTESIAN_POINT('Ctrl Pts',(0.0327551936971994,294.573925943689,
8.));
#11388=CARTESIAN_POINT('Ctrl Pts',(-2.11083834575178,294.711425943689,8.00877672769909));
#11389=CARTESIAN_POINT('Ctrl Pts',(-3.97163317015234,294.848925943689,6.94458082712412));
#11390=CARTESIAN_POINT('Ctrl Pts',(-5.83242799455291,294.986425943689,5.88038492654913));
#11391=CARTESIAN_POINT('Ctrl Pts',(-6.91182563342691,295.123925943689,4.02836682984766));
#11392=CARTESIAN_POINT('Ctrl Pts',(-7.99122327230091,295.261425943689,2.17634873314619));
#11393=CARTESIAN_POINT('Ctrl Pts',(-8.,295.398925943689,0.0327551936971979));
#11394=CARTESIAN_POINT('Ctrl Pts',(-8.00877672769909,295.536425943689,-2.11083834575178));
#11395=CARTESIAN_POINT('Ctrl Pts',(-6.94458082712411,295.673925943689,-3.97163317015235));
#11396=CARTESIAN_POINT('Ctrl Pts',(-5.88038492654913,295.811425943689,-5.83242799455291));
#11397=CARTESIAN_POINT('Ctrl Pts',(-4.02836682984766,295.948925943689,-6.91182563342691));
#11398=CARTESIAN_POINT('Ctrl Pts',(-2.17634873314618,296.086425943689,-7.99122327230091));
#11399=CARTESIAN_POINT('Ctrl Pts',(-0.0327551936971984,296.223925943689,
-8.));
#11400=CARTESIAN_POINT('Ctrl Pts',(2.11083834575178,296.361425943689,-8.00877672769909));
#11401=CARTESIAN_POINT('Ctrl Pts',(3.97163317015235,296.498925943689,-6.94458082712411));
#11402=CARTESIAN_POINT('Ctrl Pts',(5.83242799455291,296.636425943689,-5.88038492654913));
#11403=CARTESIAN_POINT('Ctrl Pts',(6.91182563342691,296.773925943689,-4.02836682984766));
#11404=CARTESIAN_POINT('Ctrl Pts',(7.99122327230091,296.911425943689,-2.17634873314618));
#11405=CARTESIAN_POINT('Ctrl Pts',(8.,297.048925943689,-0.0327551936971989));
#11406=CARTESIAN_POINT('Ctrl Pts',(8.00877672769909,297.186425943689,2.11083834575178));
#11407=CARTESIAN_POINT('Ctrl Pts',(6.94458082712411,297.323925943689,3.97163317015235));
#11408=CARTESIAN_POINT('Ctrl Pts',(5.88038492654913,297.461425943689,5.83242799455291));
#11409=CARTESIAN_POINT('Ctrl Pts',(4.02836682984766,297.598925943689,6.91182563342691));
#11410=CARTESIAN_POINT('Ctrl Pts',(2.17634873314619,297.736425943689,7.99122327230091));
#11411=CARTESIAN_POINT('Ctrl Pts',(0.0327551936971994,297.873925943689,
8.));
#11412=CARTESIAN_POINT('Ctrl Pts',(-2.11083834575178,298.011425943689,8.00877672769909));
#11413=CARTESIAN_POINT('Ctrl Pts',(-3.97163317015234,298.148925943689,6.94458082712412));
#11414=CARTESIAN_POINT('Ctrl Pts',(-5.83242799455291,298.286425943689,5.88038492654913));
#11415=CARTESIAN_POINT('Ctrl Pts',(-6.91182563342691,298.423925943689,4.02836682984766));
#11416=CARTESIAN_POINT('Ctrl Pts',(-7.99122327230091,298.561425943689,2.17634873314619));
#11417=CARTESIAN_POINT('Ctrl Pts',(-8.,298.698925943689,0.0327551936971979));
#11418=CARTESIAN_POINT('Ctrl Pts',(-8.00877672769909,298.836425943689,-2.11083834575178));
#11419=CARTESIAN_POINT('Ctrl Pts',(-6.94458082712411,298.973925943689,-3.97163317015235));
#11420=CARTESIAN_POINT('Ctrl Pts',(-5.88038492654913,299.111425943689,-5.83242799455291));
#11421=CARTESIAN_POINT('Ctrl Pts',(-4.02836682984766,299.248925943689,-6.91182563342691));
#11422=CARTESIAN_POINT('Ctrl Pts',(-2.17634873314618,299.386425943689,-7.99122327230091));
#11423=CARTESIAN_POINT('Ctrl Pts',(-0.0327551936971984,299.523925943689,
-8.));
#11424=CARTESIAN_POINT('Ctrl Pts',(2.11083834575178,299.661425943689,-8.00877672769909));
#11425=CARTESIAN_POINT('Ctrl Pts',(3.97163317015235,299.798925943689,-6.94458082712411));
#11426=CARTESIAN_POINT('Ctrl Pts',(5.83242799455291,299.936425943689,-5.88038492654913));
#11427=CARTESIAN_POINT('Ctrl Pts',(6.91182563342691,300.073925943689,-4.02836682984766));
#11428=CARTESIAN_POINT('Ctrl Pts',(7.99122327230091,300.211425943689,-2.17634873314618));
#11429=CARTESIAN_POINT('Ctrl Pts',(8.,300.348925943689,-0.0327551936971989));
#11430=CARTESIAN_POINT('Ctrl Pts',(8.00877672769909,300.486425943689,2.11083834575178));
#11431=CARTESIAN_POINT('Ctrl Pts',(6.94458082712411,300.623925943689,3.97163317015235));
#11432=CARTESIAN_POINT('Ctrl Pts',(5.88038492654913,300.761425943689,5.83242799455291));
#11433=CARTESIAN_POINT('Ctrl Pts',(4.02836682984766,300.898925943689,6.91182563342691));
#11434=CARTESIAN_POINT('Ctrl Pts',(2.17634873314619,301.036425943689,7.99122327230091));
#11435=CARTESIAN_POINT('Ctrl Pts',(0.0327551936971994,301.173925943689,
8.));
#11436=CARTESIAN_POINT('Ctrl Pts',(-2.11083834575178,301.311425943689,8.00877672769909));
#11437=CARTESIAN_POINT('Ctrl Pts',(-3.97163317015234,301.448925943689,6.94458082712412));
#11438=CARTESIAN_POINT('Ctrl Pts',(-5.83242799455291,301.586425943689,5.88038492654913));
#11439=CARTESIAN_POINT('Ctrl Pts',(-6.91182563342691,301.723925943689,4.02836682984766));
#11440=CARTESIAN_POINT('Ctrl Pts',(-7.99122327230091,301.861425943689,2.17634873314619));
#11441=CARTESIAN_POINT('Ctrl Pts',(-8.,301.998925943689,0.0327551936971979));
#11442=CARTESIAN_POINT('Ctrl Pts',(-8.00877672769909,302.136425943689,-2.11083834575178));
#11443=CARTESIAN_POINT('Ctrl Pts',(-6.94458082712411,302.273925943689,-3.97163317015235));
#11444=CARTESIAN_POINT('Ctrl Pts',(-5.88038492654913,302.411425943689,-5.83242799455291));
#11445=CARTESIAN_POINT('Ctrl Pts',(-4.02836682984766,302.548925943689,-6.91182563342691));
#11446=CARTESIAN_POINT('Ctrl Pts',(-2.17634873314618,302.686425943689,-7.99122327230091));
#11447=CARTESIAN_POINT('Ctrl Pts',(-0.0327551936971984,302.823925943689,
-8.));
#11448=CARTESIAN_POINT('Ctrl Pts',(2.11083834575178,302.961425943689,-8.00877672769909));
#11449=CARTESIAN_POINT('Ctrl Pts',(3.97163317015235,303.098925943689,-6.94458082712411));
#11450=CARTESIAN_POINT('Ctrl Pts',(5.83242799455291,303.236425943689,-5.88038492654913));
#11451=CARTESIAN_POINT('Ctrl Pts',(6.91182563342691,303.373925943689,-4.02836682984766));
#11452=CARTESIAN_POINT('Ctrl Pts',(7.99122327230091,303.511425943689,-2.17634873314618));
#11453=CARTESIAN_POINT('Ctrl Pts',(8.,303.648925943689,-0.0327551936971989));
#11454=CARTESIAN_POINT('Ctrl Pts',(8.00877672769909,303.786425943689,2.11083834575178));
#11455=CARTESIAN_POINT('Ctrl Pts',(6.94458082712411,303.923925943689,3.97163317015235));
#11456=CARTESIAN_POINT('Ctrl Pts',(5.88038492654913,304.061425943689,5.83242799455291));
#11457=CARTESIAN_POINT('Ctrl Pts',(4.02836682984766,304.198925943689,6.91182563342691));
#11458=CARTESIAN_POINT('Ctrl Pts',(2.17634873314619,304.336425943689,7.99122327230091));
#11459=CARTESIAN_POINT('Ctrl Pts',(0.0327551936971994,304.473925943689,
8.));
#11460=CARTESIAN_POINT('Ctrl Pts',(-2.11083834575178,304.611425943689,8.00877672769909));
#11461=CARTESIAN_POINT('Ctrl Pts',(-3.97163317015234,304.748925943689,6.94458082712412));
#11462=CARTESIAN_POINT('Ctrl Pts',(-5.83242799455291,304.886425943689,5.88038492654913));
#11463=CARTESIAN_POINT('Ctrl Pts',(-6.91182563342691,305.023925943689,4.02836682984766));
#11464=CARTESIAN_POINT('Ctrl Pts',(-7.99122327230091,305.161425943689,2.17634873314619));
#11465=CARTESIAN_POINT('Ctrl Pts',(-8.,305.298925943689,0.0327551936971979));
#11466=CARTESIAN_POINT('Ctrl Pts',(-8.00877672769909,305.436425943689,-2.11083834575178));
#11467=CARTESIAN_POINT('Ctrl Pts',(-6.94458082712411,305.573925943689,-3.97163317015235));
#11468=CARTESIAN_POINT('Ctrl Pts',(-5.88038492654913,305.711425943689,-5.83242799455291));
#11469=CARTESIAN_POINT('Ctrl Pts',(-4.02836682984766,305.848925943689,-6.91182563342691));
#11470=CARTESIAN_POINT('Ctrl Pts',(-2.17634873314618,305.986425943689,-7.99122327230091));
#11471=CARTESIAN_POINT('Ctrl Pts',(-0.0327551936971984,306.123925943689,
-8.));
#11472=CARTESIAN_POINT('Ctrl Pts',(2.11083834575178,306.261425943689,-8.00877672769909));
#11473=CARTESIAN_POINT('Ctrl Pts',(3.97163317015235,306.398925943689,-6.94458082712411));
#11474=CARTESIAN_POINT('Ctrl Pts',(5.83242799455291,306.536425943689,-5.88038492654913));
#11475=CARTESIAN_POINT('Ctrl Pts',(6.91182563342691,306.673925943689,-4.02836682984766));
#11476=CARTESIAN_POINT('Ctrl Pts',(7.99122327230091,306.811425943689,-2.17634873314618));
#11477=CARTESIAN_POINT('Ctrl Pts',(8.,306.948925943689,-0.0327551936971989));
#11478=CARTESIAN_POINT('Ctrl Pts',(8.00877672769909,307.086425943689,2.11083834575178));
#11479=CARTESIAN_POINT('Ctrl Pts',(6.94458082712411,307.223925943689,3.97163317015235));
#11480=CARTESIAN_POINT('Ctrl Pts',(5.88038492654913,307.361425943689,5.83242799455291));
#11481=CARTESIAN_POINT('Ctrl Pts',(4.02836682984766,307.498925943689,6.91182563342691));
#11482=CARTESIAN_POINT('Ctrl Pts',(2.17634873314619,307.636425943689,7.99122327230091));
#11483=CARTESIAN_POINT('Ctrl Pts',(0.0327551936971994,307.773925943689,
8.));
#11484=CARTESIAN_POINT('Ctrl Pts',(-2.11083834575178,307.911425943689,8.00877672769909));
#11485=CARTESIAN_POINT('Ctrl Pts',(-3.97163317015234,308.048925943689,6.94458082712412));
#11486=CARTESIAN_POINT('Ctrl Pts',(-5.83242799455291,308.186425943689,5.88038492654913));
#11487=CARTESIAN_POINT('Ctrl Pts',(-6.91182563342691,308.323925943689,4.02836682984766));
#11488=CARTESIAN_POINT('Ctrl Pts',(-7.99122327230091,308.461425943689,2.17634873314619));
#11489=CARTESIAN_POINT('Ctrl Pts',(-8.,308.598925943689,0.0327551936971979));
#11490=CARTESIAN_POINT('Ctrl Pts',(-8.00877672769909,308.736425943689,-2.11083834575178));
#11491=CARTESIAN_POINT('Ctrl Pts',(-6.94458082712411,308.873925943689,-3.97163317015235));
#11492=CARTESIAN_POINT('Ctrl Pts',(-5.88038492654913,309.011425943689,-5.83242799455291));
#11493=CARTESIAN_POINT('Ctrl Pts',(-4.02836682984766,309.148925943689,-6.91182563342691));
#11494=CARTESIAN_POINT('Ctrl Pts',(-2.17634873314618,309.286425943689,-7.99122327230091));
#11495=CARTESIAN_POINT('Ctrl Pts',(-0.0327551936971984,309.423925943689,
-8.));
#11496=CARTESIAN_POINT('Ctrl Pts',(2.11083834575178,309.561425943689,-8.00877672769909));
#11497=CARTESIAN_POINT('Ctrl Pts',(3.97163317015235,309.698925943689,-6.94458082712411));
#11498=CARTESIAN_POINT('Ctrl Pts',(5.83242799455291,309.836425943689,-5.88038492654913));
#11499=CARTESIAN_POINT('Ctrl Pts',(6.91182563342691,309.973925943689,-4.02836682984766));
#11500=CARTESIAN_POINT('Ctrl Pts',(7.99122327230091,310.111425943689,-2.17634873314618));
#11501=CARTESIAN_POINT('Ctrl Pts',(8.,310.248925943689,-0.0327551936971989));
#11502=CARTESIAN_POINT('Ctrl Pts',(8.00877672769909,310.386425943689,2.11083834575178));
#11503=CARTESIAN_POINT('Ctrl Pts',(6.94458082712411,310.523925943689,3.97163317015235));
#11504=CARTESIAN_POINT('Ctrl Pts',(5.88038492654913,310.661425943689,5.83242799455291));
#11505=CARTESIAN_POINT('Ctrl Pts',(4.02836682984766,310.798925943689,6.91182563342691));
#11506=CARTESIAN_POINT('Ctrl Pts',(2.17634873314619,310.936425943689,7.99122327230091));
#11507=CARTESIAN_POINT('Ctrl Pts',(0.0327551936971994,311.073925943689,
8.));
#11508=CARTESIAN_POINT('Ctrl Pts',(-2.11083834575178,311.211425943689,8.00877672769909));
#11509=CARTESIAN_POINT('Ctrl Pts',(-3.97163317015234,311.348925943689,6.94458082712412));
#11510=CARTESIAN_POINT('Ctrl Pts',(-5.83242799455291,311.486425943689,5.88038492654913));
#11511=CARTESIAN_POINT('Ctrl Pts',(-6.91182563342691,311.623925943689,4.02836682984766));
#11512=CARTESIAN_POINT('Ctrl Pts',(-7.99122327230091,311.761425943689,2.17634873314619));
#11513=CARTESIAN_POINT('Ctrl Pts',(-8.,311.898925943689,0.0327551936971979));
#11514=CARTESIAN_POINT('Ctrl Pts',(-8.00877672769909,312.036425943689,-2.11083834575178));
#11515=CARTESIAN_POINT('Ctrl Pts',(-6.94458082712411,312.173925943689,-3.97163317015235));
#11516=CARTESIAN_POINT('Ctrl Pts',(-5.88038492654913,312.311425943689,-5.83242799455291));
#11517=CARTESIAN_POINT('Ctrl Pts',(-4.02836682984766,312.448925943689,-6.91182563342691));
#11518=CARTESIAN_POINT('Ctrl Pts',(-2.17634873314618,312.586425943689,-7.99122327230091));
#11519=CARTESIAN_POINT('Ctrl Pts',(-0.0327551936971984,312.723925943689,
-8.));
#11520=CARTESIAN_POINT('Ctrl Pts',(2.11083834575178,312.861425943689,-8.00877672769909));
#11521=CARTESIAN_POINT('Ctrl Pts',(3.97163317015235,312.998925943689,-6.94458082712411));
#11522=CARTESIAN_POINT('Ctrl Pts',(5.83242799455291,313.136425943689,-5.88038492654913));
#11523=CARTESIAN_POINT('Ctrl Pts',(6.91182563342691,313.273925943689,-4.02836682984766));
#11524=CARTESIAN_POINT('Ctrl Pts',(7.99122327230091,313.411425943689,-2.17634873314618));
#11525=CARTESIAN_POINT('Ctrl Pts',(8.,313.548925943689,-0.0327551936971989));
#11526=CARTESIAN_POINT('Ctrl Pts',(8.00877672769909,313.686425943689,2.11083834575178));
#11527=CARTESIAN_POINT('Ctrl Pts',(6.94458082712411,313.823925943689,3.97163317015235));
#11528=CARTESIAN_POINT('Ctrl Pts',(5.88038492654913,313.961425943689,5.83242799455291));
#11529=CARTESIAN_POINT('Ctrl Pts',(4.02836682984766,314.098925943689,6.91182563342691));
#11530=CARTESIAN_POINT('Ctrl Pts',(2.17634873314619,314.236425943689,7.99122327230091));
#11531=CARTESIAN_POINT('Ctrl Pts',(0.0327551936971994,314.373925943689,
8.));
#11532=CARTESIAN_POINT('Ctrl Pts',(-2.11083834575178,314.511425943689,8.00877672769909));
#11533=CARTESIAN_POINT('Ctrl Pts',(-3.97163317015234,314.648925943689,6.94458082712412));
#11534=CARTESIAN_POINT('Ctrl Pts',(-5.83242799455291,314.786425943689,5.88038492654913));
#11535=CARTESIAN_POINT('Ctrl Pts',(-6.91182563342691,314.923925943689,4.02836682984766));
#11536=CARTESIAN_POINT('Ctrl Pts',(-7.99122327230091,315.061425943689,2.17634873314619));
#11537=CARTESIAN_POINT('Ctrl Pts',(-8.,315.198925943689,0.0327551936971979));
#11538=CARTESIAN_POINT('Ctrl Pts',(-8.00877672769909,315.336425943689,-2.11083834575178));
#11539=CARTESIAN_POINT('Ctrl Pts',(-6.94458082712411,315.473925943689,-3.97163317015235));
#11540=CARTESIAN_POINT('Ctrl Pts',(-5.88038492654913,315.611425943689,-5.83242799455291));
#11541=CARTESIAN_POINT('Ctrl Pts',(-4.02836682984766,315.748925943689,-6.91182563342691));
#11542=CARTESIAN_POINT('Ctrl Pts',(-2.17634873314618,315.886425943689,-7.99122327230091));
#11543=CARTESIAN_POINT('Ctrl Pts',(-0.0327551936971984,316.023925943689,
-8.));
#11544=CARTESIAN_POINT('Ctrl Pts',(2.11083834575178,316.161425943689,-8.00877672769909));
#11545=CARTESIAN_POINT('Ctrl Pts',(3.97163317015235,316.298925943689,-6.94458082712411));
#11546=CARTESIAN_POINT('Ctrl Pts',(5.83242799455291,316.436425943689,-5.88038492654913));
#11547=CARTESIAN_POINT('Ctrl Pts',(6.91182563342691,316.573925943689,-4.02836682984766));
#11548=CARTESIAN_POINT('Ctrl Pts',(7.99122327230091,316.711425943689,-2.17634873314618));
#11549=CARTESIAN_POINT('Ctrl Pts',(8.,316.848925943689,-0.0327551936971989));
#11550=CARTESIAN_POINT('Ctrl Pts',(8.00877672769909,316.986425943689,2.11083834575178));
#11551=CARTESIAN_POINT('Ctrl Pts',(6.94458082712411,317.123925943689,3.97163317015235));
#11552=CARTESIAN_POINT('Ctrl Pts',(5.88038492654913,317.261425943689,5.83242799455291));
#11553=CARTESIAN_POINT('Ctrl Pts',(4.02836682984766,317.398925943689,6.91182563342691));
#11554=CARTESIAN_POINT('Ctrl Pts',(2.17634873314619,317.536425943689,7.99122327230091));
#11555=CARTESIAN_POINT('Ctrl Pts',(0.0327551936971994,317.673925943689,
8.));
#11556=CARTESIAN_POINT('Ctrl Pts',(-2.11083834575178,317.811425943689,8.00877672769909));
#11557=CARTESIAN_POINT('Ctrl Pts',(-3.97163317015234,317.948925943689,6.94458082712412));
#11558=CARTESIAN_POINT('Ctrl Pts',(-5.83242799455291,318.086425943689,5.88038492654913));
#11559=CARTESIAN_POINT('Ctrl Pts',(-6.91182563342691,318.223925943689,4.02836682984766));
#11560=CARTESIAN_POINT('Ctrl Pts',(-7.99122327230091,318.361425943689,2.17634873314619));
#11561=CARTESIAN_POINT('Ctrl Pts',(-8.,318.498925943689,0.0327551936971979));
#11562=CARTESIAN_POINT('Origin',(-8.,285.,8.32667268468867E-14));
#11563=CARTESIAN_POINT('Origin',(-8.,284.501074056311,-0.0327551936970314));
#11564=CARTESIAN_POINT('',(-8.49999999999999,285.,8.09585094317261E-14));
#11565=CARTESIAN_POINT('Origin',(-8.,285.,8.32667268468867E-14));
#11566=CARTESIAN_POINT('',(-8.,285.,7.59754672369217E-14));
#11567=CARTESIAN_POINT('Ctrl Pts',(-8.,285.498925943689,0.0327551936971979));
#11568=CARTESIAN_POINT('Ctrl Pts',(-8.00877672769909,285.636425943689,-2.11083834575178));
#11569=CARTESIAN_POINT('Ctrl Pts',(-6.94458082712411,285.773925943689,-3.97163317015235));
#11570=CARTESIAN_POINT('Ctrl Pts',(-5.88038492654913,285.911425943689,-5.83242799455291));
#11571=CARTESIAN_POINT('Ctrl Pts',(-4.02836682984766,286.048925943689,-6.91182563342691));
#11572=CARTESIAN_POINT('Ctrl Pts',(-2.17634873314618,286.186425943689,-7.99122327230091));
#11573=CARTESIAN_POINT('Ctrl Pts',(-0.0327551936971984,286.323925943689,
-8.));
#11574=CARTESIAN_POINT('Ctrl Pts',(2.11083834575178,286.461425943689,-8.00877672769909));
#11575=CARTESIAN_POINT('Ctrl Pts',(3.97163317015235,286.598925943689,-6.94458082712411));
#11576=CARTESIAN_POINT('Ctrl Pts',(5.83242799455291,286.736425943689,-5.88038492654913));
#11577=CARTESIAN_POINT('Ctrl Pts',(6.91182563342691,286.873925943689,-4.02836682984766));
#11578=CARTESIAN_POINT('Ctrl Pts',(7.99122327230091,287.011425943689,-2.17634873314618));
#11579=CARTESIAN_POINT('Ctrl Pts',(8.,287.148925943689,-0.0327551936971989));
#11580=CARTESIAN_POINT('Ctrl Pts',(8.00877672769909,287.286425943689,2.11083834575178));
#11581=CARTESIAN_POINT('Ctrl Pts',(6.94458082712411,287.423925943689,3.97163317015235));
#11582=CARTESIAN_POINT('Ctrl Pts',(5.88038492654913,287.561425943689,5.83242799455291));
#11583=CARTESIAN_POINT('Ctrl Pts',(4.02836682984766,287.698925943689,6.91182563342691));
#11584=CARTESIAN_POINT('Ctrl Pts',(2.17634873314619,287.836425943689,7.99122327230091));
#11585=CARTESIAN_POINT('Ctrl Pts',(0.0327551936971994,287.973925943689,
8.));
#11586=CARTESIAN_POINT('Ctrl Pts',(-2.11083834575178,288.111425943689,8.00877672769909));
#11587=CARTESIAN_POINT('Ctrl Pts',(-3.97163317015234,288.248925943689,6.94458082712412));
#11588=CARTESIAN_POINT('Ctrl Pts',(-5.83242799455291,288.386425943689,5.88038492654913));
#11589=CARTESIAN_POINT('Ctrl Pts',(-6.91182563342691,288.523925943689,4.02836682984766));
#11590=CARTESIAN_POINT('Ctrl Pts',(-7.99122327230091,288.661425943689,2.17634873314619));
#11591=CARTESIAN_POINT('Ctrl Pts',(-8.,288.798925943689,0.0327551936971979));
#11592=CARTESIAN_POINT('Ctrl Pts',(-8.00877672769909,288.936425943689,-2.11083834575178));
#11593=CARTESIAN_POINT('Ctrl Pts',(-6.94458082712411,289.073925943689,-3.97163317015235));
#11594=CARTESIAN_POINT('Ctrl Pts',(-5.88038492654913,289.211425943689,-5.83242799455291));
#11595=CARTESIAN_POINT('Ctrl Pts',(-4.02836682984766,289.348925943689,-6.91182563342691));
#11596=CARTESIAN_POINT('Ctrl Pts',(-2.17634873314618,289.486425943689,-7.99122327230091));
#11597=CARTESIAN_POINT('Ctrl Pts',(-0.0327551936971984,289.623925943689,
-8.));
#11598=CARTESIAN_POINT('Ctrl Pts',(2.11083834575178,289.761425943689,-8.00877672769909));
#11599=CARTESIAN_POINT('Ctrl Pts',(3.97163317015235,289.898925943689,-6.94458082712411));
#11600=CARTESIAN_POINT('Ctrl Pts',(5.83242799455291,290.036425943689,-5.88038492654913));
#11601=CARTESIAN_POINT('Ctrl Pts',(6.91182563342691,290.173925943689,-4.02836682984766));
#11602=CARTESIAN_POINT('Ctrl Pts',(7.99122327230091,290.311425943689,-2.17634873314618));
#11603=CARTESIAN_POINT('Ctrl Pts',(8.,290.448925943689,-0.0327551936971989));
#11604=CARTESIAN_POINT('Ctrl Pts',(8.00877672769909,290.586425943689,2.11083834575178));
#11605=CARTESIAN_POINT('Ctrl Pts',(6.94458082712411,290.723925943689,3.97163317015235));
#11606=CARTESIAN_POINT('Ctrl Pts',(5.88038492654913,290.861425943689,5.83242799455291));
#11607=CARTESIAN_POINT('Ctrl Pts',(4.02836682984766,290.998925943689,6.91182563342691));
#11608=CARTESIAN_POINT('Ctrl Pts',(2.17634873314619,291.136425943689,7.99122327230091));
#11609=CARTESIAN_POINT('Ctrl Pts',(0.0327551936971994,291.273925943689,
8.));
#11610=CARTESIAN_POINT('Ctrl Pts',(-2.11083834575178,291.411425943689,8.00877672769909));
#11611=CARTESIAN_POINT('Ctrl Pts',(-3.97163317015234,291.548925943689,6.94458082712412));
#11612=CARTESIAN_POINT('Ctrl Pts',(-5.83242799455291,291.686425943689,5.88038492654913));
#11613=CARTESIAN_POINT('Ctrl Pts',(-6.91182563342691,291.823925943689,4.02836682984766));
#11614=CARTESIAN_POINT('Ctrl Pts',(-7.99122327230091,291.961425943689,2.17634873314619));
#11615=CARTESIAN_POINT('Ctrl Pts',(-8.,292.098925943689,0.0327551936971979));
#11616=CARTESIAN_POINT('Ctrl Pts',(-8.00877672769909,292.236425943689,-2.11083834575178));
#11617=CARTESIAN_POINT('Ctrl Pts',(-6.94458082712411,292.373925943689,-3.97163317015235));
#11618=CARTESIAN_POINT('Ctrl Pts',(-5.88038492654913,292.511425943689,-5.83242799455291));
#11619=CARTESIAN_POINT('Ctrl Pts',(-4.02836682984766,292.648925943689,-6.91182563342691));
#11620=CARTESIAN_POINT('Ctrl Pts',(-2.17634873314618,292.786425943689,-7.99122327230091));
#11621=CARTESIAN_POINT('Ctrl Pts',(-0.0327551936971984,292.923925943689,
-8.));
#11622=CARTESIAN_POINT('Ctrl Pts',(2.11083834575178,293.061425943689,-8.00877672769909));
#11623=CARTESIAN_POINT('Ctrl Pts',(3.97163317015235,293.198925943689,-6.94458082712411));
#11624=CARTESIAN_POINT('Ctrl Pts',(5.83242799455291,293.336425943689,-5.88038492654913));
#11625=CARTESIAN_POINT('Ctrl Pts',(6.91182563342691,293.473925943689,-4.02836682984766));
#11626=CARTESIAN_POINT('Ctrl Pts',(7.99122327230091,293.611425943689,-2.17634873314618));
#11627=CARTESIAN_POINT('Ctrl Pts',(8.,293.748925943689,-0.0327551936971989));
#11628=CARTESIAN_POINT('Ctrl Pts',(8.00877672769909,293.886425943689,2.11083834575178));
#11629=CARTESIAN_POINT('Ctrl Pts',(6.94458082712411,294.023925943689,3.97163317015235));
#11630=CARTESIAN_POINT('Ctrl Pts',(5.88038492654913,294.161425943689,5.83242799455291));
#11631=CARTESIAN_POINT('Ctrl Pts',(4.02836682984766,294.298925943689,6.91182563342691));
#11632=CARTESIAN_POINT('Ctrl Pts',(2.17634873314619,294.436425943689,7.99122327230091));
#11633=CARTESIAN_POINT('Ctrl Pts',(0.0327551936971994,294.573925943689,
8.));
#11634=CARTESIAN_POINT('Ctrl Pts',(-2.11083834575178,294.711425943689,8.00877672769909));
#11635=CARTESIAN_POINT('Ctrl Pts',(-3.97163317015234,294.848925943689,6.94458082712412));
#11636=CARTESIAN_POINT('Ctrl Pts',(-5.83242799455291,294.986425943689,5.88038492654913));
#11637=CARTESIAN_POINT('Ctrl Pts',(-6.91182563342691,295.123925943689,4.02836682984766));
#11638=CARTESIAN_POINT('Ctrl Pts',(-7.99122327230091,295.261425943689,2.17634873314619));
#11639=CARTESIAN_POINT('Ctrl Pts',(-8.,295.398925943689,0.0327551936971979));
#11640=CARTESIAN_POINT('Ctrl Pts',(-8.00877672769909,295.536425943689,-2.11083834575178));
#11641=CARTESIAN_POINT('Ctrl Pts',(-6.94458082712411,295.673925943689,-3.97163317015235));
#11642=CARTESIAN_POINT('Ctrl Pts',(-5.88038492654913,295.811425943689,-5.83242799455291));
#11643=CARTESIAN_POINT('Ctrl Pts',(-4.02836682984766,295.948925943689,-6.91182563342691));
#11644=CARTESIAN_POINT('Ctrl Pts',(-2.17634873314618,296.086425943689,-7.99122327230091));
#11645=CARTESIAN_POINT('Ctrl Pts',(-0.0327551936971984,296.223925943689,
-8.));
#11646=CARTESIAN_POINT('Ctrl Pts',(2.11083834575178,296.361425943689,-8.00877672769909));
#11647=CARTESIAN_POINT('Ctrl Pts',(3.97163317015235,296.498925943689,-6.94458082712411));
#11648=CARTESIAN_POINT('Ctrl Pts',(5.83242799455291,296.636425943689,-5.88038492654913));
#11649=CARTESIAN_POINT('Ctrl Pts',(6.91182563342691,296.773925943689,-4.02836682984766));
#11650=CARTESIAN_POINT('Ctrl Pts',(7.99122327230091,296.911425943689,-2.17634873314618));
#11651=CARTESIAN_POINT('Ctrl Pts',(8.,297.048925943689,-0.0327551936971989));
#11652=CARTESIAN_POINT('Ctrl Pts',(8.00877672769909,297.186425943689,2.11083834575178));
#11653=CARTESIAN_POINT('Ctrl Pts',(6.94458082712411,297.323925943689,3.97163317015235));
#11654=CARTESIAN_POINT('Ctrl Pts',(5.88038492654913,297.461425943689,5.83242799455291));
#11655=CARTESIAN_POINT('Ctrl Pts',(4.02836682984766,297.598925943689,6.91182563342691));
#11656=CARTESIAN_POINT('Ctrl Pts',(2.17634873314619,297.736425943689,7.99122327230091));
#11657=CARTESIAN_POINT('Ctrl Pts',(0.0327551936971994,297.873925943689,
8.));
#11658=CARTESIAN_POINT('Ctrl Pts',(-2.11083834575178,298.011425943689,8.00877672769909));
#11659=CARTESIAN_POINT('Ctrl Pts',(-3.97163317015234,298.148925943689,6.94458082712412));
#11660=CARTESIAN_POINT('Ctrl Pts',(-5.83242799455291,298.286425943689,5.88038492654913));
#11661=CARTESIAN_POINT('Ctrl Pts',(-6.91182563342691,298.423925943689,4.02836682984766));
#11662=CARTESIAN_POINT('Ctrl Pts',(-7.99122327230091,298.561425943689,2.17634873314619));
#11663=CARTESIAN_POINT('Ctrl Pts',(-8.,298.698925943689,0.0327551936971979));
#11664=CARTESIAN_POINT('Ctrl Pts',(-8.00877672769909,298.836425943689,-2.11083834575178));
#11665=CARTESIAN_POINT('Ctrl Pts',(-6.94458082712411,298.973925943689,-3.97163317015235));
#11666=CARTESIAN_POINT('Ctrl Pts',(-5.88038492654913,299.111425943689,-5.83242799455291));
#11667=CARTESIAN_POINT('Ctrl Pts',(-4.02836682984766,299.248925943689,-6.91182563342691));
#11668=CARTESIAN_POINT('Ctrl Pts',(-2.17634873314618,299.386425943689,-7.99122327230091));
#11669=CARTESIAN_POINT('Ctrl Pts',(-0.0327551936971984,299.523925943689,
-8.));
#11670=CARTESIAN_POINT('Ctrl Pts',(2.11083834575178,299.661425943689,-8.00877672769909));
#11671=CARTESIAN_POINT('Ctrl Pts',(3.97163317015235,299.798925943689,-6.94458082712411));
#11672=CARTESIAN_POINT('Ctrl Pts',(5.83242799455291,299.936425943689,-5.88038492654913));
#11673=CARTESIAN_POINT('Ctrl Pts',(6.91182563342691,300.073925943689,-4.02836682984766));
#11674=CARTESIAN_POINT('Ctrl Pts',(7.99122327230091,300.211425943689,-2.17634873314618));
#11675=CARTESIAN_POINT('Ctrl Pts',(8.,300.348925943689,-0.0327551936971989));
#11676=CARTESIAN_POINT('Ctrl Pts',(8.00877672769909,300.486425943689,2.11083834575178));
#11677=CARTESIAN_POINT('Ctrl Pts',(6.94458082712411,300.623925943689,3.97163317015235));
#11678=CARTESIAN_POINT('Ctrl Pts',(5.88038492654913,300.761425943689,5.83242799455291));
#11679=CARTESIAN_POINT('Ctrl Pts',(4.02836682984766,300.898925943689,6.91182563342691));
#11680=CARTESIAN_POINT('Ctrl Pts',(2.17634873314619,301.036425943689,7.99122327230091));
#11681=CARTESIAN_POINT('Ctrl Pts',(0.0327551936971994,301.173925943689,
8.));
#11682=CARTESIAN_POINT('Ctrl Pts',(-2.11083834575178,301.311425943689,8.00877672769909));
#11683=CARTESIAN_POINT('Ctrl Pts',(-3.97163317015234,301.448925943689,6.94458082712412));
#11684=CARTESIAN_POINT('Ctrl Pts',(-5.83242799455291,301.586425943689,5.88038492654913));
#11685=CARTESIAN_POINT('Ctrl Pts',(-6.91182563342691,301.723925943689,4.02836682984766));
#11686=CARTESIAN_POINT('Ctrl Pts',(-7.99122327230091,301.861425943689,2.17634873314619));
#11687=CARTESIAN_POINT('Ctrl Pts',(-8.,301.998925943689,0.0327551936971979));
#11688=CARTESIAN_POINT('Ctrl Pts',(-8.00877672769909,302.136425943689,-2.11083834575178));
#11689=CARTESIAN_POINT('Ctrl Pts',(-6.94458082712411,302.273925943689,-3.97163317015235));
#11690=CARTESIAN_POINT('Ctrl Pts',(-5.88038492654913,302.411425943689,-5.83242799455291));
#11691=CARTESIAN_POINT('Ctrl Pts',(-4.02836682984766,302.548925943689,-6.91182563342691));
#11692=CARTESIAN_POINT('Ctrl Pts',(-2.17634873314618,302.686425943689,-7.99122327230091));
#11693=CARTESIAN_POINT('Ctrl Pts',(-0.0327551936971984,302.823925943689,
-8.));
#11694=CARTESIAN_POINT('Ctrl Pts',(2.11083834575178,302.961425943689,-8.00877672769909));
#11695=CARTESIAN_POINT('Ctrl Pts',(3.97163317015235,303.098925943689,-6.94458082712411));
#11696=CARTESIAN_POINT('Ctrl Pts',(5.83242799455291,303.236425943689,-5.88038492654913));
#11697=CARTESIAN_POINT('Ctrl Pts',(6.91182563342691,303.373925943689,-4.02836682984766));
#11698=CARTESIAN_POINT('Ctrl Pts',(7.99122327230091,303.511425943689,-2.17634873314618));
#11699=CARTESIAN_POINT('Ctrl Pts',(8.,303.648925943689,-0.0327551936971989));
#11700=CARTESIAN_POINT('Ctrl Pts',(8.00877672769909,303.786425943689,2.11083834575178));
#11701=CARTESIAN_POINT('Ctrl Pts',(6.94458082712411,303.923925943689,3.97163317015235));
#11702=CARTESIAN_POINT('Ctrl Pts',(5.88038492654913,304.061425943689,5.83242799455291));
#11703=CARTESIAN_POINT('Ctrl Pts',(4.02836682984766,304.198925943689,6.91182563342691));
#11704=CARTESIAN_POINT('Ctrl Pts',(2.17634873314619,304.336425943689,7.99122327230091));
#11705=CARTESIAN_POINT('Ctrl Pts',(0.0327551936971994,304.473925943689,
8.));
#11706=CARTESIAN_POINT('Ctrl Pts',(-2.11083834575178,304.611425943689,8.00877672769909));
#11707=CARTESIAN_POINT('Ctrl Pts',(-3.97163317015234,304.748925943689,6.94458082712412));
#11708=CARTESIAN_POINT('Ctrl Pts',(-5.83242799455291,304.886425943689,5.88038492654913));
#11709=CARTESIAN_POINT('Ctrl Pts',(-6.91182563342691,305.023925943689,4.02836682984766));
#11710=CARTESIAN_POINT('Ctrl Pts',(-7.99122327230091,305.161425943689,2.17634873314619));
#11711=CARTESIAN_POINT('Ctrl Pts',(-8.,305.298925943689,0.0327551936971979));
#11712=CARTESIAN_POINT('Ctrl Pts',(-8.00877672769909,305.436425943689,-2.11083834575178));
#11713=CARTESIAN_POINT('Ctrl Pts',(-6.94458082712411,305.573925943689,-3.97163317015235));
#11714=CARTESIAN_POINT('Ctrl Pts',(-5.88038492654913,305.711425943689,-5.83242799455291));
#11715=CARTESIAN_POINT('Ctrl Pts',(-4.02836682984766,305.848925943689,-6.91182563342691));
#11716=CARTESIAN_POINT('Ctrl Pts',(-2.17634873314618,305.986425943689,-7.99122327230091));
#11717=CARTESIAN_POINT('Ctrl Pts',(-0.0327551936971984,306.123925943689,
-8.));
#11718=CARTESIAN_POINT('Ctrl Pts',(2.11083834575178,306.261425943689,-8.00877672769909));
#11719=CARTESIAN_POINT('Ctrl Pts',(3.97163317015235,306.398925943689,-6.94458082712411));
#11720=CARTESIAN_POINT('Ctrl Pts',(5.83242799455291,306.536425943689,-5.88038492654913));
#11721=CARTESIAN_POINT('Ctrl Pts',(6.91182563342691,306.673925943689,-4.02836682984766));
#11722=CARTESIAN_POINT('Ctrl Pts',(7.99122327230091,306.811425943689,-2.17634873314618));
#11723=CARTESIAN_POINT('Ctrl Pts',(8.,306.948925943689,-0.0327551936971989));
#11724=CARTESIAN_POINT('Ctrl Pts',(8.00877672769909,307.086425943689,2.11083834575178));
#11725=CARTESIAN_POINT('Ctrl Pts',(6.94458082712411,307.223925943689,3.97163317015235));
#11726=CARTESIAN_POINT('Ctrl Pts',(5.88038492654913,307.361425943689,5.83242799455291));
#11727=CARTESIAN_POINT('Ctrl Pts',(4.02836682984766,307.498925943689,6.91182563342691));
#11728=CARTESIAN_POINT('Ctrl Pts',(2.17634873314619,307.636425943689,7.99122327230091));
#11729=CARTESIAN_POINT('Ctrl Pts',(0.0327551936971994,307.773925943689,
8.));
#11730=CARTESIAN_POINT('Ctrl Pts',(-2.11083834575178,307.911425943689,8.00877672769909));
#11731=CARTESIAN_POINT('Ctrl Pts',(-3.97163317015234,308.048925943689,6.94458082712412));
#11732=CARTESIAN_POINT('Ctrl Pts',(-5.83242799455291,308.186425943689,5.88038492654913));
#11733=CARTESIAN_POINT('Ctrl Pts',(-6.91182563342691,308.323925943689,4.02836682984766));
#11734=CARTESIAN_POINT('Ctrl Pts',(-7.99122327230091,308.461425943689,2.17634873314619));
#11735=CARTESIAN_POINT('Ctrl Pts',(-8.,308.598925943689,0.0327551936971979));
#11736=CARTESIAN_POINT('Ctrl Pts',(-8.00877672769909,308.736425943689,-2.11083834575178));
#11737=CARTESIAN_POINT('Ctrl Pts',(-6.94458082712411,308.873925943689,-3.97163317015235));
#11738=CARTESIAN_POINT('Ctrl Pts',(-5.88038492654913,309.011425943689,-5.83242799455291));
#11739=CARTESIAN_POINT('Ctrl Pts',(-4.02836682984766,309.148925943689,-6.91182563342691));
#11740=CARTESIAN_POINT('Ctrl Pts',(-2.17634873314618,309.286425943689,-7.99122327230091));
#11741=CARTESIAN_POINT('Ctrl Pts',(-0.0327551936971984,309.423925943689,
-8.));
#11742=CARTESIAN_POINT('Ctrl Pts',(2.11083834575178,309.561425943689,-8.00877672769909));
#11743=CARTESIAN_POINT('Ctrl Pts',(3.97163317015235,309.698925943689,-6.94458082712411));
#11744=CARTESIAN_POINT('Ctrl Pts',(5.83242799455291,309.836425943689,-5.88038492654913));
#11745=CARTESIAN_POINT('Ctrl Pts',(6.91182563342691,309.973925943689,-4.02836682984766));
#11746=CARTESIAN_POINT('Ctrl Pts',(7.99122327230091,310.111425943689,-2.17634873314618));
#11747=CARTESIAN_POINT('Ctrl Pts',(8.,310.248925943689,-0.0327551936971989));
#11748=CARTESIAN_POINT('Ctrl Pts',(8.00877672769909,310.386425943689,2.11083834575178));
#11749=CARTESIAN_POINT('Ctrl Pts',(6.94458082712411,310.523925943689,3.97163317015235));
#11750=CARTESIAN_POINT('Ctrl Pts',(5.88038492654913,310.661425943689,5.83242799455291));
#11751=CARTESIAN_POINT('Ctrl Pts',(4.02836682984766,310.798925943689,6.91182563342691));
#11752=CARTESIAN_POINT('Ctrl Pts',(2.17634873314619,310.936425943689,7.99122327230091));
#11753=CARTESIAN_POINT('Ctrl Pts',(0.0327551936971994,311.073925943689,
8.));
#11754=CARTESIAN_POINT('Ctrl Pts',(-2.11083834575178,311.211425943689,8.00877672769909));
#11755=CARTESIAN_POINT('Ctrl Pts',(-3.97163317015234,311.348925943689,6.94458082712412));
#11756=CARTESIAN_POINT('Ctrl Pts',(-5.83242799455291,311.486425943689,5.88038492654913));
#11757=CARTESIAN_POINT('Ctrl Pts',(-6.91182563342691,311.623925943689,4.02836682984766));
#11758=CARTESIAN_POINT('Ctrl Pts',(-7.99122327230091,311.761425943689,2.17634873314619));
#11759=CARTESIAN_POINT('Ctrl Pts',(-8.,311.898925943689,0.0327551936971979));
#11760=CARTESIAN_POINT('Ctrl Pts',(-8.00877672769909,312.036425943689,-2.11083834575178));
#11761=CARTESIAN_POINT('Ctrl Pts',(-6.94458082712411,312.173925943689,-3.97163317015235));
#11762=CARTESIAN_POINT('Ctrl Pts',(-5.88038492654913,312.311425943689,-5.83242799455291));
#11763=CARTESIAN_POINT('Ctrl Pts',(-4.02836682984766,312.448925943689,-6.91182563342691));
#11764=CARTESIAN_POINT('Ctrl Pts',(-2.17634873314618,312.586425943689,-7.99122327230091));
#11765=CARTESIAN_POINT('Ctrl Pts',(-0.0327551936971984,312.723925943689,
-8.));
#11766=CARTESIAN_POINT('Ctrl Pts',(2.11083834575178,312.861425943689,-8.00877672769909));
#11767=CARTESIAN_POINT('Ctrl Pts',(3.97163317015235,312.998925943689,-6.94458082712411));
#11768=CARTESIAN_POINT('Ctrl Pts',(5.83242799455291,313.136425943689,-5.88038492654913));
#11769=CARTESIAN_POINT('Ctrl Pts',(6.91182563342691,313.273925943689,-4.02836682984766));
#11770=CARTESIAN_POINT('Ctrl Pts',(7.99122327230091,313.411425943689,-2.17634873314618));
#11771=CARTESIAN_POINT('Ctrl Pts',(8.,313.548925943689,-0.0327551936971989));
#11772=CARTESIAN_POINT('Ctrl Pts',(8.00877672769909,313.686425943689,2.11083834575178));
#11773=CARTESIAN_POINT('Ctrl Pts',(6.94458082712411,313.823925943689,3.97163317015235));
#11774=CARTESIAN_POINT('Ctrl Pts',(5.88038492654913,313.961425943689,5.83242799455291));
#11775=CARTESIAN_POINT('Ctrl Pts',(4.02836682984766,314.098925943689,6.91182563342691));
#11776=CARTESIAN_POINT('Ctrl Pts',(2.17634873314619,314.236425943689,7.99122327230091));
#11777=CARTESIAN_POINT('Ctrl Pts',(0.0327551936971994,314.373925943689,
8.));
#11778=CARTESIAN_POINT('Ctrl Pts',(-2.11083834575178,314.511425943689,8.00877672769909));
#11779=CARTESIAN_POINT('Ctrl Pts',(-3.97163317015234,314.648925943689,6.94458082712412));
#11780=CARTESIAN_POINT('Ctrl Pts',(-5.83242799455291,314.786425943689,5.88038492654913));
#11781=CARTESIAN_POINT('Ctrl Pts',(-6.91182563342691,314.923925943689,4.02836682984766));
#11782=CARTESIAN_POINT('Ctrl Pts',(-7.99122327230091,315.061425943689,2.17634873314619));
#11783=CARTESIAN_POINT('Ctrl Pts',(-8.,315.198925943689,0.0327551936971979));
#11784=CARTESIAN_POINT('Ctrl Pts',(-8.00877672769909,315.336425943689,-2.11083834575178));
#11785=CARTESIAN_POINT('Ctrl Pts',(-6.94458082712411,315.473925943689,-3.97163317015235));
#11786=CARTESIAN_POINT('Ctrl Pts',(-5.88038492654913,315.611425943689,-5.83242799455291));
#11787=CARTESIAN_POINT('Ctrl Pts',(-4.02836682984766,315.748925943689,-6.91182563342691));
#11788=CARTESIAN_POINT('Ctrl Pts',(-2.17634873314618,315.886425943689,-7.99122327230091));
#11789=CARTESIAN_POINT('Ctrl Pts',(-0.0327551936971984,316.023925943689,
-8.));
#11790=CARTESIAN_POINT('Ctrl Pts',(2.11083834575178,316.161425943689,-8.00877672769909));
#11791=CARTESIAN_POINT('Ctrl Pts',(3.97163317015235,316.298925943689,-6.94458082712411));
#11792=CARTESIAN_POINT('Ctrl Pts',(5.83242799455291,316.436425943689,-5.88038492654913));
#11793=CARTESIAN_POINT('Ctrl Pts',(6.91182563342691,316.573925943689,-4.02836682984766));
#11794=CARTESIAN_POINT('Ctrl Pts',(7.99122327230091,316.711425943689,-2.17634873314618));
#11795=CARTESIAN_POINT('Ctrl Pts',(8.,316.848925943689,-0.0327551936971989));
#11796=CARTESIAN_POINT('Ctrl Pts',(8.00877672769909,316.986425943689,2.11083834575178));
#11797=CARTESIAN_POINT('Ctrl Pts',(6.94458082712411,317.123925943689,3.97163317015235));
#11798=CARTESIAN_POINT('Ctrl Pts',(5.88038492654913,317.261425943689,5.83242799455291));
#11799=CARTESIAN_POINT('Ctrl Pts',(4.02836682984766,317.398925943689,6.91182563342691));
#11800=CARTESIAN_POINT('Ctrl Pts',(2.17634873314619,317.536425943689,7.99122327230091));
#11801=CARTESIAN_POINT('Ctrl Pts',(0.0327551936971994,317.673925943689,
8.));
#11802=CARTESIAN_POINT('Ctrl Pts',(-2.11083834575178,317.811425943689,8.00877672769909));
#11803=CARTESIAN_POINT('Ctrl Pts',(-3.97163317015234,317.948925943689,6.94458082712412));
#11804=CARTESIAN_POINT('Ctrl Pts',(-5.83242799455291,318.086425943689,5.88038492654913));
#11805=CARTESIAN_POINT('Ctrl Pts',(-6.91182563342691,318.223925943689,4.02836682984766));
#11806=CARTESIAN_POINT('Ctrl Pts',(-7.99122327230091,318.361425943689,2.17634873314619));
#11807=CARTESIAN_POINT('Ctrl Pts',(-8.,318.498925943689,0.0327551936971979));
#11808=CARTESIAN_POINT('Ctrl Pts',(-7.,285.498925943689,0.0327551936971879));
#11809=CARTESIAN_POINT('Ctrl Pts',(-7.00877672769909,285.636425943689,-1.84288915332067));
#11810=CARTESIAN_POINT('Ctrl Pts',(-6.07855542333967,285.773925943689,-3.47163317015236));
#11811=CARTESIAN_POINT('Ctrl Pts',(-5.14833411898024,285.911425943689,-5.10037718698404));
#11812=CARTESIAN_POINT('Ctrl Pts',(-3.52836682984765,286.048925943689,-6.04580022964248));
#11813=CARTESIAN_POINT('Ctrl Pts',(-1.90839954071505,286.186425943689,-6.99122327230092));
#11814=CARTESIAN_POINT('Ctrl Pts',(-0.0327551936971884,286.323925943689,
-7.));
#11815=CARTESIAN_POINT('Ctrl Pts',(1.84288915332067,286.461425943689,-7.00877672769909));
#11816=CARTESIAN_POINT('Ctrl Pts',(3.47163317015236,286.598925943689,-6.07855542333967));
#11817=CARTESIAN_POINT('Ctrl Pts',(5.10037718698404,286.736425943689,-5.14833411898024));
#11818=CARTESIAN_POINT('Ctrl Pts',(6.04580022964248,286.873925943689,-3.52836682984765));
#11819=CARTESIAN_POINT('Ctrl Pts',(6.99122327230092,287.011425943689,-1.90839954071505));
#11820=CARTESIAN_POINT('Ctrl Pts',(7.,287.148925943689,-0.0327551936971888));
#11821=CARTESIAN_POINT('Ctrl Pts',(7.00877672769909,287.286425943689,1.84288915332067));
#11822=CARTESIAN_POINT('Ctrl Pts',(6.07855542333967,287.423925943689,3.47163317015236));
#11823=CARTESIAN_POINT('Ctrl Pts',(5.14833411898025,287.561425943689,5.10037718698404));
#11824=CARTESIAN_POINT('Ctrl Pts',(3.52836682984765,287.698925943689,6.04580022964248));
#11825=CARTESIAN_POINT('Ctrl Pts',(1.90839954071505,287.836425943689,6.99122327230091));
#11826=CARTESIAN_POINT('Ctrl Pts',(0.0327551936971892,287.973925943689,
7.));
#11827=CARTESIAN_POINT('Ctrl Pts',(-1.84288915332067,288.111425943689,7.00877672769909));
#11828=CARTESIAN_POINT('Ctrl Pts',(-3.47163317015235,288.248925943689,6.07855542333967));
#11829=CARTESIAN_POINT('Ctrl Pts',(-5.10037718698404,288.386425943689,5.14833411898025));
#11830=CARTESIAN_POINT('Ctrl Pts',(-6.04580022964248,288.523925943689,3.52836682984765));
#11831=CARTESIAN_POINT('Ctrl Pts',(-6.99122327230091,288.661425943689,1.90839954071505));
#11832=CARTESIAN_POINT('Ctrl Pts',(-7.,288.798925943689,0.0327551936971879));
#11833=CARTESIAN_POINT('Ctrl Pts',(-7.00877672769909,288.936425943689,-1.84288915332067));
#11834=CARTESIAN_POINT('Ctrl Pts',(-6.07855542333967,289.073925943689,-3.47163317015236));
#11835=CARTESIAN_POINT('Ctrl Pts',(-5.14833411898024,289.211425943689,-5.10037718698404));
#11836=CARTESIAN_POINT('Ctrl Pts',(-3.52836682984765,289.348925943689,-6.04580022964248));
#11837=CARTESIAN_POINT('Ctrl Pts',(-1.90839954071505,289.486425943689,-6.99122327230092));
#11838=CARTESIAN_POINT('Ctrl Pts',(-0.0327551936971884,289.623925943689,
-7.));
#11839=CARTESIAN_POINT('Ctrl Pts',(1.84288915332067,289.761425943689,-7.00877672769909));
#11840=CARTESIAN_POINT('Ctrl Pts',(3.47163317015236,289.898925943689,-6.07855542333967));
#11841=CARTESIAN_POINT('Ctrl Pts',(5.10037718698404,290.036425943689,-5.14833411898024));
#11842=CARTESIAN_POINT('Ctrl Pts',(6.04580022964248,290.173925943689,-3.52836682984765));
#11843=CARTESIAN_POINT('Ctrl Pts',(6.99122327230092,290.311425943689,-1.90839954071505));
#11844=CARTESIAN_POINT('Ctrl Pts',(7.,290.448925943689,-0.0327551936971888));
#11845=CARTESIAN_POINT('Ctrl Pts',(7.00877672769909,290.586425943689,1.84288915332067));
#11846=CARTESIAN_POINT('Ctrl Pts',(6.07855542333967,290.723925943689,3.47163317015236));
#11847=CARTESIAN_POINT('Ctrl Pts',(5.14833411898025,290.861425943689,5.10037718698404));
#11848=CARTESIAN_POINT('Ctrl Pts',(3.52836682984765,290.998925943689,6.04580022964248));
#11849=CARTESIAN_POINT('Ctrl Pts',(1.90839954071505,291.136425943689,6.99122327230091));
#11850=CARTESIAN_POINT('Ctrl Pts',(0.0327551936971892,291.273925943689,
7.));
#11851=CARTESIAN_POINT('Ctrl Pts',(-1.84288915332067,291.411425943689,7.00877672769909));
#11852=CARTESIAN_POINT('Ctrl Pts',(-3.47163317015235,291.548925943689,6.07855542333967));
#11853=CARTESIAN_POINT('Ctrl Pts',(-5.10037718698404,291.686425943689,5.14833411898025));
#11854=CARTESIAN_POINT('Ctrl Pts',(-6.04580022964248,291.823925943689,3.52836682984765));
#11855=CARTESIAN_POINT('Ctrl Pts',(-6.99122327230091,291.961425943689,1.90839954071505));
#11856=CARTESIAN_POINT('Ctrl Pts',(-7.,292.098925943689,0.0327551936971879));
#11857=CARTESIAN_POINT('Ctrl Pts',(-7.00877672769909,292.236425943689,-1.84288915332067));
#11858=CARTESIAN_POINT('Ctrl Pts',(-6.07855542333967,292.373925943689,-3.47163317015236));
#11859=CARTESIAN_POINT('Ctrl Pts',(-5.14833411898024,292.511425943689,-5.10037718698404));
#11860=CARTESIAN_POINT('Ctrl Pts',(-3.52836682984765,292.648925943689,-6.04580022964248));
#11861=CARTESIAN_POINT('Ctrl Pts',(-1.90839954071505,292.786425943689,-6.99122327230092));
#11862=CARTESIAN_POINT('Ctrl Pts',(-0.0327551936971884,292.923925943689,
-7.));
#11863=CARTESIAN_POINT('Ctrl Pts',(1.84288915332067,293.061425943689,-7.00877672769909));
#11864=CARTESIAN_POINT('Ctrl Pts',(3.47163317015236,293.198925943689,-6.07855542333967));
#11865=CARTESIAN_POINT('Ctrl Pts',(5.10037718698404,293.336425943689,-5.14833411898024));
#11866=CARTESIAN_POINT('Ctrl Pts',(6.04580022964248,293.473925943689,-3.52836682984765));
#11867=CARTESIAN_POINT('Ctrl Pts',(6.99122327230092,293.611425943689,-1.90839954071505));
#11868=CARTESIAN_POINT('Ctrl Pts',(7.,293.748925943689,-0.0327551936971888));
#11869=CARTESIAN_POINT('Ctrl Pts',(7.00877672769909,293.886425943689,1.84288915332067));
#11870=CARTESIAN_POINT('Ctrl Pts',(6.07855542333967,294.023925943689,3.47163317015236));
#11871=CARTESIAN_POINT('Ctrl Pts',(5.14833411898025,294.161425943689,5.10037718698404));
#11872=CARTESIAN_POINT('Ctrl Pts',(3.52836682984765,294.298925943689,6.04580022964248));
#11873=CARTESIAN_POINT('Ctrl Pts',(1.90839954071505,294.436425943689,6.99122327230091));
#11874=CARTESIAN_POINT('Ctrl Pts',(0.0327551936971892,294.573925943689,
7.));
#11875=CARTESIAN_POINT('Ctrl Pts',(-1.84288915332067,294.711425943689,7.00877672769909));
#11876=CARTESIAN_POINT('Ctrl Pts',(-3.47163317015235,294.848925943689,6.07855542333967));
#11877=CARTESIAN_POINT('Ctrl Pts',(-5.10037718698404,294.986425943689,5.14833411898025));
#11878=CARTESIAN_POINT('Ctrl Pts',(-6.04580022964248,295.123925943689,3.52836682984765));
#11879=CARTESIAN_POINT('Ctrl Pts',(-6.99122327230091,295.261425943689,1.90839954071505));
#11880=CARTESIAN_POINT('Ctrl Pts',(-7.,295.398925943689,0.0327551936971879));
#11881=CARTESIAN_POINT('Ctrl Pts',(-7.00877672769909,295.536425943689,-1.84288915332067));
#11882=CARTESIAN_POINT('Ctrl Pts',(-6.07855542333967,295.673925943689,-3.47163317015236));
#11883=CARTESIAN_POINT('Ctrl Pts',(-5.14833411898024,295.811425943689,-5.10037718698404));
#11884=CARTESIAN_POINT('Ctrl Pts',(-3.52836682984765,295.948925943689,-6.04580022964248));
#11885=CARTESIAN_POINT('Ctrl Pts',(-1.90839954071505,296.086425943689,-6.99122327230092));
#11886=CARTESIAN_POINT('Ctrl Pts',(-0.0327551936971884,296.223925943689,
-7.));
#11887=CARTESIAN_POINT('Ctrl Pts',(1.84288915332067,296.361425943689,-7.00877672769909));
#11888=CARTESIAN_POINT('Ctrl Pts',(3.47163317015236,296.498925943689,-6.07855542333967));
#11889=CARTESIAN_POINT('Ctrl Pts',(5.10037718698404,296.636425943689,-5.14833411898024));
#11890=CARTESIAN_POINT('Ctrl Pts',(6.04580022964248,296.773925943689,-3.52836682984765));
#11891=CARTESIAN_POINT('Ctrl Pts',(6.99122327230092,296.911425943689,-1.90839954071505));
#11892=CARTESIAN_POINT('Ctrl Pts',(7.,297.048925943689,-0.0327551936971888));
#11893=CARTESIAN_POINT('Ctrl Pts',(7.00877672769909,297.186425943689,1.84288915332067));
#11894=CARTESIAN_POINT('Ctrl Pts',(6.07855542333967,297.323925943689,3.47163317015236));
#11895=CARTESIAN_POINT('Ctrl Pts',(5.14833411898025,297.461425943689,5.10037718698404));
#11896=CARTESIAN_POINT('Ctrl Pts',(3.52836682984765,297.598925943689,6.04580022964248));
#11897=CARTESIAN_POINT('Ctrl Pts',(1.90839954071505,297.736425943689,6.99122327230091));
#11898=CARTESIAN_POINT('Ctrl Pts',(0.0327551936971892,297.873925943689,
7.));
#11899=CARTESIAN_POINT('Ctrl Pts',(-1.84288915332067,298.011425943689,7.00877672769909));
#11900=CARTESIAN_POINT('Ctrl Pts',(-3.47163317015235,298.148925943689,6.07855542333967));
#11901=CARTESIAN_POINT('Ctrl Pts',(-5.10037718698404,298.286425943689,5.14833411898025));
#11902=CARTESIAN_POINT('Ctrl Pts',(-6.04580022964248,298.423925943689,3.52836682984765));
#11903=CARTESIAN_POINT('Ctrl Pts',(-6.99122327230091,298.561425943689,1.90839954071505));
#11904=CARTESIAN_POINT('Ctrl Pts',(-7.,298.698925943689,0.0327551936971879));
#11905=CARTESIAN_POINT('Ctrl Pts',(-7.00877672769909,298.836425943689,-1.84288915332067));
#11906=CARTESIAN_POINT('Ctrl Pts',(-6.07855542333967,298.973925943689,-3.47163317015236));
#11907=CARTESIAN_POINT('Ctrl Pts',(-5.14833411898024,299.111425943689,-5.10037718698404));
#11908=CARTESIAN_POINT('Ctrl Pts',(-3.52836682984765,299.248925943689,-6.04580022964248));
#11909=CARTESIAN_POINT('Ctrl Pts',(-1.90839954071505,299.386425943689,-6.99122327230092));
#11910=CARTESIAN_POINT('Ctrl Pts',(-0.0327551936971884,299.523925943689,
-7.));
#11911=CARTESIAN_POINT('Ctrl Pts',(1.84288915332067,299.661425943689,-7.00877672769909));
#11912=CARTESIAN_POINT('Ctrl Pts',(3.47163317015236,299.798925943689,-6.07855542333967));
#11913=CARTESIAN_POINT('Ctrl Pts',(5.10037718698404,299.936425943689,-5.14833411898024));
#11914=CARTESIAN_POINT('Ctrl Pts',(6.04580022964248,300.073925943689,-3.52836682984765));
#11915=CARTESIAN_POINT('Ctrl Pts',(6.99122327230092,300.211425943689,-1.90839954071505));
#11916=CARTESIAN_POINT('Ctrl Pts',(7.,300.348925943689,-0.0327551936971888));
#11917=CARTESIAN_POINT('Ctrl Pts',(7.00877672769909,300.486425943689,1.84288915332067));
#11918=CARTESIAN_POINT('Ctrl Pts',(6.07855542333967,300.623925943689,3.47163317015236));
#11919=CARTESIAN_POINT('Ctrl Pts',(5.14833411898025,300.761425943689,5.10037718698404));
#11920=CARTESIAN_POINT('Ctrl Pts',(3.52836682984765,300.898925943689,6.04580022964248));
#11921=CARTESIAN_POINT('Ctrl Pts',(1.90839954071505,301.036425943689,6.99122327230091));
#11922=CARTESIAN_POINT('Ctrl Pts',(0.0327551936971892,301.173925943689,
7.));
#11923=CARTESIAN_POINT('Ctrl Pts',(-1.84288915332067,301.311425943689,7.00877672769909));
#11924=CARTESIAN_POINT('Ctrl Pts',(-3.47163317015235,301.448925943689,6.07855542333967));
#11925=CARTESIAN_POINT('Ctrl Pts',(-5.10037718698404,301.586425943689,5.14833411898025));
#11926=CARTESIAN_POINT('Ctrl Pts',(-6.04580022964248,301.723925943689,3.52836682984765));
#11927=CARTESIAN_POINT('Ctrl Pts',(-6.99122327230091,301.861425943689,1.90839954071505));
#11928=CARTESIAN_POINT('Ctrl Pts',(-7.,301.998925943689,0.0327551936971879));
#11929=CARTESIAN_POINT('Ctrl Pts',(-7.00877672769909,302.136425943689,-1.84288915332067));
#11930=CARTESIAN_POINT('Ctrl Pts',(-6.07855542333967,302.273925943689,-3.47163317015236));
#11931=CARTESIAN_POINT('Ctrl Pts',(-5.14833411898024,302.411425943689,-5.10037718698404));
#11932=CARTESIAN_POINT('Ctrl Pts',(-3.52836682984765,302.548925943689,-6.04580022964248));
#11933=CARTESIAN_POINT('Ctrl Pts',(-1.90839954071505,302.686425943689,-6.99122327230092));
#11934=CARTESIAN_POINT('Ctrl Pts',(-0.0327551936971884,302.823925943689,
-7.));
#11935=CARTESIAN_POINT('Ctrl Pts',(1.84288915332067,302.961425943689,-7.00877672769909));
#11936=CARTESIAN_POINT('Ctrl Pts',(3.47163317015236,303.098925943689,-6.07855542333967));
#11937=CARTESIAN_POINT('Ctrl Pts',(5.10037718698404,303.236425943689,-5.14833411898024));
#11938=CARTESIAN_POINT('Ctrl Pts',(6.04580022964248,303.373925943689,-3.52836682984765));
#11939=CARTESIAN_POINT('Ctrl Pts',(6.99122327230092,303.511425943689,-1.90839954071505));
#11940=CARTESIAN_POINT('Ctrl Pts',(7.,303.648925943689,-0.0327551936971888));
#11941=CARTESIAN_POINT('Ctrl Pts',(7.00877672769909,303.786425943689,1.84288915332067));
#11942=CARTESIAN_POINT('Ctrl Pts',(6.07855542333967,303.923925943689,3.47163317015236));
#11943=CARTESIAN_POINT('Ctrl Pts',(5.14833411898025,304.061425943689,5.10037718698404));
#11944=CARTESIAN_POINT('Ctrl Pts',(3.52836682984765,304.198925943689,6.04580022964248));
#11945=CARTESIAN_POINT('Ctrl Pts',(1.90839954071505,304.336425943689,6.99122327230091));
#11946=CARTESIAN_POINT('Ctrl Pts',(0.0327551936971892,304.473925943689,
7.));
#11947=CARTESIAN_POINT('Ctrl Pts',(-1.84288915332067,304.611425943689,7.00877672769909));
#11948=CARTESIAN_POINT('Ctrl Pts',(-3.47163317015235,304.748925943689,6.07855542333967));
#11949=CARTESIAN_POINT('Ctrl Pts',(-5.10037718698404,304.886425943689,5.14833411898025));
#11950=CARTESIAN_POINT('Ctrl Pts',(-6.04580022964248,305.023925943689,3.52836682984765));
#11951=CARTESIAN_POINT('Ctrl Pts',(-6.99122327230091,305.161425943689,1.90839954071505));
#11952=CARTESIAN_POINT('Ctrl Pts',(-7.,305.298925943689,0.0327551936971879));
#11953=CARTESIAN_POINT('Ctrl Pts',(-7.00877672769909,305.436425943689,-1.84288915332067));
#11954=CARTESIAN_POINT('Ctrl Pts',(-6.07855542333967,305.573925943689,-3.47163317015236));
#11955=CARTESIAN_POINT('Ctrl Pts',(-5.14833411898024,305.711425943689,-5.10037718698404));
#11956=CARTESIAN_POINT('Ctrl Pts',(-3.52836682984765,305.848925943689,-6.04580022964248));
#11957=CARTESIAN_POINT('Ctrl Pts',(-1.90839954071505,305.986425943689,-6.99122327230092));
#11958=CARTESIAN_POINT('Ctrl Pts',(-0.0327551936971884,306.123925943689,
-7.));
#11959=CARTESIAN_POINT('Ctrl Pts',(1.84288915332067,306.261425943689,-7.00877672769909));
#11960=CARTESIAN_POINT('Ctrl Pts',(3.47163317015236,306.398925943689,-6.07855542333967));
#11961=CARTESIAN_POINT('Ctrl Pts',(5.10037718698404,306.536425943689,-5.14833411898024));
#11962=CARTESIAN_POINT('Ctrl Pts',(6.04580022964248,306.673925943689,-3.52836682984765));
#11963=CARTESIAN_POINT('Ctrl Pts',(6.99122327230092,306.811425943689,-1.90839954071505));
#11964=CARTESIAN_POINT('Ctrl Pts',(7.,306.948925943689,-0.0327551936971888));
#11965=CARTESIAN_POINT('Ctrl Pts',(7.00877672769909,307.086425943689,1.84288915332067));
#11966=CARTESIAN_POINT('Ctrl Pts',(6.07855542333967,307.223925943689,3.47163317015236));
#11967=CARTESIAN_POINT('Ctrl Pts',(5.14833411898025,307.361425943689,5.10037718698404));
#11968=CARTESIAN_POINT('Ctrl Pts',(3.52836682984765,307.498925943689,6.04580022964248));
#11969=CARTESIAN_POINT('Ctrl Pts',(1.90839954071505,307.636425943689,6.99122327230091));
#11970=CARTESIAN_POINT('Ctrl Pts',(0.0327551936971892,307.773925943689,
7.));
#11971=CARTESIAN_POINT('Ctrl Pts',(-1.84288915332067,307.911425943689,7.00877672769909));
#11972=CARTESIAN_POINT('Ctrl Pts',(-3.47163317015235,308.048925943689,6.07855542333967));
#11973=CARTESIAN_POINT('Ctrl Pts',(-5.10037718698404,308.186425943689,5.14833411898025));
#11974=CARTESIAN_POINT('Ctrl Pts',(-6.04580022964248,308.323925943689,3.52836682984765));
#11975=CARTESIAN_POINT('Ctrl Pts',(-6.99122327230091,308.461425943689,1.90839954071505));
#11976=CARTESIAN_POINT('Ctrl Pts',(-7.,308.598925943689,0.0327551936971879));
#11977=CARTESIAN_POINT('Ctrl Pts',(-7.00877672769909,308.736425943689,-1.84288915332067));
#11978=CARTESIAN_POINT('Ctrl Pts',(-6.07855542333967,308.873925943689,-3.47163317015236));
#11979=CARTESIAN_POINT('Ctrl Pts',(-5.14833411898024,309.011425943689,-5.10037718698404));
#11980=CARTESIAN_POINT('Ctrl Pts',(-3.52836682984765,309.148925943689,-6.04580022964248));
#11981=CARTESIAN_POINT('Ctrl Pts',(-1.90839954071505,309.286425943689,-6.99122327230092));
#11982=CARTESIAN_POINT('Ctrl Pts',(-0.0327551936971884,309.423925943689,
-7.));
#11983=CARTESIAN_POINT('Ctrl Pts',(1.84288915332067,309.561425943689,-7.00877672769909));
#11984=CARTESIAN_POINT('Ctrl Pts',(3.47163317015236,309.698925943689,-6.07855542333967));
#11985=CARTESIAN_POINT('Ctrl Pts',(5.10037718698404,309.836425943689,-5.14833411898024));
#11986=CARTESIAN_POINT('Ctrl Pts',(6.04580022964248,309.973925943689,-3.52836682984765));
#11987=CARTESIAN_POINT('Ctrl Pts',(6.99122327230092,310.111425943689,-1.90839954071505));
#11988=CARTESIAN_POINT('Ctrl Pts',(7.,310.248925943689,-0.0327551936971888));
#11989=CARTESIAN_POINT('Ctrl Pts',(7.00877672769909,310.386425943689,1.84288915332067));
#11990=CARTESIAN_POINT('Ctrl Pts',(6.07855542333967,310.523925943689,3.47163317015236));
#11991=CARTESIAN_POINT('Ctrl Pts',(5.14833411898025,310.661425943689,5.10037718698404));
#11992=CARTESIAN_POINT('Ctrl Pts',(3.52836682984765,310.798925943689,6.04580022964248));
#11993=CARTESIAN_POINT('Ctrl Pts',(1.90839954071505,310.936425943689,6.99122327230091));
#11994=CARTESIAN_POINT('Ctrl Pts',(0.0327551936971892,311.073925943689,
7.));
#11995=CARTESIAN_POINT('Ctrl Pts',(-1.84288915332067,311.211425943689,7.00877672769909));
#11996=CARTESIAN_POINT('Ctrl Pts',(-3.47163317015235,311.348925943689,6.07855542333967));
#11997=CARTESIAN_POINT('Ctrl Pts',(-5.10037718698404,311.486425943689,5.14833411898025));
#11998=CARTESIAN_POINT('Ctrl Pts',(-6.04580022964248,311.623925943689,3.52836682984765));
#11999=CARTESIAN_POINT('Ctrl Pts',(-6.99122327230091,311.761425943689,1.90839954071505));
#12000=CARTESIAN_POINT('Ctrl Pts',(-7.,311.898925943689,0.0327551936971879));
#12001=CARTESIAN_POINT('Ctrl Pts',(-7.00877672769909,312.036425943689,-1.84288915332067));
#12002=CARTESIAN_POINT('Ctrl Pts',(-6.07855542333967,312.173925943689,-3.47163317015236));
#12003=CARTESIAN_POINT('Ctrl Pts',(-5.14833411898024,312.311425943689,-5.10037718698404));
#12004=CARTESIAN_POINT('Ctrl Pts',(-3.52836682984765,312.448925943689,-6.04580022964248));
#12005=CARTESIAN_POINT('Ctrl Pts',(-1.90839954071505,312.586425943689,-6.99122327230092));
#12006=CARTESIAN_POINT('Ctrl Pts',(-0.0327551936971884,312.723925943689,
-7.));
#12007=CARTESIAN_POINT('Ctrl Pts',(1.84288915332067,312.861425943689,-7.00877672769909));
#12008=CARTESIAN_POINT('Ctrl Pts',(3.47163317015236,312.998925943689,-6.07855542333967));
#12009=CARTESIAN_POINT('Ctrl Pts',(5.10037718698404,313.136425943689,-5.14833411898024));
#12010=CARTESIAN_POINT('Ctrl Pts',(6.04580022964248,313.273925943689,-3.52836682984765));
#12011=CARTESIAN_POINT('Ctrl Pts',(6.99122327230092,313.411425943689,-1.90839954071505));
#12012=CARTESIAN_POINT('Ctrl Pts',(7.,313.548925943689,-0.0327551936971888));
#12013=CARTESIAN_POINT('Ctrl Pts',(7.00877672769909,313.686425943689,1.84288915332067));
#12014=CARTESIAN_POINT('Ctrl Pts',(6.07855542333967,313.823925943689,3.47163317015236));
#12015=CARTESIAN_POINT('Ctrl Pts',(5.14833411898025,313.961425943689,5.10037718698404));
#12016=CARTESIAN_POINT('Ctrl Pts',(3.52836682984765,314.098925943689,6.04580022964248));
#12017=CARTESIAN_POINT('Ctrl Pts',(1.90839954071505,314.236425943689,6.99122327230091));
#12018=CARTESIAN_POINT('Ctrl Pts',(0.0327551936971892,314.373925943689,
7.));
#12019=CARTESIAN_POINT('Ctrl Pts',(-1.84288915332067,314.511425943689,7.00877672769909));
#12020=CARTESIAN_POINT('Ctrl Pts',(-3.47163317015235,314.648925943689,6.07855542333967));
#12021=CARTESIAN_POINT('Ctrl Pts',(-5.10037718698404,314.786425943689,5.14833411898025));
#12022=CARTESIAN_POINT('Ctrl Pts',(-6.04580022964248,314.923925943689,3.52836682984765));
#12023=CARTESIAN_POINT('Ctrl Pts',(-6.99122327230091,315.061425943689,1.90839954071505));
#12024=CARTESIAN_POINT('Ctrl Pts',(-7.,315.198925943689,0.0327551936971879));
#12025=CARTESIAN_POINT('Ctrl Pts',(-7.00877672769909,315.336425943689,-1.84288915332067));
#12026=CARTESIAN_POINT('Ctrl Pts',(-6.07855542333967,315.473925943689,-3.47163317015236));
#12027=CARTESIAN_POINT('Ctrl Pts',(-5.14833411898024,315.611425943689,-5.10037718698404));
#12028=CARTESIAN_POINT('Ctrl Pts',(-3.52836682984765,315.748925943689,-6.04580022964248));
#12029=CARTESIAN_POINT('Ctrl Pts',(-1.90839954071505,315.886425943689,-6.99122327230092));
#12030=CARTESIAN_POINT('Ctrl Pts',(-0.0327551936971884,316.023925943689,
-7.));
#12031=CARTESIAN_POINT('Ctrl Pts',(1.84288915332067,316.161425943689,-7.00877672769909));
#12032=CARTESIAN_POINT('Ctrl Pts',(3.47163317015236,316.298925943689,-6.07855542333967));
#12033=CARTESIAN_POINT('Ctrl Pts',(5.10037718698404,316.436425943689,-5.14833411898024));
#12034=CARTESIAN_POINT('Ctrl Pts',(6.04580022964248,316.573925943689,-3.52836682984765));
#12035=CARTESIAN_POINT('Ctrl Pts',(6.99122327230092,316.711425943689,-1.90839954071505));
#12036=CARTESIAN_POINT('Ctrl Pts',(7.,316.848925943689,-0.0327551936971888));
#12037=CARTESIAN_POINT('Ctrl Pts',(7.00877672769909,316.986425943689,1.84288915332067));
#12038=CARTESIAN_POINT('Ctrl Pts',(6.07855542333967,317.123925943689,3.47163317015236));
#12039=CARTESIAN_POINT('Ctrl Pts',(5.14833411898025,317.261425943689,5.10037718698404));
#12040=CARTESIAN_POINT('Ctrl Pts',(3.52836682984765,317.398925943689,6.04580022964248));
#12041=CARTESIAN_POINT('Ctrl Pts',(1.90839954071505,317.536425943689,6.99122327230091));
#12042=CARTESIAN_POINT('Ctrl Pts',(0.0327551936971892,317.673925943689,
7.));
#12043=CARTESIAN_POINT('Ctrl Pts',(-1.84288915332067,317.811425943689,7.00877672769909));
#12044=CARTESIAN_POINT('Ctrl Pts',(-3.47163317015235,317.948925943689,6.07855542333967));
#12045=CARTESIAN_POINT('Ctrl Pts',(-5.10037718698404,318.086425943689,5.14833411898025));
#12046=CARTESIAN_POINT('Ctrl Pts',(-6.04580022964248,318.223925943689,3.52836682984765));
#12047=CARTESIAN_POINT('Ctrl Pts',(-6.99122327230091,318.361425943689,1.90839954071505));
#12048=CARTESIAN_POINT('Ctrl Pts',(-7.,318.498925943689,0.0327551936971879));
#12049=CARTESIAN_POINT('Ctrl Pts',(-7.,284.501074056311,-0.0327551936970413));
#12050=CARTESIAN_POINT('Ctrl Pts',(-6.99122327230096,284.638574056311,-1.9083995407149));
#12051=CARTESIAN_POINT('Ctrl Pts',(-6.04580022964255,284.776074056311,-3.52836682984752));
#12052=CARTESIAN_POINT('Ctrl Pts',(-5.10037718698415,284.913574056311,-5.14833411898014));
#12053=CARTESIAN_POINT('Ctrl Pts',(-3.47163317015249,285.051074056311,-6.07855542333959));
#12054=CARTESIAN_POINT('Ctrl Pts',(-1.84288915332082,285.188574056311,-7.00877672769905));
#12055=CARTESIAN_POINT('Ctrl Pts',(0.0327551936970409,285.326074056311,
-7.));
#12056=CARTESIAN_POINT('Ctrl Pts',(1.9083995407149,285.463574056311,-6.99122327230096));
#12057=CARTESIAN_POINT('Ctrl Pts',(3.52836682984752,285.601074056311,-6.04580022964255));
#12058=CARTESIAN_POINT('Ctrl Pts',(5.14833411898014,285.738574056311,-5.10037718698415));
#12059=CARTESIAN_POINT('Ctrl Pts',(6.07855542333959,285.876074056311,-3.47163317015249));
#12060=CARTESIAN_POINT('Ctrl Pts',(7.00877672769905,286.013574056311,-1.84288915332082));
#12061=CARTESIAN_POINT('Ctrl Pts',(7.,286.151074056311,0.0327551936970405));
#12062=CARTESIAN_POINT('Ctrl Pts',(6.99122327230096,286.288574056311,1.9083995407149));
#12063=CARTESIAN_POINT('Ctrl Pts',(6.04580022964255,286.426074056311,3.52836682984752));
#12064=CARTESIAN_POINT('Ctrl Pts',(5.10037718698415,286.563574056311,5.14833411898013));
#12065=CARTESIAN_POINT('Ctrl Pts',(3.47163317015249,286.701074056311,6.07855542333959));
#12066=CARTESIAN_POINT('Ctrl Pts',(1.84288915332082,286.838574056311,7.00877672769905));
#12067=CARTESIAN_POINT('Ctrl Pts',(-0.03275519369704,286.976074056311,7.));
#12068=CARTESIAN_POINT('Ctrl Pts',(-1.9083995407149,287.113574056311,6.99122327230096));
#12069=CARTESIAN_POINT('Ctrl Pts',(-3.52836682984752,287.251074056311,6.04580022964255));
#12070=CARTESIAN_POINT('Ctrl Pts',(-5.14833411898014,287.388574056311,5.10037718698415));
#12071=CARTESIAN_POINT('Ctrl Pts',(-6.07855542333959,287.526074056311,3.47163317015249));
#12072=CARTESIAN_POINT('Ctrl Pts',(-7.00877672769905,287.663574056311,1.84288915332082));
#12073=CARTESIAN_POINT('Ctrl Pts',(-7.,287.801074056311,-0.0327551936970413));
#12074=CARTESIAN_POINT('Ctrl Pts',(-6.99122327230096,287.938574056311,-1.9083995407149));
#12075=CARTESIAN_POINT('Ctrl Pts',(-6.04580022964255,288.076074056311,-3.52836682984752));
#12076=CARTESIAN_POINT('Ctrl Pts',(-5.10037718698415,288.213574056311,-5.14833411898014));
#12077=CARTESIAN_POINT('Ctrl Pts',(-3.47163317015249,288.351074056311,-6.07855542333959));
#12078=CARTESIAN_POINT('Ctrl Pts',(-1.84288915332082,288.488574056311,-7.00877672769905));
#12079=CARTESIAN_POINT('Ctrl Pts',(0.0327551936970409,288.626074056311,
-7.));
#12080=CARTESIAN_POINT('Ctrl Pts',(1.9083995407149,288.763574056311,-6.99122327230096));
#12081=CARTESIAN_POINT('Ctrl Pts',(3.52836682984752,288.901074056311,-6.04580022964255));
#12082=CARTESIAN_POINT('Ctrl Pts',(5.14833411898014,289.038574056311,-5.10037718698415));
#12083=CARTESIAN_POINT('Ctrl Pts',(6.07855542333959,289.176074056311,-3.47163317015249));
#12084=CARTESIAN_POINT('Ctrl Pts',(7.00877672769905,289.313574056311,-1.84288915332082));
#12085=CARTESIAN_POINT('Ctrl Pts',(7.,289.451074056311,0.0327551936970405));
#12086=CARTESIAN_POINT('Ctrl Pts',(6.99122327230096,289.588574056311,1.9083995407149));
#12087=CARTESIAN_POINT('Ctrl Pts',(6.04580022964255,289.726074056311,3.52836682984752));
#12088=CARTESIAN_POINT('Ctrl Pts',(5.10037718698415,289.863574056311,5.14833411898013));
#12089=CARTESIAN_POINT('Ctrl Pts',(3.47163317015249,290.001074056311,6.07855542333959));
#12090=CARTESIAN_POINT('Ctrl Pts',(1.84288915332082,290.138574056311,7.00877672769905));
#12091=CARTESIAN_POINT('Ctrl Pts',(-0.03275519369704,290.276074056311,7.));
#12092=CARTESIAN_POINT('Ctrl Pts',(-1.9083995407149,290.413574056311,6.99122327230096));
#12093=CARTESIAN_POINT('Ctrl Pts',(-3.52836682984752,290.551074056311,6.04580022964255));
#12094=CARTESIAN_POINT('Ctrl Pts',(-5.14833411898014,290.688574056311,5.10037718698415));
#12095=CARTESIAN_POINT('Ctrl Pts',(-6.07855542333959,290.826074056311,3.47163317015249));
#12096=CARTESIAN_POINT('Ctrl Pts',(-7.00877672769905,290.963574056311,1.84288915332082));
#12097=CARTESIAN_POINT('Ctrl Pts',(-7.,291.101074056311,-0.0327551936970413));
#12098=CARTESIAN_POINT('Ctrl Pts',(-6.99122327230096,291.238574056311,-1.9083995407149));
#12099=CARTESIAN_POINT('Ctrl Pts',(-6.04580022964255,291.376074056311,-3.52836682984752));
#12100=CARTESIAN_POINT('Ctrl Pts',(-5.10037718698415,291.513574056311,-5.14833411898014));
#12101=CARTESIAN_POINT('Ctrl Pts',(-3.47163317015249,291.651074056311,-6.07855542333959));
#12102=CARTESIAN_POINT('Ctrl Pts',(-1.84288915332082,291.788574056311,-7.00877672769905));
#12103=CARTESIAN_POINT('Ctrl Pts',(0.0327551936970409,291.926074056311,
-7.));
#12104=CARTESIAN_POINT('Ctrl Pts',(1.9083995407149,292.063574056311,-6.99122327230096));
#12105=CARTESIAN_POINT('Ctrl Pts',(3.52836682984752,292.201074056311,-6.04580022964255));
#12106=CARTESIAN_POINT('Ctrl Pts',(5.14833411898014,292.338574056311,-5.10037718698415));
#12107=CARTESIAN_POINT('Ctrl Pts',(6.07855542333959,292.476074056311,-3.47163317015249));
#12108=CARTESIAN_POINT('Ctrl Pts',(7.00877672769905,292.613574056311,-1.84288915332082));
#12109=CARTESIAN_POINT('Ctrl Pts',(7.,292.751074056311,0.0327551936970405));
#12110=CARTESIAN_POINT('Ctrl Pts',(6.99122327230096,292.888574056311,1.9083995407149));
#12111=CARTESIAN_POINT('Ctrl Pts',(6.04580022964255,293.026074056311,3.52836682984752));
#12112=CARTESIAN_POINT('Ctrl Pts',(5.10037718698415,293.163574056311,5.14833411898013));
#12113=CARTESIAN_POINT('Ctrl Pts',(3.47163317015249,293.301074056311,6.07855542333959));
#12114=CARTESIAN_POINT('Ctrl Pts',(1.84288915332082,293.438574056311,7.00877672769905));
#12115=CARTESIAN_POINT('Ctrl Pts',(-0.03275519369704,293.576074056311,7.));
#12116=CARTESIAN_POINT('Ctrl Pts',(-1.9083995407149,293.713574056311,6.99122327230096));
#12117=CARTESIAN_POINT('Ctrl Pts',(-3.52836682984752,293.851074056311,6.04580022964255));
#12118=CARTESIAN_POINT('Ctrl Pts',(-5.14833411898014,293.988574056311,5.10037718698415));
#12119=CARTESIAN_POINT('Ctrl Pts',(-6.07855542333959,294.126074056311,3.47163317015249));
#12120=CARTESIAN_POINT('Ctrl Pts',(-7.00877672769905,294.263574056311,1.84288915332082));
#12121=CARTESIAN_POINT('Ctrl Pts',(-7.,294.401074056311,-0.0327551936970413));
#12122=CARTESIAN_POINT('Ctrl Pts',(-6.99122327230096,294.538574056311,-1.9083995407149));
#12123=CARTESIAN_POINT('Ctrl Pts',(-6.04580022964255,294.676074056311,-3.52836682984752));
#12124=CARTESIAN_POINT('Ctrl Pts',(-5.10037718698415,294.813574056311,-5.14833411898014));
#12125=CARTESIAN_POINT('Ctrl Pts',(-3.47163317015249,294.951074056311,-6.07855542333959));
#12126=CARTESIAN_POINT('Ctrl Pts',(-1.84288915332082,295.088574056311,-7.00877672769905));
#12127=CARTESIAN_POINT('Ctrl Pts',(0.0327551936970409,295.226074056311,
-7.));
#12128=CARTESIAN_POINT('Ctrl Pts',(1.9083995407149,295.363574056311,-6.99122327230096));
#12129=CARTESIAN_POINT('Ctrl Pts',(3.52836682984752,295.501074056311,-6.04580022964255));
#12130=CARTESIAN_POINT('Ctrl Pts',(5.14833411898014,295.638574056311,-5.10037718698415));
#12131=CARTESIAN_POINT('Ctrl Pts',(6.07855542333959,295.776074056311,-3.47163317015249));
#12132=CARTESIAN_POINT('Ctrl Pts',(7.00877672769905,295.913574056311,-1.84288915332082));
#12133=CARTESIAN_POINT('Ctrl Pts',(7.,296.051074056311,0.0327551936970405));
#12134=CARTESIAN_POINT('Ctrl Pts',(6.99122327230096,296.188574056311,1.9083995407149));
#12135=CARTESIAN_POINT('Ctrl Pts',(6.04580022964255,296.326074056311,3.52836682984752));
#12136=CARTESIAN_POINT('Ctrl Pts',(5.10037718698415,296.463574056311,5.14833411898013));
#12137=CARTESIAN_POINT('Ctrl Pts',(3.47163317015249,296.601074056311,6.07855542333959));
#12138=CARTESIAN_POINT('Ctrl Pts',(1.84288915332082,296.738574056311,7.00877672769905));
#12139=CARTESIAN_POINT('Ctrl Pts',(-0.03275519369704,296.876074056311,7.));
#12140=CARTESIAN_POINT('Ctrl Pts',(-1.9083995407149,297.013574056311,6.99122327230096));
#12141=CARTESIAN_POINT('Ctrl Pts',(-3.52836682984752,297.151074056311,6.04580022964255));
#12142=CARTESIAN_POINT('Ctrl Pts',(-5.14833411898014,297.288574056311,5.10037718698415));
#12143=CARTESIAN_POINT('Ctrl Pts',(-6.07855542333959,297.426074056311,3.47163317015249));
#12144=CARTESIAN_POINT('Ctrl Pts',(-7.00877672769905,297.563574056311,1.84288915332082));
#12145=CARTESIAN_POINT('Ctrl Pts',(-7.,297.701074056311,-0.0327551936970413));
#12146=CARTESIAN_POINT('Ctrl Pts',(-6.99122327230096,297.838574056311,-1.9083995407149));
#12147=CARTESIAN_POINT('Ctrl Pts',(-6.04580022964255,297.976074056311,-3.52836682984752));
#12148=CARTESIAN_POINT('Ctrl Pts',(-5.10037718698415,298.113574056311,-5.14833411898014));
#12149=CARTESIAN_POINT('Ctrl Pts',(-3.47163317015249,298.251074056311,-6.07855542333959));
#12150=CARTESIAN_POINT('Ctrl Pts',(-1.84288915332082,298.388574056311,-7.00877672769905));
#12151=CARTESIAN_POINT('Ctrl Pts',(0.0327551936970409,298.526074056311,
-7.));
#12152=CARTESIAN_POINT('Ctrl Pts',(1.9083995407149,298.663574056311,-6.99122327230096));
#12153=CARTESIAN_POINT('Ctrl Pts',(3.52836682984752,298.801074056311,-6.04580022964255));
#12154=CARTESIAN_POINT('Ctrl Pts',(5.14833411898014,298.938574056311,-5.10037718698415));
#12155=CARTESIAN_POINT('Ctrl Pts',(6.07855542333959,299.076074056311,-3.47163317015249));
#12156=CARTESIAN_POINT('Ctrl Pts',(7.00877672769905,299.213574056311,-1.84288915332082));
#12157=CARTESIAN_POINT('Ctrl Pts',(7.,299.351074056311,0.0327551936970405));
#12158=CARTESIAN_POINT('Ctrl Pts',(6.99122327230096,299.488574056311,1.9083995407149));
#12159=CARTESIAN_POINT('Ctrl Pts',(6.04580022964255,299.626074056311,3.52836682984752));
#12160=CARTESIAN_POINT('Ctrl Pts',(5.10037718698415,299.763574056311,5.14833411898013));
#12161=CARTESIAN_POINT('Ctrl Pts',(3.47163317015249,299.901074056311,6.07855542333959));
#12162=CARTESIAN_POINT('Ctrl Pts',(1.84288915332082,300.038574056311,7.00877672769905));
#12163=CARTESIAN_POINT('Ctrl Pts',(-0.03275519369704,300.176074056311,7.));
#12164=CARTESIAN_POINT('Ctrl Pts',(-1.9083995407149,300.313574056311,6.99122327230096));
#12165=CARTESIAN_POINT('Ctrl Pts',(-3.52836682984752,300.451074056311,6.04580022964255));
#12166=CARTESIAN_POINT('Ctrl Pts',(-5.14833411898014,300.588574056311,5.10037718698415));
#12167=CARTESIAN_POINT('Ctrl Pts',(-6.07855542333959,300.726074056311,3.47163317015249));
#12168=CARTESIAN_POINT('Ctrl Pts',(-7.00877672769905,300.863574056311,1.84288915332082));
#12169=CARTESIAN_POINT('Ctrl Pts',(-7.,301.001074056311,-0.0327551936970413));
#12170=CARTESIAN_POINT('Ctrl Pts',(-6.99122327230096,301.138574056311,-1.9083995407149));
#12171=CARTESIAN_POINT('Ctrl Pts',(-6.04580022964255,301.276074056311,-3.52836682984752));
#12172=CARTESIAN_POINT('Ctrl Pts',(-5.10037718698415,301.413574056311,-5.14833411898014));
#12173=CARTESIAN_POINT('Ctrl Pts',(-3.47163317015249,301.551074056311,-6.07855542333959));
#12174=CARTESIAN_POINT('Ctrl Pts',(-1.84288915332082,301.688574056311,-7.00877672769905));
#12175=CARTESIAN_POINT('Ctrl Pts',(0.0327551936970409,301.826074056311,
-7.));
#12176=CARTESIAN_POINT('Ctrl Pts',(1.9083995407149,301.963574056311,-6.99122327230096));
#12177=CARTESIAN_POINT('Ctrl Pts',(3.52836682984752,302.101074056311,-6.04580022964255));
#12178=CARTESIAN_POINT('Ctrl Pts',(5.14833411898014,302.238574056311,-5.10037718698415));
#12179=CARTESIAN_POINT('Ctrl Pts',(6.07855542333959,302.376074056311,-3.47163317015249));
#12180=CARTESIAN_POINT('Ctrl Pts',(7.00877672769905,302.513574056311,-1.84288915332082));
#12181=CARTESIAN_POINT('Ctrl Pts',(7.,302.651074056311,0.0327551936970405));
#12182=CARTESIAN_POINT('Ctrl Pts',(6.99122327230096,302.788574056311,1.9083995407149));
#12183=CARTESIAN_POINT('Ctrl Pts',(6.04580022964255,302.926074056311,3.52836682984752));
#12184=CARTESIAN_POINT('Ctrl Pts',(5.10037718698415,303.063574056311,5.14833411898013));
#12185=CARTESIAN_POINT('Ctrl Pts',(3.47163317015249,303.201074056311,6.07855542333959));
#12186=CARTESIAN_POINT('Ctrl Pts',(1.84288915332082,303.338574056311,7.00877672769905));
#12187=CARTESIAN_POINT('Ctrl Pts',(-0.03275519369704,303.476074056311,7.));
#12188=CARTESIAN_POINT('Ctrl Pts',(-1.9083995407149,303.613574056311,6.99122327230096));
#12189=CARTESIAN_POINT('Ctrl Pts',(-3.52836682984752,303.751074056311,6.04580022964255));
#12190=CARTESIAN_POINT('Ctrl Pts',(-5.14833411898014,303.888574056311,5.10037718698415));
#12191=CARTESIAN_POINT('Ctrl Pts',(-6.07855542333959,304.026074056311,3.47163317015249));
#12192=CARTESIAN_POINT('Ctrl Pts',(-7.00877672769905,304.163574056311,1.84288915332082));
#12193=CARTESIAN_POINT('Ctrl Pts',(-7.,304.301074056311,-0.0327551936970413));
#12194=CARTESIAN_POINT('Ctrl Pts',(-6.99122327230096,304.438574056311,-1.9083995407149));
#12195=CARTESIAN_POINT('Ctrl Pts',(-6.04580022964255,304.576074056311,-3.52836682984752));
#12196=CARTESIAN_POINT('Ctrl Pts',(-5.10037718698415,304.713574056311,-5.14833411898014));
#12197=CARTESIAN_POINT('Ctrl Pts',(-3.47163317015249,304.851074056311,-6.07855542333959));
#12198=CARTESIAN_POINT('Ctrl Pts',(-1.84288915332082,304.988574056311,-7.00877672769905));
#12199=CARTESIAN_POINT('Ctrl Pts',(0.0327551936970409,305.126074056311,
-7.));
#12200=CARTESIAN_POINT('Ctrl Pts',(1.9083995407149,305.263574056311,-6.99122327230096));
#12201=CARTESIAN_POINT('Ctrl Pts',(3.52836682984752,305.401074056311,-6.04580022964255));
#12202=CARTESIAN_POINT('Ctrl Pts',(5.14833411898014,305.538574056311,-5.10037718698415));
#12203=CARTESIAN_POINT('Ctrl Pts',(6.07855542333959,305.676074056311,-3.47163317015249));
#12204=CARTESIAN_POINT('Ctrl Pts',(7.00877672769905,305.813574056311,-1.84288915332082));
#12205=CARTESIAN_POINT('Ctrl Pts',(7.,305.951074056311,0.0327551936970405));
#12206=CARTESIAN_POINT('Ctrl Pts',(6.99122327230096,306.088574056311,1.9083995407149));
#12207=CARTESIAN_POINT('Ctrl Pts',(6.04580022964255,306.226074056311,3.52836682984752));
#12208=CARTESIAN_POINT('Ctrl Pts',(5.10037718698415,306.363574056311,5.14833411898013));
#12209=CARTESIAN_POINT('Ctrl Pts',(3.47163317015249,306.501074056311,6.07855542333959));
#12210=CARTESIAN_POINT('Ctrl Pts',(1.84288915332082,306.638574056311,7.00877672769905));
#12211=CARTESIAN_POINT('Ctrl Pts',(-0.03275519369704,306.776074056311,7.));
#12212=CARTESIAN_POINT('Ctrl Pts',(-1.9083995407149,306.913574056311,6.99122327230096));
#12213=CARTESIAN_POINT('Ctrl Pts',(-3.52836682984752,307.051074056311,6.04580022964255));
#12214=CARTESIAN_POINT('Ctrl Pts',(-5.14833411898014,307.188574056311,5.10037718698415));
#12215=CARTESIAN_POINT('Ctrl Pts',(-6.07855542333959,307.326074056311,3.47163317015249));
#12216=CARTESIAN_POINT('Ctrl Pts',(-7.00877672769905,307.463574056311,1.84288915332082));
#12217=CARTESIAN_POINT('Ctrl Pts',(-7.,307.601074056311,-0.0327551936970413));
#12218=CARTESIAN_POINT('Ctrl Pts',(-6.99122327230096,307.738574056311,-1.9083995407149));
#12219=CARTESIAN_POINT('Ctrl Pts',(-6.04580022964255,307.876074056311,-3.52836682984752));
#12220=CARTESIAN_POINT('Ctrl Pts',(-5.10037718698415,308.013574056311,-5.14833411898014));
#12221=CARTESIAN_POINT('Ctrl Pts',(-3.47163317015249,308.151074056311,-6.07855542333959));
#12222=CARTESIAN_POINT('Ctrl Pts',(-1.84288915332082,308.288574056311,-7.00877672769905));
#12223=CARTESIAN_POINT('Ctrl Pts',(0.0327551936970409,308.426074056311,
-7.));
#12224=CARTESIAN_POINT('Ctrl Pts',(1.9083995407149,308.563574056311,-6.99122327230096));
#12225=CARTESIAN_POINT('Ctrl Pts',(3.52836682984752,308.701074056311,-6.04580022964255));
#12226=CARTESIAN_POINT('Ctrl Pts',(5.14833411898014,308.838574056311,-5.10037718698415));
#12227=CARTESIAN_POINT('Ctrl Pts',(6.07855542333959,308.976074056311,-3.47163317015249));
#12228=CARTESIAN_POINT('Ctrl Pts',(7.00877672769905,309.113574056311,-1.84288915332082));
#12229=CARTESIAN_POINT('Ctrl Pts',(7.,309.251074056311,0.0327551936970405));
#12230=CARTESIAN_POINT('Ctrl Pts',(6.99122327230096,309.388574056311,1.9083995407149));
#12231=CARTESIAN_POINT('Ctrl Pts',(6.04580022964255,309.526074056311,3.52836682984752));
#12232=CARTESIAN_POINT('Ctrl Pts',(5.10037718698415,309.663574056311,5.14833411898013));
#12233=CARTESIAN_POINT('Ctrl Pts',(3.47163317015249,309.801074056311,6.07855542333959));
#12234=CARTESIAN_POINT('Ctrl Pts',(1.84288915332082,309.938574056311,7.00877672769905));
#12235=CARTESIAN_POINT('Ctrl Pts',(-0.03275519369704,310.076074056311,7.));
#12236=CARTESIAN_POINT('Ctrl Pts',(-1.9083995407149,310.213574056311,6.99122327230096));
#12237=CARTESIAN_POINT('Ctrl Pts',(-3.52836682984752,310.351074056311,6.04580022964255));
#12238=CARTESIAN_POINT('Ctrl Pts',(-5.14833411898014,310.488574056311,5.10037718698415));
#12239=CARTESIAN_POINT('Ctrl Pts',(-6.07855542333959,310.626074056311,3.47163317015249));
#12240=CARTESIAN_POINT('Ctrl Pts',(-7.00877672769905,310.763574056311,1.84288915332082));
#12241=CARTESIAN_POINT('Ctrl Pts',(-7.,310.901074056311,-0.0327551936970413));
#12242=CARTESIAN_POINT('Ctrl Pts',(-6.99122327230096,311.038574056311,-1.9083995407149));
#12243=CARTESIAN_POINT('Ctrl Pts',(-6.04580022964255,311.176074056311,-3.52836682984752));
#12244=CARTESIAN_POINT('Ctrl Pts',(-5.10037718698415,311.313574056311,-5.14833411898014));
#12245=CARTESIAN_POINT('Ctrl Pts',(-3.47163317015249,311.451074056311,-6.07855542333959));
#12246=CARTESIAN_POINT('Ctrl Pts',(-1.84288915332082,311.588574056311,-7.00877672769905));
#12247=CARTESIAN_POINT('Ctrl Pts',(0.0327551936970409,311.726074056311,
-7.));
#12248=CARTESIAN_POINT('Ctrl Pts',(1.9083995407149,311.863574056311,-6.99122327230096));
#12249=CARTESIAN_POINT('Ctrl Pts',(3.52836682984752,312.001074056311,-6.04580022964255));
#12250=CARTESIAN_POINT('Ctrl Pts',(5.14833411898014,312.138574056311,-5.10037718698415));
#12251=CARTESIAN_POINT('Ctrl Pts',(6.07855542333959,312.276074056311,-3.47163317015249));
#12252=CARTESIAN_POINT('Ctrl Pts',(7.00877672769905,312.413574056311,-1.84288915332082));
#12253=CARTESIAN_POINT('Ctrl Pts',(7.,312.551074056311,0.0327551936970405));
#12254=CARTESIAN_POINT('Ctrl Pts',(6.99122327230096,312.688574056311,1.9083995407149));
#12255=CARTESIAN_POINT('Ctrl Pts',(6.04580022964255,312.826074056311,3.52836682984752));
#12256=CARTESIAN_POINT('Ctrl Pts',(5.10037718698415,312.963574056311,5.14833411898013));
#12257=CARTESIAN_POINT('Ctrl Pts',(3.47163317015249,313.101074056311,6.07855542333959));
#12258=CARTESIAN_POINT('Ctrl Pts',(1.84288915332082,313.238574056311,7.00877672769905));
#12259=CARTESIAN_POINT('Ctrl Pts',(-0.03275519369704,313.376074056311,7.));
#12260=CARTESIAN_POINT('Ctrl Pts',(-1.9083995407149,313.513574056311,6.99122327230096));
#12261=CARTESIAN_POINT('Ctrl Pts',(-3.52836682984752,313.651074056311,6.04580022964255));
#12262=CARTESIAN_POINT('Ctrl Pts',(-5.14833411898014,313.788574056311,5.10037718698415));
#12263=CARTESIAN_POINT('Ctrl Pts',(-6.07855542333959,313.926074056311,3.47163317015249));
#12264=CARTESIAN_POINT('Ctrl Pts',(-7.00877672769905,314.063574056311,1.84288915332082));
#12265=CARTESIAN_POINT('Ctrl Pts',(-7.,314.201074056311,-0.0327551936970413));
#12266=CARTESIAN_POINT('Ctrl Pts',(-6.99122327230096,314.338574056311,-1.9083995407149));
#12267=CARTESIAN_POINT('Ctrl Pts',(-6.04580022964255,314.476074056311,-3.52836682984752));
#12268=CARTESIAN_POINT('Ctrl Pts',(-5.10037718698415,314.613574056311,-5.14833411898014));
#12269=CARTESIAN_POINT('Ctrl Pts',(-3.47163317015249,314.751074056311,-6.07855542333959));
#12270=CARTESIAN_POINT('Ctrl Pts',(-1.84288915332082,314.888574056311,-7.00877672769905));
#12271=CARTESIAN_POINT('Ctrl Pts',(0.0327551936970409,315.026074056311,
-7.));
#12272=CARTESIAN_POINT('Ctrl Pts',(1.9083995407149,315.163574056311,-6.99122327230096));
#12273=CARTESIAN_POINT('Ctrl Pts',(3.52836682984752,315.301074056311,-6.04580022964255));
#12274=CARTESIAN_POINT('Ctrl Pts',(5.14833411898014,315.438574056311,-5.10037718698415));
#12275=CARTESIAN_POINT('Ctrl Pts',(6.07855542333959,315.576074056311,-3.47163317015249));
#12276=CARTESIAN_POINT('Ctrl Pts',(7.00877672769905,315.713574056311,-1.84288915332082));
#12277=CARTESIAN_POINT('Ctrl Pts',(7.,315.851074056311,0.0327551936970405));
#12278=CARTESIAN_POINT('Ctrl Pts',(6.99122327230096,315.988574056311,1.9083995407149));
#12279=CARTESIAN_POINT('Ctrl Pts',(6.04580022964255,316.126074056311,3.52836682984752));
#12280=CARTESIAN_POINT('Ctrl Pts',(5.10037718698415,316.263574056311,5.14833411898013));
#12281=CARTESIAN_POINT('Ctrl Pts',(3.47163317015249,316.401074056311,6.07855542333959));
#12282=CARTESIAN_POINT('Ctrl Pts',(1.84288915332082,316.538574056311,7.00877672769905));
#12283=CARTESIAN_POINT('Ctrl Pts',(-0.03275519369704,316.676074056311,7.));
#12284=CARTESIAN_POINT('Ctrl Pts',(-1.9083995407149,316.813574056311,6.99122327230096));
#12285=CARTESIAN_POINT('Ctrl Pts',(-3.52836682984752,316.951074056311,6.04580022964255));
#12286=CARTESIAN_POINT('Ctrl Pts',(-5.14833411898014,317.088574056311,5.10037718698415));
#12287=CARTESIAN_POINT('Ctrl Pts',(-6.07855542333959,317.226074056311,3.47163317015249));
#12288=CARTESIAN_POINT('Ctrl Pts',(-7.00877672769905,317.363574056311,1.84288915332082));
#12289=CARTESIAN_POINT('Ctrl Pts',(-7.,317.501074056311,-0.0327551936970413));
#12290=CARTESIAN_POINT('Ctrl Pts',(-8.,284.501074056311,-0.0327551936970314));
#12291=CARTESIAN_POINT('Ctrl Pts',(-7.99122327230096,284.638574056311,-2.17634873314601));
#12292=CARTESIAN_POINT('Ctrl Pts',(-6.911825633427,284.776074056311,-4.02836682984751));
#12293=CARTESIAN_POINT('Ctrl Pts',(-5.83242799455303,284.913574056311,-5.88038492654901));
#12294=CARTESIAN_POINT('Ctrl Pts',(-3.97163317015249,285.051074056311,-6.94458082712403));
#12295=CARTESIAN_POINT('Ctrl Pts',(-2.11083834575195,285.188574056311,-8.00877672769905));
#12296=CARTESIAN_POINT('Ctrl Pts',(0.0327551936970309,285.326074056311,
-8.));
#12297=CARTESIAN_POINT('Ctrl Pts',(2.17634873314601,285.463574056311,-7.99122327230096));
#12298=CARTESIAN_POINT('Ctrl Pts',(4.02836682984751,285.601074056311,-6.911825633427));
#12299=CARTESIAN_POINT('Ctrl Pts',(5.88038492654901,285.738574056311,-5.83242799455303));
#12300=CARTESIAN_POINT('Ctrl Pts',(6.94458082712403,285.876074056311,-3.9716331701525));
#12301=CARTESIAN_POINT('Ctrl Pts',(8.00877672769905,286.013574056311,-2.11083834575195));
#12302=CARTESIAN_POINT('Ctrl Pts',(8.,286.151074056311,0.0327551936970304));
#12303=CARTESIAN_POINT('Ctrl Pts',(7.99122327230096,286.288574056311,2.17634873314601));
#12304=CARTESIAN_POINT('Ctrl Pts',(6.911825633427,286.426074056311,4.02836682984751));
#12305=CARTESIAN_POINT('Ctrl Pts',(5.83242799455304,286.563574056311,5.880384926549));
#12306=CARTESIAN_POINT('Ctrl Pts',(3.9716331701525,286.701074056311,6.94458082712403));
#12307=CARTESIAN_POINT('Ctrl Pts',(2.11083834575196,286.838574056311,8.00877672769905));
#12308=CARTESIAN_POINT('Ctrl Pts',(-0.0327551936970299,286.976074056311,
8.));
#12309=CARTESIAN_POINT('Ctrl Pts',(-2.17634873314601,287.113574056311,7.99122327230096));
#12310=CARTESIAN_POINT('Ctrl Pts',(-4.02836682984751,287.251074056311,6.911825633427));
#12311=CARTESIAN_POINT('Ctrl Pts',(-5.88038492654901,287.388574056311,5.83242799455303));
#12312=CARTESIAN_POINT('Ctrl Pts',(-6.94458082712403,287.526074056311,3.9716331701525));
#12313=CARTESIAN_POINT('Ctrl Pts',(-8.00877672769905,287.663574056311,2.11083834575196));
#12314=CARTESIAN_POINT('Ctrl Pts',(-8.,287.801074056311,-0.0327551936970314));
#12315=CARTESIAN_POINT('Ctrl Pts',(-7.99122327230096,287.938574056311,-2.17634873314601));
#12316=CARTESIAN_POINT('Ctrl Pts',(-6.911825633427,288.076074056311,-4.02836682984751));
#12317=CARTESIAN_POINT('Ctrl Pts',(-5.83242799455303,288.213574056311,-5.88038492654901));
#12318=CARTESIAN_POINT('Ctrl Pts',(-3.97163317015249,288.351074056311,-6.94458082712403));
#12319=CARTESIAN_POINT('Ctrl Pts',(-2.11083834575195,288.488574056311,-8.00877672769905));
#12320=CARTESIAN_POINT('Ctrl Pts',(0.0327551936970309,288.626074056311,
-8.));
#12321=CARTESIAN_POINT('Ctrl Pts',(2.17634873314601,288.763574056311,-7.99122327230096));
#12322=CARTESIAN_POINT('Ctrl Pts',(4.02836682984751,288.901074056311,-6.911825633427));
#12323=CARTESIAN_POINT('Ctrl Pts',(5.88038492654901,289.038574056311,-5.83242799455303));
#12324=CARTESIAN_POINT('Ctrl Pts',(6.94458082712403,289.176074056311,-3.9716331701525));
#12325=CARTESIAN_POINT('Ctrl Pts',(8.00877672769905,289.313574056311,-2.11083834575195));
#12326=CARTESIAN_POINT('Ctrl Pts',(8.,289.451074056311,0.0327551936970304));
#12327=CARTESIAN_POINT('Ctrl Pts',(7.99122327230096,289.588574056311,2.17634873314601));
#12328=CARTESIAN_POINT('Ctrl Pts',(6.911825633427,289.726074056311,4.02836682984751));
#12329=CARTESIAN_POINT('Ctrl Pts',(5.83242799455304,289.863574056311,5.880384926549));
#12330=CARTESIAN_POINT('Ctrl Pts',(3.9716331701525,290.001074056311,6.94458082712403));
#12331=CARTESIAN_POINT('Ctrl Pts',(2.11083834575196,290.138574056311,8.00877672769905));
#12332=CARTESIAN_POINT('Ctrl Pts',(-0.0327551936970299,290.276074056311,
8.));
#12333=CARTESIAN_POINT('Ctrl Pts',(-2.17634873314601,290.413574056311,7.99122327230096));
#12334=CARTESIAN_POINT('Ctrl Pts',(-4.02836682984751,290.551074056311,6.911825633427));
#12335=CARTESIAN_POINT('Ctrl Pts',(-5.88038492654901,290.688574056311,5.83242799455303));
#12336=CARTESIAN_POINT('Ctrl Pts',(-6.94458082712403,290.826074056311,3.9716331701525));
#12337=CARTESIAN_POINT('Ctrl Pts',(-8.00877672769905,290.963574056311,2.11083834575196));
#12338=CARTESIAN_POINT('Ctrl Pts',(-8.,291.101074056311,-0.0327551936970314));
#12339=CARTESIAN_POINT('Ctrl Pts',(-7.99122327230096,291.238574056311,-2.17634873314601));
#12340=CARTESIAN_POINT('Ctrl Pts',(-6.911825633427,291.376074056311,-4.02836682984751));
#12341=CARTESIAN_POINT('Ctrl Pts',(-5.83242799455303,291.513574056311,-5.88038492654901));
#12342=CARTESIAN_POINT('Ctrl Pts',(-3.97163317015249,291.651074056311,-6.94458082712403));
#12343=CARTESIAN_POINT('Ctrl Pts',(-2.11083834575195,291.788574056311,-8.00877672769905));
#12344=CARTESIAN_POINT('Ctrl Pts',(0.0327551936970309,291.926074056311,
-8.));
#12345=CARTESIAN_POINT('Ctrl Pts',(2.17634873314601,292.063574056311,-7.99122327230096));
#12346=CARTESIAN_POINT('Ctrl Pts',(4.02836682984751,292.201074056311,-6.911825633427));
#12347=CARTESIAN_POINT('Ctrl Pts',(5.88038492654901,292.338574056311,-5.83242799455303));
#12348=CARTESIAN_POINT('Ctrl Pts',(6.94458082712403,292.476074056311,-3.9716331701525));
#12349=CARTESIAN_POINT('Ctrl Pts',(8.00877672769905,292.613574056311,-2.11083834575195));
#12350=CARTESIAN_POINT('Ctrl Pts',(8.,292.751074056311,0.0327551936970304));
#12351=CARTESIAN_POINT('Ctrl Pts',(7.99122327230096,292.888574056311,2.17634873314601));
#12352=CARTESIAN_POINT('Ctrl Pts',(6.911825633427,293.026074056311,4.02836682984751));
#12353=CARTESIAN_POINT('Ctrl Pts',(5.83242799455304,293.163574056311,5.880384926549));
#12354=CARTESIAN_POINT('Ctrl Pts',(3.9716331701525,293.301074056311,6.94458082712403));
#12355=CARTESIAN_POINT('Ctrl Pts',(2.11083834575196,293.438574056311,8.00877672769905));
#12356=CARTESIAN_POINT('Ctrl Pts',(-0.0327551936970299,293.576074056311,
8.));
#12357=CARTESIAN_POINT('Ctrl Pts',(-2.17634873314601,293.713574056311,7.99122327230096));
#12358=CARTESIAN_POINT('Ctrl Pts',(-4.02836682984751,293.851074056311,6.911825633427));
#12359=CARTESIAN_POINT('Ctrl Pts',(-5.88038492654901,293.988574056311,5.83242799455303));
#12360=CARTESIAN_POINT('Ctrl Pts',(-6.94458082712403,294.126074056311,3.9716331701525));
#12361=CARTESIAN_POINT('Ctrl Pts',(-8.00877672769905,294.263574056311,2.11083834575196));
#12362=CARTESIAN_POINT('Ctrl Pts',(-8.,294.401074056311,-0.0327551936970314));
#12363=CARTESIAN_POINT('Ctrl Pts',(-7.99122327230096,294.538574056311,-2.17634873314601));
#12364=CARTESIAN_POINT('Ctrl Pts',(-6.911825633427,294.676074056311,-4.02836682984751));
#12365=CARTESIAN_POINT('Ctrl Pts',(-5.83242799455303,294.813574056311,-5.88038492654901));
#12366=CARTESIAN_POINT('Ctrl Pts',(-3.97163317015249,294.951074056311,-6.94458082712403));
#12367=CARTESIAN_POINT('Ctrl Pts',(-2.11083834575195,295.088574056311,-8.00877672769905));
#12368=CARTESIAN_POINT('Ctrl Pts',(0.0327551936970309,295.226074056311,
-8.));
#12369=CARTESIAN_POINT('Ctrl Pts',(2.17634873314601,295.363574056311,-7.99122327230096));
#12370=CARTESIAN_POINT('Ctrl Pts',(4.02836682984751,295.501074056311,-6.911825633427));
#12371=CARTESIAN_POINT('Ctrl Pts',(5.88038492654901,295.638574056311,-5.83242799455303));
#12372=CARTESIAN_POINT('Ctrl Pts',(6.94458082712403,295.776074056311,-3.9716331701525));
#12373=CARTESIAN_POINT('Ctrl Pts',(8.00877672769905,295.913574056311,-2.11083834575195));
#12374=CARTESIAN_POINT('Ctrl Pts',(8.,296.051074056311,0.0327551936970304));
#12375=CARTESIAN_POINT('Ctrl Pts',(7.99122327230096,296.188574056311,2.17634873314601));
#12376=CARTESIAN_POINT('Ctrl Pts',(6.911825633427,296.326074056311,4.02836682984751));
#12377=CARTESIAN_POINT('Ctrl Pts',(5.83242799455304,296.463574056311,5.880384926549));
#12378=CARTESIAN_POINT('Ctrl Pts',(3.9716331701525,296.601074056311,6.94458082712403));
#12379=CARTESIAN_POINT('Ctrl Pts',(2.11083834575196,296.738574056311,8.00877672769905));
#12380=CARTESIAN_POINT('Ctrl Pts',(-0.0327551936970299,296.876074056311,
8.));
#12381=CARTESIAN_POINT('Ctrl Pts',(-2.17634873314601,297.013574056311,7.99122327230096));
#12382=CARTESIAN_POINT('Ctrl Pts',(-4.02836682984751,297.151074056311,6.911825633427));
#12383=CARTESIAN_POINT('Ctrl Pts',(-5.88038492654901,297.288574056311,5.83242799455303));
#12384=CARTESIAN_POINT('Ctrl Pts',(-6.94458082712403,297.426074056311,3.9716331701525));
#12385=CARTESIAN_POINT('Ctrl Pts',(-8.00877672769905,297.563574056311,2.11083834575196));
#12386=CARTESIAN_POINT('Ctrl Pts',(-8.,297.701074056311,-0.0327551936970314));
#12387=CARTESIAN_POINT('Ctrl Pts',(-7.99122327230096,297.838574056311,-2.17634873314601));
#12388=CARTESIAN_POINT('Ctrl Pts',(-6.911825633427,297.976074056311,-4.02836682984751));
#12389=CARTESIAN_POINT('Ctrl Pts',(-5.83242799455303,298.113574056311,-5.88038492654901));
#12390=CARTESIAN_POINT('Ctrl Pts',(-3.97163317015249,298.251074056311,-6.94458082712403));
#12391=CARTESIAN_POINT('Ctrl Pts',(-2.11083834575195,298.388574056311,-8.00877672769905));
#12392=CARTESIAN_POINT('Ctrl Pts',(0.0327551936970309,298.526074056311,
-8.));
#12393=CARTESIAN_POINT('Ctrl Pts',(2.17634873314601,298.663574056311,-7.99122327230096));
#12394=CARTESIAN_POINT('Ctrl Pts',(4.02836682984751,298.801074056311,-6.911825633427));
#12395=CARTESIAN_POINT('Ctrl Pts',(5.88038492654901,298.938574056311,-5.83242799455303));
#12396=CARTESIAN_POINT('Ctrl Pts',(6.94458082712403,299.076074056311,-3.9716331701525));
#12397=CARTESIAN_POINT('Ctrl Pts',(8.00877672769905,299.213574056311,-2.11083834575195));
#12398=CARTESIAN_POINT('Ctrl Pts',(8.,299.351074056311,0.0327551936970304));
#12399=CARTESIAN_POINT('Ctrl Pts',(7.99122327230096,299.488574056311,2.17634873314601));
#12400=CARTESIAN_POINT('Ctrl Pts',(6.911825633427,299.626074056311,4.02836682984751));
#12401=CARTESIAN_POINT('Ctrl Pts',(5.83242799455304,299.763574056311,5.880384926549));
#12402=CARTESIAN_POINT('Ctrl Pts',(3.9716331701525,299.901074056311,6.94458082712403));
#12403=CARTESIAN_POINT('Ctrl Pts',(2.11083834575196,300.038574056311,8.00877672769905));
#12404=CARTESIAN_POINT('Ctrl Pts',(-0.0327551936970299,300.176074056311,
8.));
#12405=CARTESIAN_POINT('Ctrl Pts',(-2.17634873314601,300.313574056311,7.99122327230096));
#12406=CARTESIAN_POINT('Ctrl Pts',(-4.02836682984751,300.451074056311,6.911825633427));
#12407=CARTESIAN_POINT('Ctrl Pts',(-5.88038492654901,300.588574056311,5.83242799455303));
#12408=CARTESIAN_POINT('Ctrl Pts',(-6.94458082712403,300.726074056311,3.9716331701525));
#12409=CARTESIAN_POINT('Ctrl Pts',(-8.00877672769905,300.863574056311,2.11083834575196));
#12410=CARTESIAN_POINT('Ctrl Pts',(-8.,301.001074056311,-0.0327551936970314));
#12411=CARTESIAN_POINT('Ctrl Pts',(-7.99122327230096,301.138574056311,-2.17634873314601));
#12412=CARTESIAN_POINT('Ctrl Pts',(-6.911825633427,301.276074056311,-4.02836682984751));
#12413=CARTESIAN_POINT('Ctrl Pts',(-5.83242799455303,301.413574056311,-5.88038492654901));
#12414=CARTESIAN_POINT('Ctrl Pts',(-3.97163317015249,301.551074056311,-6.94458082712403));
#12415=CARTESIAN_POINT('Ctrl Pts',(-2.11083834575195,301.688574056311,-8.00877672769905));
#12416=CARTESIAN_POINT('Ctrl Pts',(0.0327551936970309,301.826074056311,
-8.));
#12417=CARTESIAN_POINT('Ctrl Pts',(2.17634873314601,301.963574056311,-7.99122327230096));
#12418=CARTESIAN_POINT('Ctrl Pts',(4.02836682984751,302.101074056311,-6.911825633427));
#12419=CARTESIAN_POINT('Ctrl Pts',(5.88038492654901,302.238574056311,-5.83242799455303));
#12420=CARTESIAN_POINT('Ctrl Pts',(6.94458082712403,302.376074056311,-3.9716331701525));
#12421=CARTESIAN_POINT('Ctrl Pts',(8.00877672769905,302.513574056311,-2.11083834575195));
#12422=CARTESIAN_POINT('Ctrl Pts',(8.,302.651074056311,0.0327551936970304));
#12423=CARTESIAN_POINT('Ctrl Pts',(7.99122327230096,302.788574056311,2.17634873314601));
#12424=CARTESIAN_POINT('Ctrl Pts',(6.911825633427,302.926074056311,4.02836682984751));
#12425=CARTESIAN_POINT('Ctrl Pts',(5.83242799455304,303.063574056311,5.880384926549));
#12426=CARTESIAN_POINT('Ctrl Pts',(3.9716331701525,303.201074056311,6.94458082712403));
#12427=CARTESIAN_POINT('Ctrl Pts',(2.11083834575196,303.338574056311,8.00877672769905));
#12428=CARTESIAN_POINT('Ctrl Pts',(-0.0327551936970299,303.476074056311,
8.));
#12429=CARTESIAN_POINT('Ctrl Pts',(-2.17634873314601,303.613574056311,7.99122327230096));
#12430=CARTESIAN_POINT('Ctrl Pts',(-4.02836682984751,303.751074056311,6.911825633427));
#12431=CARTESIAN_POINT('Ctrl Pts',(-5.88038492654901,303.888574056311,5.83242799455303));
#12432=CARTESIAN_POINT('Ctrl Pts',(-6.94458082712403,304.026074056311,3.9716331701525));
#12433=CARTESIAN_POINT('Ctrl Pts',(-8.00877672769905,304.163574056311,2.11083834575196));
#12434=CARTESIAN_POINT('Ctrl Pts',(-8.,304.301074056311,-0.0327551936970314));
#12435=CARTESIAN_POINT('Ctrl Pts',(-7.99122327230096,304.438574056311,-2.17634873314601));
#12436=CARTESIAN_POINT('Ctrl Pts',(-6.911825633427,304.576074056311,-4.02836682984751));
#12437=CARTESIAN_POINT('Ctrl Pts',(-5.83242799455303,304.713574056311,-5.88038492654901));
#12438=CARTESIAN_POINT('Ctrl Pts',(-3.97163317015249,304.851074056311,-6.94458082712403));
#12439=CARTESIAN_POINT('Ctrl Pts',(-2.11083834575195,304.988574056311,-8.00877672769905));
#12440=CARTESIAN_POINT('Ctrl Pts',(0.0327551936970309,305.126074056311,
-8.));
#12441=CARTESIAN_POINT('Ctrl Pts',(2.17634873314601,305.263574056311,-7.99122327230096));
#12442=CARTESIAN_POINT('Ctrl Pts',(4.02836682984751,305.401074056311,-6.911825633427));
#12443=CARTESIAN_POINT('Ctrl Pts',(5.88038492654901,305.538574056311,-5.83242799455303));
#12444=CARTESIAN_POINT('Ctrl Pts',(6.94458082712403,305.676074056311,-3.9716331701525));
#12445=CARTESIAN_POINT('Ctrl Pts',(8.00877672769905,305.813574056311,-2.11083834575195));
#12446=CARTESIAN_POINT('Ctrl Pts',(8.,305.951074056311,0.0327551936970304));
#12447=CARTESIAN_POINT('Ctrl Pts',(7.99122327230096,306.088574056311,2.17634873314601));
#12448=CARTESIAN_POINT('Ctrl Pts',(6.911825633427,306.226074056311,4.02836682984751));
#12449=CARTESIAN_POINT('Ctrl Pts',(5.83242799455304,306.363574056311,5.880384926549));
#12450=CARTESIAN_POINT('Ctrl Pts',(3.9716331701525,306.501074056311,6.94458082712403));
#12451=CARTESIAN_POINT('Ctrl Pts',(2.11083834575196,306.638574056311,8.00877672769905));
#12452=CARTESIAN_POINT('Ctrl Pts',(-0.0327551936970299,306.776074056311,
8.));
#12453=CARTESIAN_POINT('Ctrl Pts',(-2.17634873314601,306.913574056311,7.99122327230096));
#12454=CARTESIAN_POINT('Ctrl Pts',(-4.02836682984751,307.051074056311,6.911825633427));
#12455=CARTESIAN_POINT('Ctrl Pts',(-5.88038492654901,307.188574056311,5.83242799455303));
#12456=CARTESIAN_POINT('Ctrl Pts',(-6.94458082712403,307.326074056311,3.9716331701525));
#12457=CARTESIAN_POINT('Ctrl Pts',(-8.00877672769905,307.463574056311,2.11083834575196));
#12458=CARTESIAN_POINT('Ctrl Pts',(-8.,307.601074056311,-0.0327551936970314));
#12459=CARTESIAN_POINT('Ctrl Pts',(-7.99122327230096,307.738574056311,-2.17634873314601));
#12460=CARTESIAN_POINT('Ctrl Pts',(-6.911825633427,307.876074056311,-4.02836682984751));
#12461=CARTESIAN_POINT('Ctrl Pts',(-5.83242799455303,308.013574056311,-5.88038492654901));
#12462=CARTESIAN_POINT('Ctrl Pts',(-3.97163317015249,308.151074056311,-6.94458082712403));
#12463=CARTESIAN_POINT('Ctrl Pts',(-2.11083834575195,308.288574056311,-8.00877672769905));
#12464=CARTESIAN_POINT('Ctrl Pts',(0.0327551936970309,308.426074056311,
-8.));
#12465=CARTESIAN_POINT('Ctrl Pts',(2.17634873314601,308.563574056311,-7.99122327230096));
#12466=CARTESIAN_POINT('Ctrl Pts',(4.02836682984751,308.701074056311,-6.911825633427));
#12467=CARTESIAN_POINT('Ctrl Pts',(5.88038492654901,308.838574056311,-5.83242799455303));
#12468=CARTESIAN_POINT('Ctrl Pts',(6.94458082712403,308.976074056311,-3.9716331701525));
#12469=CARTESIAN_POINT('Ctrl Pts',(8.00877672769905,309.113574056311,-2.11083834575195));
#12470=CARTESIAN_POINT('Ctrl Pts',(8.,309.251074056311,0.0327551936970304));
#12471=CARTESIAN_POINT('Ctrl Pts',(7.99122327230096,309.388574056311,2.17634873314601));
#12472=CARTESIAN_POINT('Ctrl Pts',(6.911825633427,309.526074056311,4.02836682984751));
#12473=CARTESIAN_POINT('Ctrl Pts',(5.83242799455304,309.663574056311,5.880384926549));
#12474=CARTESIAN_POINT('Ctrl Pts',(3.9716331701525,309.801074056311,6.94458082712403));
#12475=CARTESIAN_POINT('Ctrl Pts',(2.11083834575196,309.938574056311,8.00877672769905));
#12476=CARTESIAN_POINT('Ctrl Pts',(-0.0327551936970299,310.076074056311,
8.));
#12477=CARTESIAN_POINT('Ctrl Pts',(-2.17634873314601,310.213574056311,7.99122327230096));
#12478=CARTESIAN_POINT('Ctrl Pts',(-4.02836682984751,310.351074056311,6.911825633427));
#12479=CARTESIAN_POINT('Ctrl Pts',(-5.88038492654901,310.488574056311,5.83242799455303));
#12480=CARTESIAN_POINT('Ctrl Pts',(-6.94458082712403,310.626074056311,3.9716331701525));
#12481=CARTESIAN_POINT('Ctrl Pts',(-8.00877672769905,310.763574056311,2.11083834575196));
#12482=CARTESIAN_POINT('Ctrl Pts',(-8.,310.901074056311,-0.0327551936970314));
#12483=CARTESIAN_POINT('Ctrl Pts',(-7.99122327230096,311.038574056311,-2.17634873314601));
#12484=CARTESIAN_POINT('Ctrl Pts',(-6.911825633427,311.176074056311,-4.02836682984751));
#12485=CARTESIAN_POINT('Ctrl Pts',(-5.83242799455303,311.313574056311,-5.88038492654901));
#12486=CARTESIAN_POINT('Ctrl Pts',(-3.97163317015249,311.451074056311,-6.94458082712403));
#12487=CARTESIAN_POINT('Ctrl Pts',(-2.11083834575195,311.588574056311,-8.00877672769905));
#12488=CARTESIAN_POINT('Ctrl Pts',(0.0327551936970309,311.726074056311,
-8.));
#12489=CARTESIAN_POINT('Ctrl Pts',(2.17634873314601,311.863574056311,-7.99122327230096));
#12490=CARTESIAN_POINT('Ctrl Pts',(4.02836682984751,312.001074056311,-6.911825633427));
#12491=CARTESIAN_POINT('Ctrl Pts',(5.88038492654901,312.138574056311,-5.83242799455303));
#12492=CARTESIAN_POINT('Ctrl Pts',(6.94458082712403,312.276074056311,-3.9716331701525));
#12493=CARTESIAN_POINT('Ctrl Pts',(8.00877672769905,312.413574056311,-2.11083834575195));
#12494=CARTESIAN_POINT('Ctrl Pts',(8.,312.551074056311,0.0327551936970304));
#12495=CARTESIAN_POINT('Ctrl Pts',(7.99122327230096,312.688574056311,2.17634873314601));
#12496=CARTESIAN_POINT('Ctrl Pts',(6.911825633427,312.826074056311,4.02836682984751));
#12497=CARTESIAN_POINT('Ctrl Pts',(5.83242799455304,312.963574056311,5.880384926549));
#12498=CARTESIAN_POINT('Ctrl Pts',(3.9716331701525,313.101074056311,6.94458082712403));
#12499=CARTESIAN_POINT('Ctrl Pts',(2.11083834575196,313.238574056311,8.00877672769905));
#12500=CARTESIAN_POINT('Ctrl Pts',(-0.0327551936970299,313.376074056311,
8.));
#12501=CARTESIAN_POINT('Ctrl Pts',(-2.17634873314601,313.513574056311,7.99122327230096));
#12502=CARTESIAN_POINT('Ctrl Pts',(-4.02836682984751,313.651074056311,6.911825633427));
#12503=CARTESIAN_POINT('Ctrl Pts',(-5.88038492654901,313.788574056311,5.83242799455303));
#12504=CARTESIAN_POINT('Ctrl Pts',(-6.94458082712403,313.926074056311,3.9716331701525));
#12505=CARTESIAN_POINT('Ctrl Pts',(-8.00877672769905,314.063574056311,2.11083834575196));
#12506=CARTESIAN_POINT('Ctrl Pts',(-8.,314.201074056311,-0.0327551936970314));
#12507=CARTESIAN_POINT('Ctrl Pts',(-7.99122327230096,314.338574056311,-2.17634873314601));
#12508=CARTESIAN_POINT('Ctrl Pts',(-6.911825633427,314.476074056311,-4.02836682984751));
#12509=CARTESIAN_POINT('Ctrl Pts',(-5.83242799455303,314.613574056311,-5.88038492654901));
#12510=CARTESIAN_POINT('Ctrl Pts',(-3.97163317015249,314.751074056311,-6.94458082712403));
#12511=CARTESIAN_POINT('Ctrl Pts',(-2.11083834575195,314.888574056311,-8.00877672769905));
#12512=CARTESIAN_POINT('Ctrl Pts',(0.0327551936970309,315.026074056311,
-8.));
#12513=CARTESIAN_POINT('Ctrl Pts',(2.17634873314601,315.163574056311,-7.99122327230096));
#12514=CARTESIAN_POINT('Ctrl Pts',(4.02836682984751,315.301074056311,-6.911825633427));
#12515=CARTESIAN_POINT('Ctrl Pts',(5.88038492654901,315.438574056311,-5.83242799455303));
#12516=CARTESIAN_POINT('Ctrl Pts',(6.94458082712403,315.576074056311,-3.9716331701525));
#12517=CARTESIAN_POINT('Ctrl Pts',(8.00877672769905,315.713574056311,-2.11083834575195));
#12518=CARTESIAN_POINT('Ctrl Pts',(8.,315.851074056311,0.0327551936970304));
#12519=CARTESIAN_POINT('Ctrl Pts',(7.99122327230096,315.988574056311,2.17634873314601));
#12520=CARTESIAN_POINT('Ctrl Pts',(6.911825633427,316.126074056311,4.02836682984751));
#12521=CARTESIAN_POINT('Ctrl Pts',(5.83242799455304,316.263574056311,5.880384926549));
#12522=CARTESIAN_POINT('Ctrl Pts',(3.9716331701525,316.401074056311,6.94458082712403));
#12523=CARTESIAN_POINT('Ctrl Pts',(2.11083834575196,316.538574056311,8.00877672769905));
#12524=CARTESIAN_POINT('Ctrl Pts',(-0.0327551936970299,316.676074056311,
8.));
#12525=CARTESIAN_POINT('Ctrl Pts',(-2.17634873314601,316.813574056311,7.99122327230096));
#12526=CARTESIAN_POINT('Ctrl Pts',(-4.02836682984751,316.951074056311,6.911825633427));
#12527=CARTESIAN_POINT('Ctrl Pts',(-5.88038492654901,317.088574056311,5.83242799455303));
#12528=CARTESIAN_POINT('Ctrl Pts',(-6.94458082712403,317.226074056311,3.9716331701525));
#12529=CARTESIAN_POINT('Ctrl Pts',(-8.00877672769905,317.363574056311,2.11083834575196));
#12530=CARTESIAN_POINT('Ctrl Pts',(-8.,317.501074056311,-0.0327551936970314));
#12531=CARTESIAN_POINT('Ctrl Pts',(-9.,284.501074056311,-0.0327551936970214));
#12532=CARTESIAN_POINT('Ctrl Pts',(-8.99122327230096,284.638574056311,-2.44429792557713));
#12533=CARTESIAN_POINT('Ctrl Pts',(-7.77785103721144,284.776074056311,-4.5283668298475));
#12534=CARTESIAN_POINT('Ctrl Pts',(-6.56447880212192,284.913574056311,-6.61243573411788));
#12535=CARTESIAN_POINT('Ctrl Pts',(-4.4716331701525,285.051074056311,-7.81060623090846));
#12536=CARTESIAN_POINT('Ctrl Pts',(-2.37878753818309,285.188574056311,-9.00877672769904));
#12537=CARTESIAN_POINT('Ctrl Pts',(0.0327551936970209,285.326074056311,
-9.));
#12538=CARTESIAN_POINT('Ctrl Pts',(2.44429792557713,285.463574056311,-8.99122327230096));
#12539=CARTESIAN_POINT('Ctrl Pts',(4.5283668298475,285.601074056311,-7.77785103721144));
#12540=CARTESIAN_POINT('Ctrl Pts',(6.61243573411788,285.738574056311,-6.56447880212192));
#12541=CARTESIAN_POINT('Ctrl Pts',(7.81060623090846,285.876074056311,-4.4716331701525));
#12542=CARTESIAN_POINT('Ctrl Pts',(9.00877672769904,286.013574056311,-2.37878753818309));
#12543=CARTESIAN_POINT('Ctrl Pts',(9.,286.151074056311,0.0327551936970203));
#12544=CARTESIAN_POINT('Ctrl Pts',(8.99122327230096,286.288574056311,2.44429792557712));
#12545=CARTESIAN_POINT('Ctrl Pts',(7.77785103721144,286.426074056311,4.5283668298475));
#12546=CARTESIAN_POINT('Ctrl Pts',(6.56447880212192,286.563574056311,6.61243573411788));
#12547=CARTESIAN_POINT('Ctrl Pts',(4.47163317015251,286.701074056311,7.81060623090846));
#12548=CARTESIAN_POINT('Ctrl Pts',(2.37878753818309,286.838574056311,9.00877672769904));
#12549=CARTESIAN_POINT('Ctrl Pts',(-0.0327551936970198,286.976074056311,
9.));
#12550=CARTESIAN_POINT('Ctrl Pts',(-2.44429792557712,287.113574056311,8.99122327230096));
#12551=CARTESIAN_POINT('Ctrl Pts',(-4.5283668298475,287.251074056311,7.77785103721144));
#12552=CARTESIAN_POINT('Ctrl Pts',(-6.61243573411788,287.388574056311,6.56447880212192));
#12553=CARTESIAN_POINT('Ctrl Pts',(-7.81060623090846,287.526074056311,4.47163317015251));
#12554=CARTESIAN_POINT('Ctrl Pts',(-9.00877672769904,287.663574056311,2.37878753818309));
#12555=CARTESIAN_POINT('Ctrl Pts',(-9.,287.801074056311,-0.0327551936970214));
#12556=CARTESIAN_POINT('Ctrl Pts',(-8.99122327230096,287.938574056311,-2.44429792557713));
#12557=CARTESIAN_POINT('Ctrl Pts',(-7.77785103721144,288.076074056311,-4.5283668298475));
#12558=CARTESIAN_POINT('Ctrl Pts',(-6.56447880212192,288.213574056311,-6.61243573411788));
#12559=CARTESIAN_POINT('Ctrl Pts',(-4.4716331701525,288.351074056311,-7.81060623090846));
#12560=CARTESIAN_POINT('Ctrl Pts',(-2.37878753818309,288.488574056311,-9.00877672769904));
#12561=CARTESIAN_POINT('Ctrl Pts',(0.0327551936970209,288.626074056311,
-9.));
#12562=CARTESIAN_POINT('Ctrl Pts',(2.44429792557713,288.763574056311,-8.99122327230096));
#12563=CARTESIAN_POINT('Ctrl Pts',(4.5283668298475,288.901074056311,-7.77785103721144));
#12564=CARTESIAN_POINT('Ctrl Pts',(6.61243573411788,289.038574056311,-6.56447880212192));
#12565=CARTESIAN_POINT('Ctrl Pts',(7.81060623090846,289.176074056311,-4.4716331701525));
#12566=CARTESIAN_POINT('Ctrl Pts',(9.00877672769904,289.313574056311,-2.37878753818309));
#12567=CARTESIAN_POINT('Ctrl Pts',(9.,289.451074056311,0.0327551936970203));
#12568=CARTESIAN_POINT('Ctrl Pts',(8.99122327230096,289.588574056311,2.44429792557712));
#12569=CARTESIAN_POINT('Ctrl Pts',(7.77785103721144,289.726074056311,4.5283668298475));
#12570=CARTESIAN_POINT('Ctrl Pts',(6.56447880212192,289.863574056311,6.61243573411788));
#12571=CARTESIAN_POINT('Ctrl Pts',(4.47163317015251,290.001074056311,7.81060623090846));
#12572=CARTESIAN_POINT('Ctrl Pts',(2.37878753818309,290.138574056311,9.00877672769904));
#12573=CARTESIAN_POINT('Ctrl Pts',(-0.0327551936970198,290.276074056311,
9.));
#12574=CARTESIAN_POINT('Ctrl Pts',(-2.44429792557712,290.413574056311,8.99122327230096));
#12575=CARTESIAN_POINT('Ctrl Pts',(-4.5283668298475,290.551074056311,7.77785103721144));
#12576=CARTESIAN_POINT('Ctrl Pts',(-6.61243573411788,290.688574056311,6.56447880212192));
#12577=CARTESIAN_POINT('Ctrl Pts',(-7.81060623090846,290.826074056311,4.47163317015251));
#12578=CARTESIAN_POINT('Ctrl Pts',(-9.00877672769904,290.963574056311,2.37878753818309));
#12579=CARTESIAN_POINT('Ctrl Pts',(-9.,291.101074056311,-0.0327551936970214));
#12580=CARTESIAN_POINT('Ctrl Pts',(-8.99122327230096,291.238574056311,-2.44429792557713));
#12581=CARTESIAN_POINT('Ctrl Pts',(-7.77785103721144,291.376074056311,-4.5283668298475));
#12582=CARTESIAN_POINT('Ctrl Pts',(-6.56447880212192,291.513574056311,-6.61243573411788));
#12583=CARTESIAN_POINT('Ctrl Pts',(-4.4716331701525,291.651074056311,-7.81060623090846));
#12584=CARTESIAN_POINT('Ctrl Pts',(-2.37878753818309,291.788574056311,-9.00877672769904));
#12585=CARTESIAN_POINT('Ctrl Pts',(0.0327551936970209,291.926074056311,
-9.));
#12586=CARTESIAN_POINT('Ctrl Pts',(2.44429792557713,292.063574056311,-8.99122327230096));
#12587=CARTESIAN_POINT('Ctrl Pts',(4.5283668298475,292.201074056311,-7.77785103721144));
#12588=CARTESIAN_POINT('Ctrl Pts',(6.61243573411788,292.338574056311,-6.56447880212192));
#12589=CARTESIAN_POINT('Ctrl Pts',(7.81060623090846,292.476074056311,-4.4716331701525));
#12590=CARTESIAN_POINT('Ctrl Pts',(9.00877672769904,292.613574056311,-2.37878753818309));
#12591=CARTESIAN_POINT('Ctrl Pts',(9.,292.751074056311,0.0327551936970203));
#12592=CARTESIAN_POINT('Ctrl Pts',(8.99122327230096,292.888574056311,2.44429792557712));
#12593=CARTESIAN_POINT('Ctrl Pts',(7.77785103721144,293.026074056311,4.5283668298475));
#12594=CARTESIAN_POINT('Ctrl Pts',(6.56447880212192,293.163574056311,6.61243573411788));
#12595=CARTESIAN_POINT('Ctrl Pts',(4.47163317015251,293.301074056311,7.81060623090846));
#12596=CARTESIAN_POINT('Ctrl Pts',(2.37878753818309,293.438574056311,9.00877672769904));
#12597=CARTESIAN_POINT('Ctrl Pts',(-0.0327551936970198,293.576074056311,
9.));
#12598=CARTESIAN_POINT('Ctrl Pts',(-2.44429792557712,293.713574056311,8.99122327230096));
#12599=CARTESIAN_POINT('Ctrl Pts',(-4.5283668298475,293.851074056311,7.77785103721144));
#12600=CARTESIAN_POINT('Ctrl Pts',(-6.61243573411788,293.988574056311,6.56447880212192));
#12601=CARTESIAN_POINT('Ctrl Pts',(-7.81060623090846,294.126074056311,4.47163317015251));
#12602=CARTESIAN_POINT('Ctrl Pts',(-9.00877672769904,294.263574056311,2.37878753818309));
#12603=CARTESIAN_POINT('Ctrl Pts',(-9.,294.401074056311,-0.0327551936970214));
#12604=CARTESIAN_POINT('Ctrl Pts',(-8.99122327230096,294.538574056311,-2.44429792557713));
#12605=CARTESIAN_POINT('Ctrl Pts',(-7.77785103721144,294.676074056311,-4.5283668298475));
#12606=CARTESIAN_POINT('Ctrl Pts',(-6.56447880212192,294.813574056311,-6.61243573411788));
#12607=CARTESIAN_POINT('Ctrl Pts',(-4.4716331701525,294.951074056311,-7.81060623090846));
#12608=CARTESIAN_POINT('Ctrl Pts',(-2.37878753818309,295.088574056311,-9.00877672769904));
#12609=CARTESIAN_POINT('Ctrl Pts',(0.0327551936970209,295.226074056311,
-9.));
#12610=CARTESIAN_POINT('Ctrl Pts',(2.44429792557713,295.363574056311,-8.99122327230096));
#12611=CARTESIAN_POINT('Ctrl Pts',(4.5283668298475,295.501074056311,-7.77785103721144));
#12612=CARTESIAN_POINT('Ctrl Pts',(6.61243573411788,295.638574056311,-6.56447880212192));
#12613=CARTESIAN_POINT('Ctrl Pts',(7.81060623090846,295.776074056311,-4.4716331701525));
#12614=CARTESIAN_POINT('Ctrl Pts',(9.00877672769904,295.913574056311,-2.37878753818309));
#12615=CARTESIAN_POINT('Ctrl Pts',(9.,296.051074056311,0.0327551936970203));
#12616=CARTESIAN_POINT('Ctrl Pts',(8.99122327230096,296.188574056311,2.44429792557712));
#12617=CARTESIAN_POINT('Ctrl Pts',(7.77785103721144,296.326074056311,4.5283668298475));
#12618=CARTESIAN_POINT('Ctrl Pts',(6.56447880212192,296.463574056311,6.61243573411788));
#12619=CARTESIAN_POINT('Ctrl Pts',(4.47163317015251,296.601074056311,7.81060623090846));
#12620=CARTESIAN_POINT('Ctrl Pts',(2.37878753818309,296.738574056311,9.00877672769904));
#12621=CARTESIAN_POINT('Ctrl Pts',(-0.0327551936970198,296.876074056311,
9.));
#12622=CARTESIAN_POINT('Ctrl Pts',(-2.44429792557712,297.013574056311,8.99122327230096));
#12623=CARTESIAN_POINT('Ctrl Pts',(-4.5283668298475,297.151074056311,7.77785103721144));
#12624=CARTESIAN_POINT('Ctrl Pts',(-6.61243573411788,297.288574056311,6.56447880212192));
#12625=CARTESIAN_POINT('Ctrl Pts',(-7.81060623090846,297.426074056311,4.47163317015251));
#12626=CARTESIAN_POINT('Ctrl Pts',(-9.00877672769904,297.563574056311,2.37878753818309));
#12627=CARTESIAN_POINT('Ctrl Pts',(-9.,297.701074056311,-0.0327551936970214));
#12628=CARTESIAN_POINT('Ctrl Pts',(-8.99122327230096,297.838574056311,-2.44429792557713));
#12629=CARTESIAN_POINT('Ctrl Pts',(-7.77785103721144,297.976074056311,-4.5283668298475));
#12630=CARTESIAN_POINT('Ctrl Pts',(-6.56447880212192,298.113574056311,-6.61243573411788));
#12631=CARTESIAN_POINT('Ctrl Pts',(-4.4716331701525,298.251074056311,-7.81060623090846));
#12632=CARTESIAN_POINT('Ctrl Pts',(-2.37878753818309,298.388574056311,-9.00877672769904));
#12633=CARTESIAN_POINT('Ctrl Pts',(0.0327551936970209,298.526074056311,
-9.));
#12634=CARTESIAN_POINT('Ctrl Pts',(2.44429792557713,298.663574056311,-8.99122327230096));
#12635=CARTESIAN_POINT('Ctrl Pts',(4.5283668298475,298.801074056311,-7.77785103721144));
#12636=CARTESIAN_POINT('Ctrl Pts',(6.61243573411788,298.938574056311,-6.56447880212192));
#12637=CARTESIAN_POINT('Ctrl Pts',(7.81060623090846,299.076074056311,-4.4716331701525));
#12638=CARTESIAN_POINT('Ctrl Pts',(9.00877672769904,299.213574056311,-2.37878753818309));
#12639=CARTESIAN_POINT('Ctrl Pts',(9.,299.351074056311,0.0327551936970203));
#12640=CARTESIAN_POINT('Ctrl Pts',(8.99122327230096,299.488574056311,2.44429792557712));
#12641=CARTESIAN_POINT('Ctrl Pts',(7.77785103721144,299.626074056311,4.5283668298475));
#12642=CARTESIAN_POINT('Ctrl Pts',(6.56447880212192,299.763574056311,6.61243573411788));
#12643=CARTESIAN_POINT('Ctrl Pts',(4.47163317015251,299.901074056311,7.81060623090846));
#12644=CARTESIAN_POINT('Ctrl Pts',(2.37878753818309,300.038574056311,9.00877672769904));
#12645=CARTESIAN_POINT('Ctrl Pts',(-0.0327551936970198,300.176074056311,
9.));
#12646=CARTESIAN_POINT('Ctrl Pts',(-2.44429792557712,300.313574056311,8.99122327230096));
#12647=CARTESIAN_POINT('Ctrl Pts',(-4.5283668298475,300.451074056311,7.77785103721144));
#12648=CARTESIAN_POINT('Ctrl Pts',(-6.61243573411788,300.588574056311,6.56447880212192));
#12649=CARTESIAN_POINT('Ctrl Pts',(-7.81060623090846,300.726074056311,4.47163317015251));
#12650=CARTESIAN_POINT('Ctrl Pts',(-9.00877672769904,300.863574056311,2.37878753818309));
#12651=CARTESIAN_POINT('Ctrl Pts',(-9.,301.001074056311,-0.0327551936970214));
#12652=CARTESIAN_POINT('Ctrl Pts',(-8.99122327230096,301.138574056311,-2.44429792557713));
#12653=CARTESIAN_POINT('Ctrl Pts',(-7.77785103721144,301.276074056311,-4.5283668298475));
#12654=CARTESIAN_POINT('Ctrl Pts',(-6.56447880212192,301.413574056311,-6.61243573411788));
#12655=CARTESIAN_POINT('Ctrl Pts',(-4.4716331701525,301.551074056311,-7.81060623090846));
#12656=CARTESIAN_POINT('Ctrl Pts',(-2.37878753818309,301.688574056311,-9.00877672769904));
#12657=CARTESIAN_POINT('Ctrl Pts',(0.0327551936970209,301.826074056311,
-9.));
#12658=CARTESIAN_POINT('Ctrl Pts',(2.44429792557713,301.963574056311,-8.99122327230096));
#12659=CARTESIAN_POINT('Ctrl Pts',(4.5283668298475,302.101074056311,-7.77785103721144));
#12660=CARTESIAN_POINT('Ctrl Pts',(6.61243573411788,302.238574056311,-6.56447880212192));
#12661=CARTESIAN_POINT('Ctrl Pts',(7.81060623090846,302.376074056311,-4.4716331701525));
#12662=CARTESIAN_POINT('Ctrl Pts',(9.00877672769904,302.513574056311,-2.37878753818309));
#12663=CARTESIAN_POINT('Ctrl Pts',(9.,302.651074056311,0.0327551936970203));
#12664=CARTESIAN_POINT('Ctrl Pts',(8.99122327230096,302.788574056311,2.44429792557712));
#12665=CARTESIAN_POINT('Ctrl Pts',(7.77785103721144,302.926074056311,4.5283668298475));
#12666=CARTESIAN_POINT('Ctrl Pts',(6.56447880212192,303.063574056311,6.61243573411788));
#12667=CARTESIAN_POINT('Ctrl Pts',(4.47163317015251,303.201074056311,7.81060623090846));
#12668=CARTESIAN_POINT('Ctrl Pts',(2.37878753818309,303.338574056311,9.00877672769904));
#12669=CARTESIAN_POINT('Ctrl Pts',(-0.0327551936970198,303.476074056311,
9.));
#12670=CARTESIAN_POINT('Ctrl Pts',(-2.44429792557712,303.613574056311,8.99122327230096));
#12671=CARTESIAN_POINT('Ctrl Pts',(-4.5283668298475,303.751074056311,7.77785103721144));
#12672=CARTESIAN_POINT('Ctrl Pts',(-6.61243573411788,303.888574056311,6.56447880212192));
#12673=CARTESIAN_POINT('Ctrl Pts',(-7.81060623090846,304.026074056311,4.47163317015251));
#12674=CARTESIAN_POINT('Ctrl Pts',(-9.00877672769904,304.163574056311,2.37878753818309));
#12675=CARTESIAN_POINT('Ctrl Pts',(-9.,304.301074056311,-0.0327551936970214));
#12676=CARTESIAN_POINT('Ctrl Pts',(-8.99122327230096,304.438574056311,-2.44429792557713));
#12677=CARTESIAN_POINT('Ctrl Pts',(-7.77785103721144,304.576074056311,-4.5283668298475));
#12678=CARTESIAN_POINT('Ctrl Pts',(-6.56447880212192,304.713574056311,-6.61243573411788));
#12679=CARTESIAN_POINT('Ctrl Pts',(-4.4716331701525,304.851074056311,-7.81060623090846));
#12680=CARTESIAN_POINT('Ctrl Pts',(-2.37878753818309,304.988574056311,-9.00877672769904));
#12681=CARTESIAN_POINT('Ctrl Pts',(0.0327551936970209,305.126074056311,
-9.));
#12682=CARTESIAN_POINT('Ctrl Pts',(2.44429792557713,305.263574056311,-8.99122327230096));
#12683=CARTESIAN_POINT('Ctrl Pts',(4.5283668298475,305.401074056311,-7.77785103721144));
#12684=CARTESIAN_POINT('Ctrl Pts',(6.61243573411788,305.538574056311,-6.56447880212192));
#12685=CARTESIAN_POINT('Ctrl Pts',(7.81060623090846,305.676074056311,-4.4716331701525));
#12686=CARTESIAN_POINT('Ctrl Pts',(9.00877672769904,305.813574056311,-2.37878753818309));
#12687=CARTESIAN_POINT('Ctrl Pts',(9.,305.951074056311,0.0327551936970203));
#12688=CARTESIAN_POINT('Ctrl Pts',(8.99122327230096,306.088574056311,2.44429792557712));
#12689=CARTESIAN_POINT('Ctrl Pts',(7.77785103721144,306.226074056311,4.5283668298475));
#12690=CARTESIAN_POINT('Ctrl Pts',(6.56447880212192,306.363574056311,6.61243573411788));
#12691=CARTESIAN_POINT('Ctrl Pts',(4.47163317015251,306.501074056311,7.81060623090846));
#12692=CARTESIAN_POINT('Ctrl Pts',(2.37878753818309,306.638574056311,9.00877672769904));
#12693=CARTESIAN_POINT('Ctrl Pts',(-0.0327551936970198,306.776074056311,
9.));
#12694=CARTESIAN_POINT('Ctrl Pts',(-2.44429792557712,306.913574056311,8.99122327230096));
#12695=CARTESIAN_POINT('Ctrl Pts',(-4.5283668298475,307.051074056311,7.77785103721144));
#12696=CARTESIAN_POINT('Ctrl Pts',(-6.61243573411788,307.188574056311,6.56447880212192));
#12697=CARTESIAN_POINT('Ctrl Pts',(-7.81060623090846,307.326074056311,4.47163317015251));
#12698=CARTESIAN_POINT('Ctrl Pts',(-9.00877672769904,307.463574056311,2.37878753818309));
#12699=CARTESIAN_POINT('Ctrl Pts',(-9.,307.601074056311,-0.0327551936970214));
#12700=CARTESIAN_POINT('Ctrl Pts',(-8.99122327230096,307.738574056311,-2.44429792557713));
#12701=CARTESIAN_POINT('Ctrl Pts',(-7.77785103721144,307.876074056311,-4.5283668298475));
#12702=CARTESIAN_POINT('Ctrl Pts',(-6.56447880212192,308.013574056311,-6.61243573411788));
#12703=CARTESIAN_POINT('Ctrl Pts',(-4.4716331701525,308.151074056311,-7.81060623090846));
#12704=CARTESIAN_POINT('Ctrl Pts',(-2.37878753818309,308.288574056311,-9.00877672769904));
#12705=CARTESIAN_POINT('Ctrl Pts',(0.0327551936970209,308.426074056311,
-9.));
#12706=CARTESIAN_POINT('Ctrl Pts',(2.44429792557713,308.563574056311,-8.99122327230096));
#12707=CARTESIAN_POINT('Ctrl Pts',(4.5283668298475,308.701074056311,-7.77785103721144));
#12708=CARTESIAN_POINT('Ctrl Pts',(6.61243573411788,308.838574056311,-6.56447880212192));
#12709=CARTESIAN_POINT('Ctrl Pts',(7.81060623090846,308.976074056311,-4.4716331701525));
#12710=CARTESIAN_POINT('Ctrl Pts',(9.00877672769904,309.113574056311,-2.37878753818309));
#12711=CARTESIAN_POINT('Ctrl Pts',(9.,309.251074056311,0.0327551936970203));
#12712=CARTESIAN_POINT('Ctrl Pts',(8.99122327230096,309.388574056311,2.44429792557712));
#12713=CARTESIAN_POINT('Ctrl Pts',(7.77785103721144,309.526074056311,4.5283668298475));
#12714=CARTESIAN_POINT('Ctrl Pts',(6.56447880212192,309.663574056311,6.61243573411788));
#12715=CARTESIAN_POINT('Ctrl Pts',(4.47163317015251,309.801074056311,7.81060623090846));
#12716=CARTESIAN_POINT('Ctrl Pts',(2.37878753818309,309.938574056311,9.00877672769904));
#12717=CARTESIAN_POINT('Ctrl Pts',(-0.0327551936970198,310.076074056311,
9.));
#12718=CARTESIAN_POINT('Ctrl Pts',(-2.44429792557712,310.213574056311,8.99122327230096));
#12719=CARTESIAN_POINT('Ctrl Pts',(-4.5283668298475,310.351074056311,7.77785103721144));
#12720=CARTESIAN_POINT('Ctrl Pts',(-6.61243573411788,310.488574056311,6.56447880212192));
#12721=CARTESIAN_POINT('Ctrl Pts',(-7.81060623090846,310.626074056311,4.47163317015251));
#12722=CARTESIAN_POINT('Ctrl Pts',(-9.00877672769904,310.763574056311,2.37878753818309));
#12723=CARTESIAN_POINT('Ctrl Pts',(-9.,310.901074056311,-0.0327551936970214));
#12724=CARTESIAN_POINT('Ctrl Pts',(-8.99122327230096,311.038574056311,-2.44429792557713));
#12725=CARTESIAN_POINT('Ctrl Pts',(-7.77785103721144,311.176074056311,-4.5283668298475));
#12726=CARTESIAN_POINT('Ctrl Pts',(-6.56447880212192,311.313574056311,-6.61243573411788));
#12727=CARTESIAN_POINT('Ctrl Pts',(-4.4716331701525,311.451074056311,-7.81060623090846));
#12728=CARTESIAN_POINT('Ctrl Pts',(-2.37878753818309,311.588574056311,-9.00877672769904));
#12729=CARTESIAN_POINT('Ctrl Pts',(0.0327551936970209,311.726074056311,
-9.));
#12730=CARTESIAN_POINT('Ctrl Pts',(2.44429792557713,311.863574056311,-8.99122327230096));
#12731=CARTESIAN_POINT('Ctrl Pts',(4.5283668298475,312.001074056311,-7.77785103721144));
#12732=CARTESIAN_POINT('Ctrl Pts',(6.61243573411788,312.138574056311,-6.56447880212192));
#12733=CARTESIAN_POINT('Ctrl Pts',(7.81060623090846,312.276074056311,-4.4716331701525));
#12734=CARTESIAN_POINT('Ctrl Pts',(9.00877672769904,312.413574056311,-2.37878753818309));
#12735=CARTESIAN_POINT('Ctrl Pts',(9.,312.551074056311,0.0327551936970203));
#12736=CARTESIAN_POINT('Ctrl Pts',(8.99122327230096,312.688574056311,2.44429792557712));
#12737=CARTESIAN_POINT('Ctrl Pts',(7.77785103721144,312.826074056311,4.5283668298475));
#12738=CARTESIAN_POINT('Ctrl Pts',(6.56447880212192,312.963574056311,6.61243573411788));
#12739=CARTESIAN_POINT('Ctrl Pts',(4.47163317015251,313.101074056311,7.81060623090846));
#12740=CARTESIAN_POINT('Ctrl Pts',(2.37878753818309,313.238574056311,9.00877672769904));
#12741=CARTESIAN_POINT('Ctrl Pts',(-0.0327551936970198,313.376074056311,
9.));
#12742=CARTESIAN_POINT('Ctrl Pts',(-2.44429792557712,313.513574056311,8.99122327230096));
#12743=CARTESIAN_POINT('Ctrl Pts',(-4.5283668298475,313.651074056311,7.77785103721144));
#12744=CARTESIAN_POINT('Ctrl Pts',(-6.61243573411788,313.788574056311,6.56447880212192));
#12745=CARTESIAN_POINT('Ctrl Pts',(-7.81060623090846,313.926074056311,4.47163317015251));
#12746=CARTESIAN_POINT('Ctrl Pts',(-9.00877672769904,314.063574056311,2.37878753818309));
#12747=CARTESIAN_POINT('Ctrl Pts',(-9.,314.201074056311,-0.0327551936970214));
#12748=CARTESIAN_POINT('Ctrl Pts',(-8.99122327230096,314.338574056311,-2.44429792557713));
#12749=CARTESIAN_POINT('Ctrl Pts',(-7.77785103721144,314.476074056311,-4.5283668298475));
#12750=CARTESIAN_POINT('Ctrl Pts',(-6.56447880212192,314.613574056311,-6.61243573411788));
#12751=CARTESIAN_POINT('Ctrl Pts',(-4.4716331701525,314.751074056311,-7.81060623090846));
#12752=CARTESIAN_POINT('Ctrl Pts',(-2.37878753818309,314.888574056311,-9.00877672769904));
#12753=CARTESIAN_POINT('Ctrl Pts',(0.0327551936970209,315.026074056311,
-9.));
#12754=CARTESIAN_POINT('Ctrl Pts',(2.44429792557713,315.163574056311,-8.99122327230096));
#12755=CARTESIAN_POINT('Ctrl Pts',(4.5283668298475,315.301074056311,-7.77785103721144));
#12756=CARTESIAN_POINT('Ctrl Pts',(6.61243573411788,315.438574056311,-6.56447880212192));
#12757=CARTESIAN_POINT('Ctrl Pts',(7.81060623090846,315.576074056311,-4.4716331701525));
#12758=CARTESIAN_POINT('Ctrl Pts',(9.00877672769904,315.713574056311,-2.37878753818309));
#12759=CARTESIAN_POINT('Ctrl Pts',(9.,315.851074056311,0.0327551936970203));
#12760=CARTESIAN_POINT('Ctrl Pts',(8.99122327230096,315.988574056311,2.44429792557712));
#12761=CARTESIAN_POINT('Ctrl Pts',(7.77785103721144,316.126074056311,4.5283668298475));
#12762=CARTESIAN_POINT('Ctrl Pts',(6.56447880212192,316.263574056311,6.61243573411788));
#12763=CARTESIAN_POINT('Ctrl Pts',(4.47163317015251,316.401074056311,7.81060623090846));
#12764=CARTESIAN_POINT('Ctrl Pts',(2.37878753818309,316.538574056311,9.00877672769904));
#12765=CARTESIAN_POINT('Ctrl Pts',(-0.0327551936970198,316.676074056311,
9.));
#12766=CARTESIAN_POINT('Ctrl Pts',(-2.44429792557712,316.813574056311,8.99122327230096));
#12767=CARTESIAN_POINT('Ctrl Pts',(-4.5283668298475,316.951074056311,7.77785103721144));
#12768=CARTESIAN_POINT('Ctrl Pts',(-6.61243573411788,317.088574056311,6.56447880212192));
#12769=CARTESIAN_POINT('Ctrl Pts',(-7.81060623090846,317.226074056311,4.47163317015251));
#12770=CARTESIAN_POINT('Ctrl Pts',(-9.00877672769904,317.363574056311,2.37878753818309));
#12771=CARTESIAN_POINT('Ctrl Pts',(-9.,317.501074056311,-0.0327551936970214));
#12772=CARTESIAN_POINT('Ctrl Pts',(-9.,285.498925943689,0.0327551936972079));
#12773=CARTESIAN_POINT('Ctrl Pts',(-9.0087767276991,285.636425943689,-2.3787875381829));
#12774=CARTESIAN_POINT('Ctrl Pts',(-7.81060623090856,285.773925943689,-4.47163317015234));
#12775=CARTESIAN_POINT('Ctrl Pts',(-6.61243573411802,285.911425943689,-6.56447880212179));
#12776=CARTESIAN_POINT('Ctrl Pts',(-4.52836682984766,286.048925943689,-7.77785103721135));
#12777=CARTESIAN_POINT('Ctrl Pts',(-2.44429792557731,286.186425943689,-8.99122327230091));
#12778=CARTESIAN_POINT('Ctrl Pts',(-0.0327551936972084,286.323925943689,
-9.));
#12779=CARTESIAN_POINT('Ctrl Pts',(2.3787875381829,286.461425943689,-9.0087767276991));
#12780=CARTESIAN_POINT('Ctrl Pts',(4.47163317015234,286.598925943689,-7.81060623090856));
#12781=CARTESIAN_POINT('Ctrl Pts',(6.56447880212178,286.736425943689,-6.61243573411802));
#12782=CARTESIAN_POINT('Ctrl Pts',(7.77785103721135,286.873925943689,-4.52836682984767));
#12783=CARTESIAN_POINT('Ctrl Pts',(8.99122327230091,287.011425943689,-2.44429792557732));
#12784=CARTESIAN_POINT('Ctrl Pts',(9.,287.148925943689,-0.032755193697209));
#12785=CARTESIAN_POINT('Ctrl Pts',(9.0087767276991,287.286425943689,2.37878753818289));
#12786=CARTESIAN_POINT('Ctrl Pts',(7.81060623090856,287.423925943689,4.47163317015234));
#12787=CARTESIAN_POINT('Ctrl Pts',(6.61243573411802,287.561425943689,6.56447880212178));
#12788=CARTESIAN_POINT('Ctrl Pts',(4.52836682984767,287.698925943689,7.77785103721135));
#12789=CARTESIAN_POINT('Ctrl Pts',(2.44429792557732,287.836425943689,8.99122327230091));
#12790=CARTESIAN_POINT('Ctrl Pts',(0.0327551936972095,287.973925943689,
9.));
#12791=CARTESIAN_POINT('Ctrl Pts',(-2.37878753818289,288.111425943689,9.0087767276991));
#12792=CARTESIAN_POINT('Ctrl Pts',(-4.47163317015233,288.248925943689,7.81060623090856));
#12793=CARTESIAN_POINT('Ctrl Pts',(-6.56447880212178,288.386425943689,6.61243573411802));
#12794=CARTESIAN_POINT('Ctrl Pts',(-7.77785103721135,288.523925943689,4.52836682984767));
#12795=CARTESIAN_POINT('Ctrl Pts',(-8.99122327230091,288.661425943689,2.44429792557732));
#12796=CARTESIAN_POINT('Ctrl Pts',(-9.,288.798925943689,0.0327551936972079));
#12797=CARTESIAN_POINT('Ctrl Pts',(-9.0087767276991,288.936425943689,-2.3787875381829));
#12798=CARTESIAN_POINT('Ctrl Pts',(-7.81060623090856,289.073925943689,-4.47163317015234));
#12799=CARTESIAN_POINT('Ctrl Pts',(-6.61243573411802,289.211425943689,-6.56447880212179));
#12800=CARTESIAN_POINT('Ctrl Pts',(-4.52836682984766,289.348925943689,-7.77785103721135));
#12801=CARTESIAN_POINT('Ctrl Pts',(-2.44429792557731,289.486425943689,-8.99122327230091));
#12802=CARTESIAN_POINT('Ctrl Pts',(-0.0327551936972084,289.623925943689,
-9.));
#12803=CARTESIAN_POINT('Ctrl Pts',(2.3787875381829,289.761425943689,-9.0087767276991));
#12804=CARTESIAN_POINT('Ctrl Pts',(4.47163317015234,289.898925943689,-7.81060623090856));
#12805=CARTESIAN_POINT('Ctrl Pts',(6.56447880212178,290.036425943689,-6.61243573411802));
#12806=CARTESIAN_POINT('Ctrl Pts',(7.77785103721135,290.173925943689,-4.52836682984767));
#12807=CARTESIAN_POINT('Ctrl Pts',(8.99122327230091,290.311425943689,-2.44429792557732));
#12808=CARTESIAN_POINT('Ctrl Pts',(9.,290.448925943689,-0.032755193697209));
#12809=CARTESIAN_POINT('Ctrl Pts',(9.0087767276991,290.586425943689,2.37878753818289));
#12810=CARTESIAN_POINT('Ctrl Pts',(7.81060623090856,290.723925943689,4.47163317015234));
#12811=CARTESIAN_POINT('Ctrl Pts',(6.61243573411802,290.861425943689,6.56447880212178));
#12812=CARTESIAN_POINT('Ctrl Pts',(4.52836682984767,290.998925943689,7.77785103721135));
#12813=CARTESIAN_POINT('Ctrl Pts',(2.44429792557732,291.136425943689,8.99122327230091));
#12814=CARTESIAN_POINT('Ctrl Pts',(0.0327551936972095,291.273925943689,
9.));
#12815=CARTESIAN_POINT('Ctrl Pts',(-2.37878753818289,291.411425943689,9.0087767276991));
#12816=CARTESIAN_POINT('Ctrl Pts',(-4.47163317015233,291.548925943689,7.81060623090856));
#12817=CARTESIAN_POINT('Ctrl Pts',(-6.56447880212178,291.686425943689,6.61243573411802));
#12818=CARTESIAN_POINT('Ctrl Pts',(-7.77785103721135,291.823925943689,4.52836682984767));
#12819=CARTESIAN_POINT('Ctrl Pts',(-8.99122327230091,291.961425943689,2.44429792557732));
#12820=CARTESIAN_POINT('Ctrl Pts',(-9.,292.098925943689,0.0327551936972079));
#12821=CARTESIAN_POINT('Ctrl Pts',(-9.0087767276991,292.236425943689,-2.3787875381829));
#12822=CARTESIAN_POINT('Ctrl Pts',(-7.81060623090856,292.373925943689,-4.47163317015234));
#12823=CARTESIAN_POINT('Ctrl Pts',(-6.61243573411802,292.511425943689,-6.56447880212179));
#12824=CARTESIAN_POINT('Ctrl Pts',(-4.52836682984766,292.648925943689,-7.77785103721135));
#12825=CARTESIAN_POINT('Ctrl Pts',(-2.44429792557731,292.786425943689,-8.99122327230091));
#12826=CARTESIAN_POINT('Ctrl Pts',(-0.0327551936972084,292.923925943689,
-9.));
#12827=CARTESIAN_POINT('Ctrl Pts',(2.3787875381829,293.061425943689,-9.0087767276991));
#12828=CARTESIAN_POINT('Ctrl Pts',(4.47163317015234,293.198925943689,-7.81060623090856));
#12829=CARTESIAN_POINT('Ctrl Pts',(6.56447880212178,293.336425943689,-6.61243573411802));
#12830=CARTESIAN_POINT('Ctrl Pts',(7.77785103721135,293.473925943689,-4.52836682984767));
#12831=CARTESIAN_POINT('Ctrl Pts',(8.99122327230091,293.611425943689,-2.44429792557732));
#12832=CARTESIAN_POINT('Ctrl Pts',(9.,293.748925943689,-0.032755193697209));
#12833=CARTESIAN_POINT('Ctrl Pts',(9.0087767276991,293.886425943689,2.37878753818289));
#12834=CARTESIAN_POINT('Ctrl Pts',(7.81060623090856,294.023925943689,4.47163317015234));
#12835=CARTESIAN_POINT('Ctrl Pts',(6.61243573411802,294.161425943689,6.56447880212178));
#12836=CARTESIAN_POINT('Ctrl Pts',(4.52836682984767,294.298925943689,7.77785103721135));
#12837=CARTESIAN_POINT('Ctrl Pts',(2.44429792557732,294.436425943689,8.99122327230091));
#12838=CARTESIAN_POINT('Ctrl Pts',(0.0327551936972095,294.573925943689,
9.));
#12839=CARTESIAN_POINT('Ctrl Pts',(-2.37878753818289,294.711425943689,9.0087767276991));
#12840=CARTESIAN_POINT('Ctrl Pts',(-4.47163317015233,294.848925943689,7.81060623090856));
#12841=CARTESIAN_POINT('Ctrl Pts',(-6.56447880212178,294.986425943689,6.61243573411802));
#12842=CARTESIAN_POINT('Ctrl Pts',(-7.77785103721135,295.123925943689,4.52836682984767));
#12843=CARTESIAN_POINT('Ctrl Pts',(-8.99122327230091,295.261425943689,2.44429792557732));
#12844=CARTESIAN_POINT('Ctrl Pts',(-9.,295.398925943689,0.0327551936972079));
#12845=CARTESIAN_POINT('Ctrl Pts',(-9.0087767276991,295.536425943689,-2.3787875381829));
#12846=CARTESIAN_POINT('Ctrl Pts',(-7.81060623090856,295.673925943689,-4.47163317015234));
#12847=CARTESIAN_POINT('Ctrl Pts',(-6.61243573411802,295.811425943689,-6.56447880212179));
#12848=CARTESIAN_POINT('Ctrl Pts',(-4.52836682984766,295.948925943689,-7.77785103721135));
#12849=CARTESIAN_POINT('Ctrl Pts',(-2.44429792557731,296.086425943689,-8.99122327230091));
#12850=CARTESIAN_POINT('Ctrl Pts',(-0.0327551936972084,296.223925943689,
-9.));
#12851=CARTESIAN_POINT('Ctrl Pts',(2.3787875381829,296.361425943689,-9.0087767276991));
#12852=CARTESIAN_POINT('Ctrl Pts',(4.47163317015234,296.498925943689,-7.81060623090856));
#12853=CARTESIAN_POINT('Ctrl Pts',(6.56447880212178,296.636425943689,-6.61243573411802));
#12854=CARTESIAN_POINT('Ctrl Pts',(7.77785103721135,296.773925943689,-4.52836682984767));
#12855=CARTESIAN_POINT('Ctrl Pts',(8.99122327230091,296.911425943689,-2.44429792557732));
#12856=CARTESIAN_POINT('Ctrl Pts',(9.,297.048925943689,-0.032755193697209));
#12857=CARTESIAN_POINT('Ctrl Pts',(9.0087767276991,297.186425943689,2.37878753818289));
#12858=CARTESIAN_POINT('Ctrl Pts',(7.81060623090856,297.323925943689,4.47163317015234));
#12859=CARTESIAN_POINT('Ctrl Pts',(6.61243573411802,297.461425943689,6.56447880212178));
#12860=CARTESIAN_POINT('Ctrl Pts',(4.52836682984767,297.598925943689,7.77785103721135));
#12861=CARTESIAN_POINT('Ctrl Pts',(2.44429792557732,297.736425943689,8.99122327230091));
#12862=CARTESIAN_POINT('Ctrl Pts',(0.0327551936972095,297.873925943689,
9.));
#12863=CARTESIAN_POINT('Ctrl Pts',(-2.37878753818289,298.011425943689,9.0087767276991));
#12864=CARTESIAN_POINT('Ctrl Pts',(-4.47163317015233,298.148925943689,7.81060623090856));
#12865=CARTESIAN_POINT('Ctrl Pts',(-6.56447880212178,298.286425943689,6.61243573411802));
#12866=CARTESIAN_POINT('Ctrl Pts',(-7.77785103721135,298.423925943689,4.52836682984767));
#12867=CARTESIAN_POINT('Ctrl Pts',(-8.99122327230091,298.561425943689,2.44429792557732));
#12868=CARTESIAN_POINT('Ctrl Pts',(-9.,298.698925943689,0.0327551936972079));
#12869=CARTESIAN_POINT('Ctrl Pts',(-9.0087767276991,298.836425943689,-2.3787875381829));
#12870=CARTESIAN_POINT('Ctrl Pts',(-7.81060623090856,298.973925943689,-4.47163317015234));
#12871=CARTESIAN_POINT('Ctrl Pts',(-6.61243573411802,299.111425943689,-6.56447880212179));
#12872=CARTESIAN_POINT('Ctrl Pts',(-4.52836682984766,299.248925943689,-7.77785103721135));
#12873=CARTESIAN_POINT('Ctrl Pts',(-2.44429792557731,299.386425943689,-8.99122327230091));
#12874=CARTESIAN_POINT('Ctrl Pts',(-0.0327551936972084,299.523925943689,
-9.));
#12875=CARTESIAN_POINT('Ctrl Pts',(2.3787875381829,299.661425943689,-9.0087767276991));
#12876=CARTESIAN_POINT('Ctrl Pts',(4.47163317015234,299.798925943689,-7.81060623090856));
#12877=CARTESIAN_POINT('Ctrl Pts',(6.56447880212178,299.936425943689,-6.61243573411802));
#12878=CARTESIAN_POINT('Ctrl Pts',(7.77785103721135,300.073925943689,-4.52836682984767));
#12879=CARTESIAN_POINT('Ctrl Pts',(8.99122327230091,300.211425943689,-2.44429792557732));
#12880=CARTESIAN_POINT('Ctrl Pts',(9.,300.348925943689,-0.032755193697209));
#12881=CARTESIAN_POINT('Ctrl Pts',(9.0087767276991,300.486425943689,2.37878753818289));
#12882=CARTESIAN_POINT('Ctrl Pts',(7.81060623090856,300.623925943689,4.47163317015234));
#12883=CARTESIAN_POINT('Ctrl Pts',(6.61243573411802,300.761425943689,6.56447880212178));
#12884=CARTESIAN_POINT('Ctrl Pts',(4.52836682984767,300.898925943689,7.77785103721135));
#12885=CARTESIAN_POINT('Ctrl Pts',(2.44429792557732,301.036425943689,8.99122327230091));
#12886=CARTESIAN_POINT('Ctrl Pts',(0.0327551936972095,301.173925943689,
9.));
#12887=CARTESIAN_POINT('Ctrl Pts',(-2.37878753818289,301.311425943689,9.0087767276991));
#12888=CARTESIAN_POINT('Ctrl Pts',(-4.47163317015233,301.448925943689,7.81060623090856));
#12889=CARTESIAN_POINT('Ctrl Pts',(-6.56447880212178,301.586425943689,6.61243573411802));
#12890=CARTESIAN_POINT('Ctrl Pts',(-7.77785103721135,301.723925943689,4.52836682984767));
#12891=CARTESIAN_POINT('Ctrl Pts',(-8.99122327230091,301.861425943689,2.44429792557732));
#12892=CARTESIAN_POINT('Ctrl Pts',(-9.,301.998925943689,0.0327551936972079));
#12893=CARTESIAN_POINT('Ctrl Pts',(-9.0087767276991,302.136425943689,-2.3787875381829));
#12894=CARTESIAN_POINT('Ctrl Pts',(-7.81060623090856,302.273925943689,-4.47163317015234));
#12895=CARTESIAN_POINT('Ctrl Pts',(-6.61243573411802,302.411425943689,-6.56447880212179));
#12896=CARTESIAN_POINT('Ctrl Pts',(-4.52836682984766,302.548925943689,-7.77785103721135));
#12897=CARTESIAN_POINT('Ctrl Pts',(-2.44429792557731,302.686425943689,-8.99122327230091));
#12898=CARTESIAN_POINT('Ctrl Pts',(-0.0327551936972084,302.823925943689,
-9.));
#12899=CARTESIAN_POINT('Ctrl Pts',(2.3787875381829,302.961425943689,-9.0087767276991));
#12900=CARTESIAN_POINT('Ctrl Pts',(4.47163317015234,303.098925943689,-7.81060623090856));
#12901=CARTESIAN_POINT('Ctrl Pts',(6.56447880212178,303.236425943689,-6.61243573411802));
#12902=CARTESIAN_POINT('Ctrl Pts',(7.77785103721135,303.373925943689,-4.52836682984767));
#12903=CARTESIAN_POINT('Ctrl Pts',(8.99122327230091,303.511425943689,-2.44429792557732));
#12904=CARTESIAN_POINT('Ctrl Pts',(9.,303.648925943689,-0.032755193697209));
#12905=CARTESIAN_POINT('Ctrl Pts',(9.0087767276991,303.786425943689,2.37878753818289));
#12906=CARTESIAN_POINT('Ctrl Pts',(7.81060623090856,303.923925943689,4.47163317015234));
#12907=CARTESIAN_POINT('Ctrl Pts',(6.61243573411802,304.061425943689,6.56447880212178));
#12908=CARTESIAN_POINT('Ctrl Pts',(4.52836682984767,304.198925943689,7.77785103721135));
#12909=CARTESIAN_POINT('Ctrl Pts',(2.44429792557732,304.336425943689,8.99122327230091));
#12910=CARTESIAN_POINT('Ctrl Pts',(0.0327551936972095,304.473925943689,
9.));
#12911=CARTESIAN_POINT('Ctrl Pts',(-2.37878753818289,304.611425943689,9.0087767276991));
#12912=CARTESIAN_POINT('Ctrl Pts',(-4.47163317015233,304.748925943689,7.81060623090856));
#12913=CARTESIAN_POINT('Ctrl Pts',(-6.56447880212178,304.886425943689,6.61243573411802));
#12914=CARTESIAN_POINT('Ctrl Pts',(-7.77785103721135,305.023925943689,4.52836682984767));
#12915=CARTESIAN_POINT('Ctrl Pts',(-8.99122327230091,305.161425943689,2.44429792557732));
#12916=CARTESIAN_POINT('Ctrl Pts',(-9.,305.298925943689,0.0327551936972079));
#12917=CARTESIAN_POINT('Ctrl Pts',(-9.0087767276991,305.436425943689,-2.3787875381829));
#12918=CARTESIAN_POINT('Ctrl Pts',(-7.81060623090856,305.573925943689,-4.47163317015234));
#12919=CARTESIAN_POINT('Ctrl Pts',(-6.61243573411802,305.711425943689,-6.56447880212179));
#12920=CARTESIAN_POINT('Ctrl Pts',(-4.52836682984766,305.848925943689,-7.77785103721135));
#12921=CARTESIAN_POINT('Ctrl Pts',(-2.44429792557731,305.986425943689,-8.99122327230091));
#12922=CARTESIAN_POINT('Ctrl Pts',(-0.0327551936972084,306.123925943689,
-9.));
#12923=CARTESIAN_POINT('Ctrl Pts',(2.3787875381829,306.261425943689,-9.0087767276991));
#12924=CARTESIAN_POINT('Ctrl Pts',(4.47163317015234,306.398925943689,-7.81060623090856));
#12925=CARTESIAN_POINT('Ctrl Pts',(6.56447880212178,306.536425943689,-6.61243573411802));
#12926=CARTESIAN_POINT('Ctrl Pts',(7.77785103721135,306.673925943689,-4.52836682984767));
#12927=CARTESIAN_POINT('Ctrl Pts',(8.99122327230091,306.811425943689,-2.44429792557732));
#12928=CARTESIAN_POINT('Ctrl Pts',(9.,306.948925943689,-0.032755193697209));
#12929=CARTESIAN_POINT('Ctrl Pts',(9.0087767276991,307.086425943689,2.37878753818289));
#12930=CARTESIAN_POINT('Ctrl Pts',(7.81060623090856,307.223925943689,4.47163317015234));
#12931=CARTESIAN_POINT('Ctrl Pts',(6.61243573411802,307.361425943689,6.56447880212178));
#12932=CARTESIAN_POINT('Ctrl Pts',(4.52836682984767,307.498925943689,7.77785103721135));
#12933=CARTESIAN_POINT('Ctrl Pts',(2.44429792557732,307.636425943689,8.99122327230091));
#12934=CARTESIAN_POINT('Ctrl Pts',(0.0327551936972095,307.773925943689,
9.));
#12935=CARTESIAN_POINT('Ctrl Pts',(-2.37878753818289,307.911425943689,9.0087767276991));
#12936=CARTESIAN_POINT('Ctrl Pts',(-4.47163317015233,308.048925943689,7.81060623090856));
#12937=CARTESIAN_POINT('Ctrl Pts',(-6.56447880212178,308.186425943689,6.61243573411802));
#12938=CARTESIAN_POINT('Ctrl Pts',(-7.77785103721135,308.323925943689,4.52836682984767));
#12939=CARTESIAN_POINT('Ctrl Pts',(-8.99122327230091,308.461425943689,2.44429792557732));
#12940=CARTESIAN_POINT('Ctrl Pts',(-9.,308.598925943689,0.0327551936972079));
#12941=CARTESIAN_POINT('Ctrl Pts',(-9.0087767276991,308.736425943689,-2.3787875381829));
#12942=CARTESIAN_POINT('Ctrl Pts',(-7.81060623090856,308.873925943689,-4.47163317015234));
#12943=CARTESIAN_POINT('Ctrl Pts',(-6.61243573411802,309.011425943689,-6.56447880212179));
#12944=CARTESIAN_POINT('Ctrl Pts',(-4.52836682984766,309.148925943689,-7.77785103721135));
#12945=CARTESIAN_POINT('Ctrl Pts',(-2.44429792557731,309.286425943689,-8.99122327230091));
#12946=CARTESIAN_POINT('Ctrl Pts',(-0.0327551936972084,309.423925943689,
-9.));
#12947=CARTESIAN_POINT('Ctrl Pts',(2.3787875381829,309.561425943689,-9.0087767276991));
#12948=CARTESIAN_POINT('Ctrl Pts',(4.47163317015234,309.698925943689,-7.81060623090856));
#12949=CARTESIAN_POINT('Ctrl Pts',(6.56447880212178,309.836425943689,-6.61243573411802));
#12950=CARTESIAN_POINT('Ctrl Pts',(7.77785103721135,309.973925943689,-4.52836682984767));
#12951=CARTESIAN_POINT('Ctrl Pts',(8.99122327230091,310.111425943689,-2.44429792557732));
#12952=CARTESIAN_POINT('Ctrl Pts',(9.,310.248925943689,-0.032755193697209));
#12953=CARTESIAN_POINT('Ctrl Pts',(9.0087767276991,310.386425943689,2.37878753818289));
#12954=CARTESIAN_POINT('Ctrl Pts',(7.81060623090856,310.523925943689,4.47163317015234));
#12955=CARTESIAN_POINT('Ctrl Pts',(6.61243573411802,310.661425943689,6.56447880212178));
#12956=CARTESIAN_POINT('Ctrl Pts',(4.52836682984767,310.798925943689,7.77785103721135));
#12957=CARTESIAN_POINT('Ctrl Pts',(2.44429792557732,310.936425943689,8.99122327230091));
#12958=CARTESIAN_POINT('Ctrl Pts',(0.0327551936972095,311.073925943689,
9.));
#12959=CARTESIAN_POINT('Ctrl Pts',(-2.37878753818289,311.211425943689,9.0087767276991));
#12960=CARTESIAN_POINT('Ctrl Pts',(-4.47163317015233,311.348925943689,7.81060623090856));
#12961=CARTESIAN_POINT('Ctrl Pts',(-6.56447880212178,311.486425943689,6.61243573411802));
#12962=CARTESIAN_POINT('Ctrl Pts',(-7.77785103721135,311.623925943689,4.52836682984767));
#12963=CARTESIAN_POINT('Ctrl Pts',(-8.99122327230091,311.761425943689,2.44429792557732));
#12964=CARTESIAN_POINT('Ctrl Pts',(-9.,311.898925943689,0.0327551936972079));
#12965=CARTESIAN_POINT('Ctrl Pts',(-9.0087767276991,312.036425943689,-2.3787875381829));
#12966=CARTESIAN_POINT('Ctrl Pts',(-7.81060623090856,312.173925943689,-4.47163317015234));
#12967=CARTESIAN_POINT('Ctrl Pts',(-6.61243573411802,312.311425943689,-6.56447880212179));
#12968=CARTESIAN_POINT('Ctrl Pts',(-4.52836682984766,312.448925943689,-7.77785103721135));
#12969=CARTESIAN_POINT('Ctrl Pts',(-2.44429792557731,312.586425943689,-8.99122327230091));
#12970=CARTESIAN_POINT('Ctrl Pts',(-0.0327551936972084,312.723925943689,
-9.));
#12971=CARTESIAN_POINT('Ctrl Pts',(2.3787875381829,312.861425943689,-9.0087767276991));
#12972=CARTESIAN_POINT('Ctrl Pts',(4.47163317015234,312.998925943689,-7.81060623090856));
#12973=CARTESIAN_POINT('Ctrl Pts',(6.56447880212178,313.136425943689,-6.61243573411802));
#12974=CARTESIAN_POINT('Ctrl Pts',(7.77785103721135,313.273925943689,-4.52836682984767));
#12975=CARTESIAN_POINT('Ctrl Pts',(8.99122327230091,313.411425943689,-2.44429792557732));
#12976=CARTESIAN_POINT('Ctrl Pts',(9.,313.548925943689,-0.032755193697209));
#12977=CARTESIAN_POINT('Ctrl Pts',(9.0087767276991,313.686425943689,2.37878753818289));
#12978=CARTESIAN_POINT('Ctrl Pts',(7.81060623090856,313.823925943689,4.47163317015234));
#12979=CARTESIAN_POINT('Ctrl Pts',(6.61243573411802,313.961425943689,6.56447880212178));
#12980=CARTESIAN_POINT('Ctrl Pts',(4.52836682984767,314.098925943689,7.77785103721135));
#12981=CARTESIAN_POINT('Ctrl Pts',(2.44429792557732,314.236425943689,8.99122327230091));
#12982=CARTESIAN_POINT('Ctrl Pts',(0.0327551936972095,314.373925943689,
9.));
#12983=CARTESIAN_POINT('Ctrl Pts',(-2.37878753818289,314.511425943689,9.0087767276991));
#12984=CARTESIAN_POINT('Ctrl Pts',(-4.47163317015233,314.648925943689,7.81060623090856));
#12985=CARTESIAN_POINT('Ctrl Pts',(-6.56447880212178,314.786425943689,6.61243573411802));
#12986=CARTESIAN_POINT('Ctrl Pts',(-7.77785103721135,314.923925943689,4.52836682984767));
#12987=CARTESIAN_POINT('Ctrl Pts',(-8.99122327230091,315.061425943689,2.44429792557732));
#12988=CARTESIAN_POINT('Ctrl Pts',(-9.,315.198925943689,0.0327551936972079));
#12989=CARTESIAN_POINT('Ctrl Pts',(-9.0087767276991,315.336425943689,-2.3787875381829));
#12990=CARTESIAN_POINT('Ctrl Pts',(-7.81060623090856,315.473925943689,-4.47163317015234));
#12991=CARTESIAN_POINT('Ctrl Pts',(-6.61243573411802,315.611425943689,-6.56447880212179));
#12992=CARTESIAN_POINT('Ctrl Pts',(-4.52836682984766,315.748925943689,-7.77785103721135));
#12993=CARTESIAN_POINT('Ctrl Pts',(-2.44429792557731,315.886425943689,-8.99122327230091));
#12994=CARTESIAN_POINT('Ctrl Pts',(-0.0327551936972084,316.023925943689,
-9.));
#12995=CARTESIAN_POINT('Ctrl Pts',(2.3787875381829,316.161425943689,-9.0087767276991));
#12996=CARTESIAN_POINT('Ctrl Pts',(4.47163317015234,316.298925943689,-7.81060623090856));
#12997=CARTESIAN_POINT('Ctrl Pts',(6.56447880212178,316.436425943689,-6.61243573411802));
#12998=CARTESIAN_POINT('Ctrl Pts',(7.77785103721135,316.573925943689,-4.52836682984767));
#12999=CARTESIAN_POINT('Ctrl Pts',(8.99122327230091,316.711425943689,-2.44429792557732));
#13000=CARTESIAN_POINT('Ctrl Pts',(9.,316.848925943689,-0.032755193697209));
#13001=CARTESIAN_POINT('Ctrl Pts',(9.0087767276991,316.986425943689,2.37878753818289));
#13002=CARTESIAN_POINT('Ctrl Pts',(7.81060623090856,317.123925943689,4.47163317015234));
#13003=CARTESIAN_POINT('Ctrl Pts',(6.61243573411802,317.261425943689,6.56447880212178));
#13004=CARTESIAN_POINT('Ctrl Pts',(4.52836682984767,317.398925943689,7.77785103721135));
#13005=CARTESIAN_POINT('Ctrl Pts',(2.44429792557732,317.536425943689,8.99122327230091));
#13006=CARTESIAN_POINT('Ctrl Pts',(0.0327551936972095,317.673925943689,
9.));
#13007=CARTESIAN_POINT('Ctrl Pts',(-2.37878753818289,317.811425943689,9.0087767276991));
#13008=CARTESIAN_POINT('Ctrl Pts',(-4.47163317015233,317.948925943689,7.81060623090856));
#13009=CARTESIAN_POINT('Ctrl Pts',(-6.56447880212178,318.086425943689,6.61243573411802));
#13010=CARTESIAN_POINT('Ctrl Pts',(-7.77785103721135,318.223925943689,4.52836682984767));
#13011=CARTESIAN_POINT('Ctrl Pts',(-8.99122327230091,318.361425943689,2.44429792557732));
#13012=CARTESIAN_POINT('Ctrl Pts',(-9.,318.498925943689,0.0327551936972079));
#13013=CARTESIAN_POINT('Ctrl Pts',(-8.,285.498925943689,0.0327551936971979));
#13014=CARTESIAN_POINT('Ctrl Pts',(-8.00877672769909,285.636425943689,-2.11083834575178));
#13015=CARTESIAN_POINT('Ctrl Pts',(-6.94458082712411,285.773925943689,-3.97163317015235));
#13016=CARTESIAN_POINT('Ctrl Pts',(-5.88038492654913,285.911425943689,-5.83242799455291));
#13017=CARTESIAN_POINT('Ctrl Pts',(-4.02836682984766,286.048925943689,-6.91182563342691));
#13018=CARTESIAN_POINT('Ctrl Pts',(-2.17634873314618,286.186425943689,-7.99122327230091));
#13019=CARTESIAN_POINT('Ctrl Pts',(-0.0327551936971984,286.323925943689,
-8.));
#13020=CARTESIAN_POINT('Ctrl Pts',(2.11083834575178,286.461425943689,-8.00877672769909));
#13021=CARTESIAN_POINT('Ctrl Pts',(3.97163317015235,286.598925943689,-6.94458082712411));
#13022=CARTESIAN_POINT('Ctrl Pts',(5.83242799455291,286.736425943689,-5.88038492654913));
#13023=CARTESIAN_POINT('Ctrl Pts',(6.91182563342691,286.873925943689,-4.02836682984766));
#13024=CARTESIAN_POINT('Ctrl Pts',(7.99122327230091,287.011425943689,-2.17634873314618));
#13025=CARTESIAN_POINT('Ctrl Pts',(8.,287.148925943689,-0.0327551936971989));
#13026=CARTESIAN_POINT('Ctrl Pts',(8.00877672769909,287.286425943689,2.11083834575178));
#13027=CARTESIAN_POINT('Ctrl Pts',(6.94458082712411,287.423925943689,3.97163317015235));
#13028=CARTESIAN_POINT('Ctrl Pts',(5.88038492654913,287.561425943689,5.83242799455291));
#13029=CARTESIAN_POINT('Ctrl Pts',(4.02836682984766,287.698925943689,6.91182563342691));
#13030=CARTESIAN_POINT('Ctrl Pts',(2.17634873314619,287.836425943689,7.99122327230091));
#13031=CARTESIAN_POINT('Ctrl Pts',(0.0327551936971994,287.973925943689,
8.));
#13032=CARTESIAN_POINT('Ctrl Pts',(-2.11083834575178,288.111425943689,8.00877672769909));
#13033=CARTESIAN_POINT('Ctrl Pts',(-3.97163317015234,288.248925943689,6.94458082712412));
#13034=CARTESIAN_POINT('Ctrl Pts',(-5.83242799455291,288.386425943689,5.88038492654913));
#13035=CARTESIAN_POINT('Ctrl Pts',(-6.91182563342691,288.523925943689,4.02836682984766));
#13036=CARTESIAN_POINT('Ctrl Pts',(-7.99122327230091,288.661425943689,2.17634873314619));
#13037=CARTESIAN_POINT('Ctrl Pts',(-8.,288.798925943689,0.0327551936971979));
#13038=CARTESIAN_POINT('Ctrl Pts',(-8.00877672769909,288.936425943689,-2.11083834575178));
#13039=CARTESIAN_POINT('Ctrl Pts',(-6.94458082712411,289.073925943689,-3.97163317015235));
#13040=CARTESIAN_POINT('Ctrl Pts',(-5.88038492654913,289.211425943689,-5.83242799455291));
#13041=CARTESIAN_POINT('Ctrl Pts',(-4.02836682984766,289.348925943689,-6.91182563342691));
#13042=CARTESIAN_POINT('Ctrl Pts',(-2.17634873314618,289.486425943689,-7.99122327230091));
#13043=CARTESIAN_POINT('Ctrl Pts',(-0.0327551936971984,289.623925943689,
-8.));
#13044=CARTESIAN_POINT('Ctrl Pts',(2.11083834575178,289.761425943689,-8.00877672769909));
#13045=CARTESIAN_POINT('Ctrl Pts',(3.97163317015235,289.898925943689,-6.94458082712411));
#13046=CARTESIAN_POINT('Ctrl Pts',(5.83242799455291,290.036425943689,-5.88038492654913));
#13047=CARTESIAN_POINT('Ctrl Pts',(6.91182563342691,290.173925943689,-4.02836682984766));
#13048=CARTESIAN_POINT('Ctrl Pts',(7.99122327230091,290.311425943689,-2.17634873314618));
#13049=CARTESIAN_POINT('Ctrl Pts',(8.,290.448925943689,-0.0327551936971989));
#13050=CARTESIAN_POINT('Ctrl Pts',(8.00877672769909,290.586425943689,2.11083834575178));
#13051=CARTESIAN_POINT('Ctrl Pts',(6.94458082712411,290.723925943689,3.97163317015235));
#13052=CARTESIAN_POINT('Ctrl Pts',(5.88038492654913,290.861425943689,5.83242799455291));
#13053=CARTESIAN_POINT('Ctrl Pts',(4.02836682984766,290.998925943689,6.91182563342691));
#13054=CARTESIAN_POINT('Ctrl Pts',(2.17634873314619,291.136425943689,7.99122327230091));
#13055=CARTESIAN_POINT('Ctrl Pts',(0.0327551936971994,291.273925943689,
8.));
#13056=CARTESIAN_POINT('Ctrl Pts',(-2.11083834575178,291.411425943689,8.00877672769909));
#13057=CARTESIAN_POINT('Ctrl Pts',(-3.97163317015234,291.548925943689,6.94458082712412));
#13058=CARTESIAN_POINT('Ctrl Pts',(-5.83242799455291,291.686425943689,5.88038492654913));
#13059=CARTESIAN_POINT('Ctrl Pts',(-6.91182563342691,291.823925943689,4.02836682984766));
#13060=CARTESIAN_POINT('Ctrl Pts',(-7.99122327230091,291.961425943689,2.17634873314619));
#13061=CARTESIAN_POINT('Ctrl Pts',(-8.,292.098925943689,0.0327551936971979));
#13062=CARTESIAN_POINT('Ctrl Pts',(-8.00877672769909,292.236425943689,-2.11083834575178));
#13063=CARTESIAN_POINT('Ctrl Pts',(-6.94458082712411,292.373925943689,-3.97163317015235));
#13064=CARTESIAN_POINT('Ctrl Pts',(-5.88038492654913,292.511425943689,-5.83242799455291));
#13065=CARTESIAN_POINT('Ctrl Pts',(-4.02836682984766,292.648925943689,-6.91182563342691));
#13066=CARTESIAN_POINT('Ctrl Pts',(-2.17634873314618,292.786425943689,-7.99122327230091));
#13067=CARTESIAN_POINT('Ctrl Pts',(-0.0327551936971984,292.923925943689,
-8.));
#13068=CARTESIAN_POINT('Ctrl Pts',(2.11083834575178,293.061425943689,-8.00877672769909));
#13069=CARTESIAN_POINT('Ctrl Pts',(3.97163317015235,293.198925943689,-6.94458082712411));
#13070=CARTESIAN_POINT('Ctrl Pts',(5.83242799455291,293.336425943689,-5.88038492654913));
#13071=CARTESIAN_POINT('Ctrl Pts',(6.91182563342691,293.473925943689,-4.02836682984766));
#13072=CARTESIAN_POINT('Ctrl Pts',(7.99122327230091,293.611425943689,-2.17634873314618));
#13073=CARTESIAN_POINT('Ctrl Pts',(8.,293.748925943689,-0.0327551936971989));
#13074=CARTESIAN_POINT('Ctrl Pts',(8.00877672769909,293.886425943689,2.11083834575178));
#13075=CARTESIAN_POINT('Ctrl Pts',(6.94458082712411,294.023925943689,3.97163317015235));
#13076=CARTESIAN_POINT('Ctrl Pts',(5.88038492654913,294.161425943689,5.83242799455291));
#13077=CARTESIAN_POINT('Ctrl Pts',(4.02836682984766,294.298925943689,6.91182563342691));
#13078=CARTESIAN_POINT('Ctrl Pts',(2.17634873314619,294.436425943689,7.99122327230091));
#13079=CARTESIAN_POINT('Ctrl Pts',(0.0327551936971994,294.573925943689,
8.));
#13080=CARTESIAN_POINT('Ctrl Pts',(-2.11083834575178,294.711425943689,8.00877672769909));
#13081=CARTESIAN_POINT('Ctrl Pts',(-3.97163317015234,294.848925943689,6.94458082712412));
#13082=CARTESIAN_POINT('Ctrl Pts',(-5.83242799455291,294.986425943689,5.88038492654913));
#13083=CARTESIAN_POINT('Ctrl Pts',(-6.91182563342691,295.123925943689,4.02836682984766));
#13084=CARTESIAN_POINT('Ctrl Pts',(-7.99122327230091,295.261425943689,2.17634873314619));
#13085=CARTESIAN_POINT('Ctrl Pts',(-8.,295.398925943689,0.0327551936971979));
#13086=CARTESIAN_POINT('Ctrl Pts',(-8.00877672769909,295.536425943689,-2.11083834575178));
#13087=CARTESIAN_POINT('Ctrl Pts',(-6.94458082712411,295.673925943689,-3.97163317015235));
#13088=CARTESIAN_POINT('Ctrl Pts',(-5.88038492654913,295.811425943689,-5.83242799455291));
#13089=CARTESIAN_POINT('Ctrl Pts',(-4.02836682984766,295.948925943689,-6.91182563342691));
#13090=CARTESIAN_POINT('Ctrl Pts',(-2.17634873314618,296.086425943689,-7.99122327230091));
#13091=CARTESIAN_POINT('Ctrl Pts',(-0.0327551936971984,296.223925943689,
-8.));
#13092=CARTESIAN_POINT('Ctrl Pts',(2.11083834575178,296.361425943689,-8.00877672769909));
#13093=CARTESIAN_POINT('Ctrl Pts',(3.97163317015235,296.498925943689,-6.94458082712411));
#13094=CARTESIAN_POINT('Ctrl Pts',(5.83242799455291,296.636425943689,-5.88038492654913));
#13095=CARTESIAN_POINT('Ctrl Pts',(6.91182563342691,296.773925943689,-4.02836682984766));
#13096=CARTESIAN_POINT('Ctrl Pts',(7.99122327230091,296.911425943689,-2.17634873314618));
#13097=CARTESIAN_POINT('Ctrl Pts',(8.,297.048925943689,-0.0327551936971989));
#13098=CARTESIAN_POINT('Ctrl Pts',(8.00877672769909,297.186425943689,2.11083834575178));
#13099=CARTESIAN_POINT('Ctrl Pts',(6.94458082712411,297.323925943689,3.97163317015235));
#13100=CARTESIAN_POINT('Ctrl Pts',(5.88038492654913,297.461425943689,5.83242799455291));
#13101=CARTESIAN_POINT('Ctrl Pts',(4.02836682984766,297.598925943689,6.91182563342691));
#13102=CARTESIAN_POINT('Ctrl Pts',(2.17634873314619,297.736425943689,7.99122327230091));
#13103=CARTESIAN_POINT('Ctrl Pts',(0.0327551936971994,297.873925943689,
8.));
#13104=CARTESIAN_POINT('Ctrl Pts',(-2.11083834575178,298.011425943689,8.00877672769909));
#13105=CARTESIAN_POINT('Ctrl Pts',(-3.97163317015234,298.148925943689,6.94458082712412));
#13106=CARTESIAN_POINT('Ctrl Pts',(-5.83242799455291,298.286425943689,5.88038492654913));
#13107=CARTESIAN_POINT('Ctrl Pts',(-6.91182563342691,298.423925943689,4.02836682984766));
#13108=CARTESIAN_POINT('Ctrl Pts',(-7.99122327230091,298.561425943689,2.17634873314619));
#13109=CARTESIAN_POINT('Ctrl Pts',(-8.,298.698925943689,0.0327551936971979));
#13110=CARTESIAN_POINT('Ctrl Pts',(-8.00877672769909,298.836425943689,-2.11083834575178));
#13111=CARTESIAN_POINT('Ctrl Pts',(-6.94458082712411,298.973925943689,-3.97163317015235));
#13112=CARTESIAN_POINT('Ctrl Pts',(-5.88038492654913,299.111425943689,-5.83242799455291));
#13113=CARTESIAN_POINT('Ctrl Pts',(-4.02836682984766,299.248925943689,-6.91182563342691));
#13114=CARTESIAN_POINT('Ctrl Pts',(-2.17634873314618,299.386425943689,-7.99122327230091));
#13115=CARTESIAN_POINT('Ctrl Pts',(-0.0327551936971984,299.523925943689,
-8.));
#13116=CARTESIAN_POINT('Ctrl Pts',(2.11083834575178,299.661425943689,-8.00877672769909));
#13117=CARTESIAN_POINT('Ctrl Pts',(3.97163317015235,299.798925943689,-6.94458082712411));
#13118=CARTESIAN_POINT('Ctrl Pts',(5.83242799455291,299.936425943689,-5.88038492654913));
#13119=CARTESIAN_POINT('Ctrl Pts',(6.91182563342691,300.073925943689,-4.02836682984766));
#13120=CARTESIAN_POINT('Ctrl Pts',(7.99122327230091,300.211425943689,-2.17634873314618));
#13121=CARTESIAN_POINT('Ctrl Pts',(8.,300.348925943689,-0.0327551936971989));
#13122=CARTESIAN_POINT('Ctrl Pts',(8.00877672769909,300.486425943689,2.11083834575178));
#13123=CARTESIAN_POINT('Ctrl Pts',(6.94458082712411,300.623925943689,3.97163317015235));
#13124=CARTESIAN_POINT('Ctrl Pts',(5.88038492654913,300.761425943689,5.83242799455291));
#13125=CARTESIAN_POINT('Ctrl Pts',(4.02836682984766,300.898925943689,6.91182563342691));
#13126=CARTESIAN_POINT('Ctrl Pts',(2.17634873314619,301.036425943689,7.99122327230091));
#13127=CARTESIAN_POINT('Ctrl Pts',(0.0327551936971994,301.173925943689,
8.));
#13128=CARTESIAN_POINT('Ctrl Pts',(-2.11083834575178,301.311425943689,8.00877672769909));
#13129=CARTESIAN_POINT('Ctrl Pts',(-3.97163317015234,301.448925943689,6.94458082712412));
#13130=CARTESIAN_POINT('Ctrl Pts',(-5.83242799455291,301.586425943689,5.88038492654913));
#13131=CARTESIAN_POINT('Ctrl Pts',(-6.91182563342691,301.723925943689,4.02836682984766));
#13132=CARTESIAN_POINT('Ctrl Pts',(-7.99122327230091,301.861425943689,2.17634873314619));
#13133=CARTESIAN_POINT('Ctrl Pts',(-8.,301.998925943689,0.0327551936971979));
#13134=CARTESIAN_POINT('Ctrl Pts',(-8.00877672769909,302.136425943689,-2.11083834575178));
#13135=CARTESIAN_POINT('Ctrl Pts',(-6.94458082712411,302.273925943689,-3.97163317015235));
#13136=CARTESIAN_POINT('Ctrl Pts',(-5.88038492654913,302.411425943689,-5.83242799455291));
#13137=CARTESIAN_POINT('Ctrl Pts',(-4.02836682984766,302.548925943689,-6.91182563342691));
#13138=CARTESIAN_POINT('Ctrl Pts',(-2.17634873314618,302.686425943689,-7.99122327230091));
#13139=CARTESIAN_POINT('Ctrl Pts',(-0.0327551936971984,302.823925943689,
-8.));
#13140=CARTESIAN_POINT('Ctrl Pts',(2.11083834575178,302.961425943689,-8.00877672769909));
#13141=CARTESIAN_POINT('Ctrl Pts',(3.97163317015235,303.098925943689,-6.94458082712411));
#13142=CARTESIAN_POINT('Ctrl Pts',(5.83242799455291,303.236425943689,-5.88038492654913));
#13143=CARTESIAN_POINT('Ctrl Pts',(6.91182563342691,303.373925943689,-4.02836682984766));
#13144=CARTESIAN_POINT('Ctrl Pts',(7.99122327230091,303.511425943689,-2.17634873314618));
#13145=CARTESIAN_POINT('Ctrl Pts',(8.,303.648925943689,-0.0327551936971989));
#13146=CARTESIAN_POINT('Ctrl Pts',(8.00877672769909,303.786425943689,2.11083834575178));
#13147=CARTESIAN_POINT('Ctrl Pts',(6.94458082712411,303.923925943689,3.97163317015235));
#13148=CARTESIAN_POINT('Ctrl Pts',(5.88038492654913,304.061425943689,5.83242799455291));
#13149=CARTESIAN_POINT('Ctrl Pts',(4.02836682984766,304.198925943689,6.91182563342691));
#13150=CARTESIAN_POINT('Ctrl Pts',(2.17634873314619,304.336425943689,7.99122327230091));
#13151=CARTESIAN_POINT('Ctrl Pts',(0.0327551936971994,304.473925943689,
8.));
#13152=CARTESIAN_POINT('Ctrl Pts',(-2.11083834575178,304.611425943689,8.00877672769909));
#13153=CARTESIAN_POINT('Ctrl Pts',(-3.97163317015234,304.748925943689,6.94458082712412));
#13154=CARTESIAN_POINT('Ctrl Pts',(-5.83242799455291,304.886425943689,5.88038492654913));
#13155=CARTESIAN_POINT('Ctrl Pts',(-6.91182563342691,305.023925943689,4.02836682984766));
#13156=CARTESIAN_POINT('Ctrl Pts',(-7.99122327230091,305.161425943689,2.17634873314619));
#13157=CARTESIAN_POINT('Ctrl Pts',(-8.,305.298925943689,0.0327551936971979));
#13158=CARTESIAN_POINT('Ctrl Pts',(-8.00877672769909,305.436425943689,-2.11083834575178));
#13159=CARTESIAN_POINT('Ctrl Pts',(-6.94458082712411,305.573925943689,-3.97163317015235));
#13160=CARTESIAN_POINT('Ctrl Pts',(-5.88038492654913,305.711425943689,-5.83242799455291));
#13161=CARTESIAN_POINT('Ctrl Pts',(-4.02836682984766,305.848925943689,-6.91182563342691));
#13162=CARTESIAN_POINT('Ctrl Pts',(-2.17634873314618,305.986425943689,-7.99122327230091));
#13163=CARTESIAN_POINT('Ctrl Pts',(-0.0327551936971984,306.123925943689,
-8.));
#13164=CARTESIAN_POINT('Ctrl Pts',(2.11083834575178,306.261425943689,-8.00877672769909));
#13165=CARTESIAN_POINT('Ctrl Pts',(3.97163317015235,306.398925943689,-6.94458082712411));
#13166=CARTESIAN_POINT('Ctrl Pts',(5.83242799455291,306.536425943689,-5.88038492654913));
#13167=CARTESIAN_POINT('Ctrl Pts',(6.91182563342691,306.673925943689,-4.02836682984766));
#13168=CARTESIAN_POINT('Ctrl Pts',(7.99122327230091,306.811425943689,-2.17634873314618));
#13169=CARTESIAN_POINT('Ctrl Pts',(8.,306.948925943689,-0.0327551936971989));
#13170=CARTESIAN_POINT('Ctrl Pts',(8.00877672769909,307.086425943689,2.11083834575178));
#13171=CARTESIAN_POINT('Ctrl Pts',(6.94458082712411,307.223925943689,3.97163317015235));
#13172=CARTESIAN_POINT('Ctrl Pts',(5.88038492654913,307.361425943689,5.83242799455291));
#13173=CARTESIAN_POINT('Ctrl Pts',(4.02836682984766,307.498925943689,6.91182563342691));
#13174=CARTESIAN_POINT('Ctrl Pts',(2.17634873314619,307.636425943689,7.99122327230091));
#13175=CARTESIAN_POINT('Ctrl Pts',(0.0327551936971994,307.773925943689,
8.));
#13176=CARTESIAN_POINT('Ctrl Pts',(-2.11083834575178,307.911425943689,8.00877672769909));
#13177=CARTESIAN_POINT('Ctrl Pts',(-3.97163317015234,308.048925943689,6.94458082712412));
#13178=CARTESIAN_POINT('Ctrl Pts',(-5.83242799455291,308.186425943689,5.88038492654913));
#13179=CARTESIAN_POINT('Ctrl Pts',(-6.91182563342691,308.323925943689,4.02836682984766));
#13180=CARTESIAN_POINT('Ctrl Pts',(-7.99122327230091,308.461425943689,2.17634873314619));
#13181=CARTESIAN_POINT('Ctrl Pts',(-8.,308.598925943689,0.0327551936971979));
#13182=CARTESIAN_POINT('Ctrl Pts',(-8.00877672769909,308.736425943689,-2.11083834575178));
#13183=CARTESIAN_POINT('Ctrl Pts',(-6.94458082712411,308.873925943689,-3.97163317015235));
#13184=CARTESIAN_POINT('Ctrl Pts',(-5.88038492654913,309.011425943689,-5.83242799455291));
#13185=CARTESIAN_POINT('Ctrl Pts',(-4.02836682984766,309.148925943689,-6.91182563342691));
#13186=CARTESIAN_POINT('Ctrl Pts',(-2.17634873314618,309.286425943689,-7.99122327230091));
#13187=CARTESIAN_POINT('Ctrl Pts',(-0.0327551936971984,309.423925943689,
-8.));
#13188=CARTESIAN_POINT('Ctrl Pts',(2.11083834575178,309.561425943689,-8.00877672769909));
#13189=CARTESIAN_POINT('Ctrl Pts',(3.97163317015235,309.698925943689,-6.94458082712411));
#13190=CARTESIAN_POINT('Ctrl Pts',(5.83242799455291,309.836425943689,-5.88038492654913));
#13191=CARTESIAN_POINT('Ctrl Pts',(6.91182563342691,309.973925943689,-4.02836682984766));
#13192=CARTESIAN_POINT('Ctrl Pts',(7.99122327230091,310.111425943689,-2.17634873314618));
#13193=CARTESIAN_POINT('Ctrl Pts',(8.,310.248925943689,-0.0327551936971989));
#13194=CARTESIAN_POINT('Ctrl Pts',(8.00877672769909,310.386425943689,2.11083834575178));
#13195=CARTESIAN_POINT('Ctrl Pts',(6.94458082712411,310.523925943689,3.97163317015235));
#13196=CARTESIAN_POINT('Ctrl Pts',(5.88038492654913,310.661425943689,5.83242799455291));
#13197=CARTESIAN_POINT('Ctrl Pts',(4.02836682984766,310.798925943689,6.91182563342691));
#13198=CARTESIAN_POINT('Ctrl Pts',(2.17634873314619,310.936425943689,7.99122327230091));
#13199=CARTESIAN_POINT('Ctrl Pts',(0.0327551936971994,311.073925943689,
8.));
#13200=CARTESIAN_POINT('Ctrl Pts',(-2.11083834575178,311.211425943689,8.00877672769909));
#13201=CARTESIAN_POINT('Ctrl Pts',(-3.97163317015234,311.348925943689,6.94458082712412));
#13202=CARTESIAN_POINT('Ctrl Pts',(-5.83242799455291,311.486425943689,5.88038492654913));
#13203=CARTESIAN_POINT('Ctrl Pts',(-6.91182563342691,311.623925943689,4.02836682984766));
#13204=CARTESIAN_POINT('Ctrl Pts',(-7.99122327230091,311.761425943689,2.17634873314619));
#13205=CARTESIAN_POINT('Ctrl Pts',(-8.,311.898925943689,0.0327551936971979));
#13206=CARTESIAN_POINT('Ctrl Pts',(-8.00877672769909,312.036425943689,-2.11083834575178));
#13207=CARTESIAN_POINT('Ctrl Pts',(-6.94458082712411,312.173925943689,-3.97163317015235));
#13208=CARTESIAN_POINT('Ctrl Pts',(-5.88038492654913,312.311425943689,-5.83242799455291));
#13209=CARTESIAN_POINT('Ctrl Pts',(-4.02836682984766,312.448925943689,-6.91182563342691));
#13210=CARTESIAN_POINT('Ctrl Pts',(-2.17634873314618,312.586425943689,-7.99122327230091));
#13211=CARTESIAN_POINT('Ctrl Pts',(-0.0327551936971984,312.723925943689,
-8.));
#13212=CARTESIAN_POINT('Ctrl Pts',(2.11083834575178,312.861425943689,-8.00877672769909));
#13213=CARTESIAN_POINT('Ctrl Pts',(3.97163317015235,312.998925943689,-6.94458082712411));
#13214=CARTESIAN_POINT('Ctrl Pts',(5.83242799455291,313.136425943689,-5.88038492654913));
#13215=CARTESIAN_POINT('Ctrl Pts',(6.91182563342691,313.273925943689,-4.02836682984766));
#13216=CARTESIAN_POINT('Ctrl Pts',(7.99122327230091,313.411425943689,-2.17634873314618));
#13217=CARTESIAN_POINT('Ctrl Pts',(8.,313.548925943689,-0.0327551936971989));
#13218=CARTESIAN_POINT('Ctrl Pts',(8.00877672769909,313.686425943689,2.11083834575178));
#13219=CARTESIAN_POINT('Ctrl Pts',(6.94458082712411,313.823925943689,3.97163317015235));
#13220=CARTESIAN_POINT('Ctrl Pts',(5.88038492654913,313.961425943689,5.83242799455291));
#13221=CARTESIAN_POINT('Ctrl Pts',(4.02836682984766,314.098925943689,6.91182563342691));
#13222=CARTESIAN_POINT('Ctrl Pts',(2.17634873314619,314.236425943689,7.99122327230091));
#13223=CARTESIAN_POINT('Ctrl Pts',(0.0327551936971994,314.373925943689,
8.));
#13224=CARTESIAN_POINT('Ctrl Pts',(-2.11083834575178,314.511425943689,8.00877672769909));
#13225=CARTESIAN_POINT('Ctrl Pts',(-3.97163317015234,314.648925943689,6.94458082712412));
#13226=CARTESIAN_POINT('Ctrl Pts',(-5.83242799455291,314.786425943689,5.88038492654913));
#13227=CARTESIAN_POINT('Ctrl Pts',(-6.91182563342691,314.923925943689,4.02836682984766));
#13228=CARTESIAN_POINT('Ctrl Pts',(-7.99122327230091,315.061425943689,2.17634873314619));
#13229=CARTESIAN_POINT('Ctrl Pts',(-8.,315.198925943689,0.0327551936971979));
#13230=CARTESIAN_POINT('Ctrl Pts',(-8.00877672769909,315.336425943689,-2.11083834575178));
#13231=CARTESIAN_POINT('Ctrl Pts',(-6.94458082712411,315.473925943689,-3.97163317015235));
#13232=CARTESIAN_POINT('Ctrl Pts',(-5.88038492654913,315.611425943689,-5.83242799455291));
#13233=CARTESIAN_POINT('Ctrl Pts',(-4.02836682984766,315.748925943689,-6.91182563342691));
#13234=CARTESIAN_POINT('Ctrl Pts',(-2.17634873314618,315.886425943689,-7.99122327230091));
#13235=CARTESIAN_POINT('Ctrl Pts',(-0.0327551936971984,316.023925943689,
-8.));
#13236=CARTESIAN_POINT('Ctrl Pts',(2.11083834575178,316.161425943689,-8.00877672769909));
#13237=CARTESIAN_POINT('Ctrl Pts',(3.97163317015235,316.298925943689,-6.94458082712411));
#13238=CARTESIAN_POINT('Ctrl Pts',(5.83242799455291,316.436425943689,-5.88038492654913));
#13239=CARTESIAN_POINT('Ctrl Pts',(6.91182563342691,316.573925943689,-4.02836682984766));
#13240=CARTESIAN_POINT('Ctrl Pts',(7.99122327230091,316.711425943689,-2.17634873314618));
#13241=CARTESIAN_POINT('Ctrl Pts',(8.,316.848925943689,-0.0327551936971989));
#13242=CARTESIAN_POINT('Ctrl Pts',(8.00877672769909,316.986425943689,2.11083834575178));
#13243=CARTESIAN_POINT('Ctrl Pts',(6.94458082712411,317.123925943689,3.97163317015235));
#13244=CARTESIAN_POINT('Ctrl Pts',(5.88038492654913,317.261425943689,5.83242799455291));
#13245=CARTESIAN_POINT('Ctrl Pts',(4.02836682984766,317.398925943689,6.91182563342691));
#13246=CARTESIAN_POINT('Ctrl Pts',(2.17634873314619,317.536425943689,7.99122327230091));
#13247=CARTESIAN_POINT('Ctrl Pts',(0.0327551936971994,317.673925943689,
8.));
#13248=CARTESIAN_POINT('Ctrl Pts',(-2.11083834575178,317.811425943689,8.00877672769909));
#13249=CARTESIAN_POINT('Ctrl Pts',(-3.97163317015234,317.948925943689,6.94458082712412));
#13250=CARTESIAN_POINT('Ctrl Pts',(-5.83242799455291,318.086425943689,5.88038492654913));
#13251=CARTESIAN_POINT('Ctrl Pts',(-6.91182563342691,318.223925943689,4.02836682984766));
#13252=CARTESIAN_POINT('Ctrl Pts',(-7.99122327230091,318.361425943689,2.17634873314619));
#13253=CARTESIAN_POINT('Ctrl Pts',(-8.,318.498925943689,0.0327551936971979));
#13254=CARTESIAN_POINT('Ctrl Pts',(-4.63461213585364,285.,-6.52084682023068));
#13255=CARTESIAN_POINT('Ctrl Pts',(-4.63617687809023,285.,-6.52302941473603));
#13256=CARTESIAN_POINT('Ctrl Pts',(-4.63798167723247,285.,-6.52498169175354));
#13257=CARTESIAN_POINT('Ctrl Pts',(-4.64219825050599,285.,-6.52861106616703));
#13258=CARTESIAN_POINT('Ctrl Pts',(-4.64459104103043,285.,-6.53021023836018));
#13259=CARTESIAN_POINT('Ctrl Pts',(-4.65315442170252,285.,-6.53481267652416));
#13260=CARTESIAN_POINT('Ctrl Pts',(-4.6600128556107,285.,-6.53672564774018));
#13261=CARTESIAN_POINT('Ctrl Pts',(-4.68576001867322,285.,-6.54097523595292));
#13262=CARTESIAN_POINT('Ctrl Pts',(-4.70898798502752,285.,-6.53862241186785));
#13263=CARTESIAN_POINT('Ctrl Pts',(-4.78979719606241,285.,-6.52397532465739));
#13264=CARTESIAN_POINT('Ctrl Pts',(-4.87291591474625,285.,-6.49381972833199));
#13265=CARTESIAN_POINT('Ctrl Pts',(-5.22082506112394,285.,-6.32959551460495));
#13266=CARTESIAN_POINT('Ctrl Pts',(-5.60001341231252,285.,-6.09157840023));
#13267=CARTESIAN_POINT('Ctrl Pts',(-6.53370549418297,285.,-5.26074061589865));
#13268=CARTESIAN_POINT('Ctrl Pts',(-7.06063989282633,285.000000000001,-4.64167227552575));
#13269=CARTESIAN_POINT('Ctrl Pts',(-7.81016526044142,285.000000000001,-3.30202932947539));
#13270=CARTESIAN_POINT('Ctrl Pts',(-8.05076497001306,284.999999999935,-2.7124664396346));
#13271=CARTESIAN_POINT('Ctrl Pts',(-8.40561382232048,284.999999999935,-1.41649823255915));
#13272=CARTESIAN_POINT('Ctrl Pts',(-8.5,285.,-0.709762093140782));
#13273=CARTESIAN_POINT('Ctrl Pts',(-8.5,285.,8.11850586757146E-14));
#13274=CARTESIAN_POINT('Origin',(-8.,318.,8.32667268468867E-14));
#13275=CARTESIAN_POINT('Origin',(-8.,317.501074056311,-0.0327551936970314));
#13276=CARTESIAN_POINT('Origin',(0.,285.,0.));
#14070=UNCERTAINTY_MEASURE_WITH_UNIT(LENGTH_MEASURE(0.01),#14085,
'DISTANCE_ACCURACY_VALUE',
'Maximum model space distance between geometric entities at asserted c
onnectivities');
#14073=UNCERTAINTY_MEASURE_WITH_UNIT(LENGTH_MEASURE(0.01),#14085,
'DISTANCE_ACCURACY_VALUE',
'Maximum model space distance between geometric entities at asserted c
onnectivities');
#14081=(
GEOMETRIC_REPRESENTATION_CONTEXT(3)
GLOBAL_UNCERTAINTY_ASSIGNED_CONTEXT((#14070))
GLOBAL_UNIT_ASSIGNED_CONTEXT((#14085,#14087,#14088))
REPRESENTATION_CONTEXT('','3D')
);
#14084=(
GEOMETRIC_REPRESENTATION_CONTEXT(3)
GLOBAL_UNCERTAINTY_ASSIGNED_CONTEXT((#14073))
GLOBAL_UNIT_ASSIGNED_CONTEXT((#14085,#14087,#14088))
REPRESENTATION_CONTEXT('','3D')
);
#14085=(
LENGTH_UNIT()
NAMED_UNIT(*)
SI_UNIT(.MILLI.,.METRE.)
);
#14087=(
NAMED_UNIT(*)
PLANE_ANGLE_UNIT()
SI_UNIT($,.RADIAN.)
);
#14088=(
NAMED_UNIT(*)
SI_UNIT($,.STERADIAN.)
SOLID_ANGLE_UNIT()
);
#14096=SHAPE_DEFINITION_REPRESENTATION(#14106,#14126);
#14106=PRODUCT_DEFINITION_SHAPE('',$,#14137);
#14126=SHAPE_REPRESENTATION('',(#3794),#14081);
#14129=PRODUCT_DEFINITION_CONTEXT('part definition',#14161,'design');
#14137=PRODUCT_DEFINITION('spring','spring',#14147,#14129);
#14147=PRODUCT_DEFINITION_FORMATION('',$,#14170);
#14161=APPLICATION_CONTEXT(
'Core Data for Automotive Mechanical Design Process');
#14162=PRODUCT_CONTEXT('part definition',#14161,'mechanical');
#14170=PRODUCT('spring','spring',$,(#14162));
#14176=PRESENTATION_STYLE_ASSIGNMENT((#14182));
#14182=SURFACE_STYLE_USAGE(.BOTH.,#14188);
#14188=SURFACE_SIDE_STYLE('',(#14194));
#14194=SURFACE_STYLE_FILL_AREA(#14200);
#14200=FILL_AREA_STYLE('Opaque(122,133,145)',(#14206));
#14206=FILL_AREA_STYLE_COLOUR('Opaque(122,133,145)',#14212);
#14212=COLOUR_RGB('Opaque(122,133,145)',0.47843137254902,0.52156862745098,
0.568627450980392);
ENDSEC;
END-ISO-10303-21;
